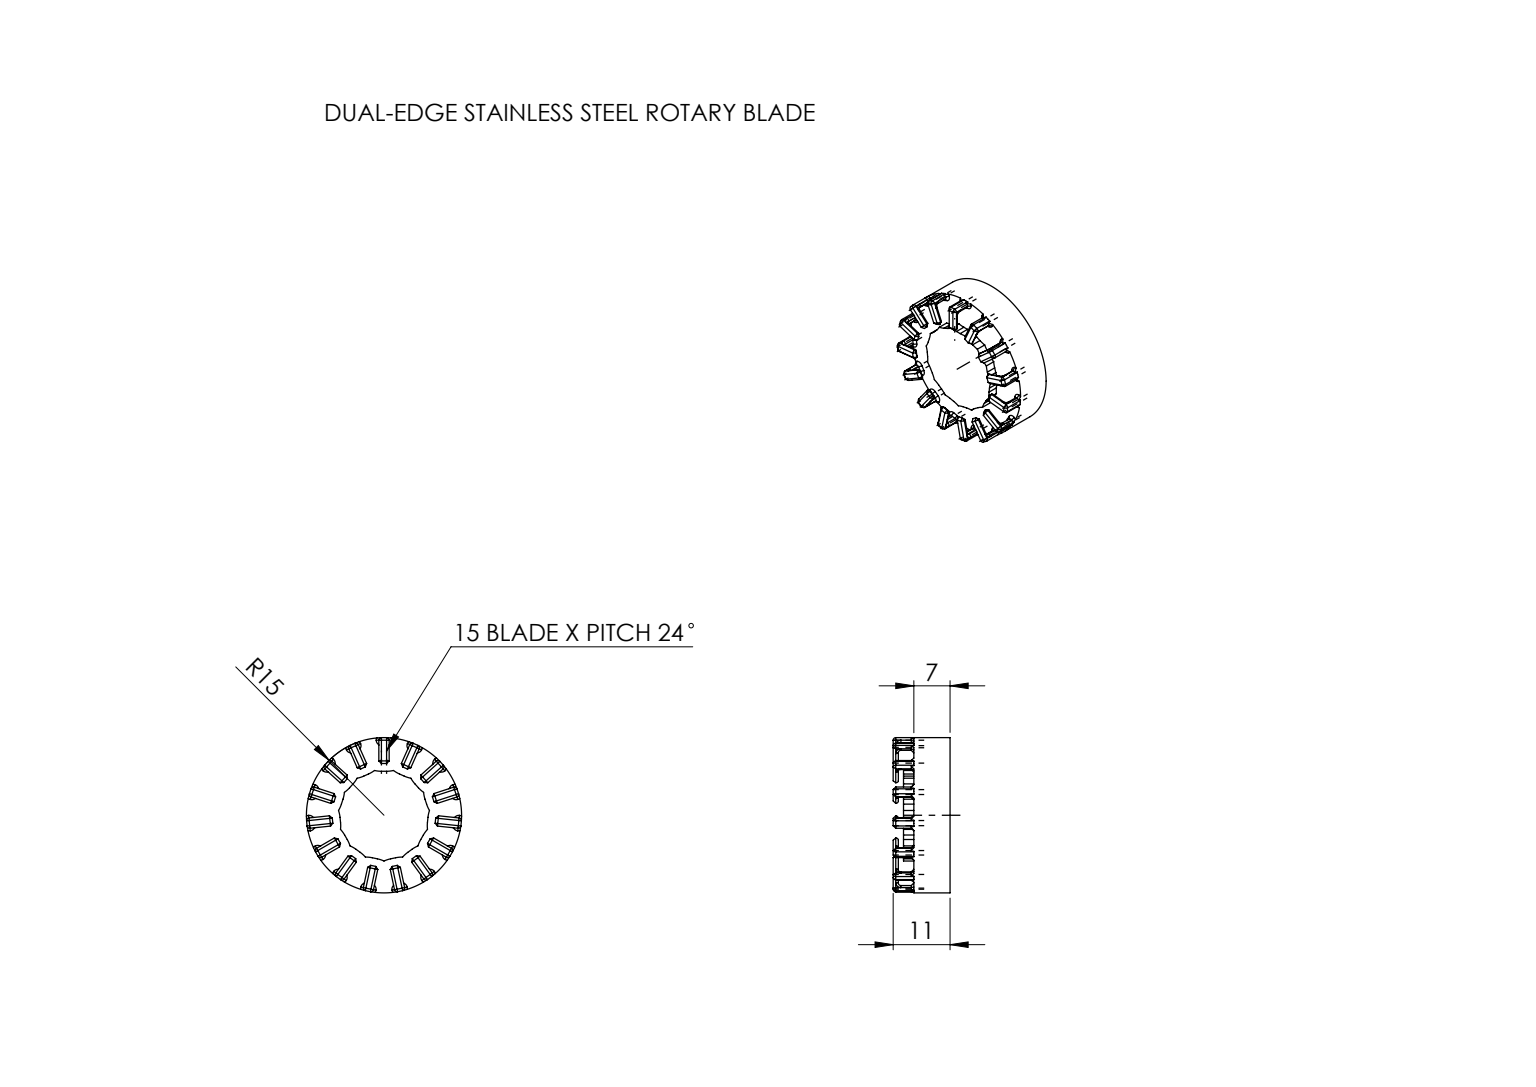
ISO-10303-21;
HEADER;
FILE_DESCRIPTION (('STEP AP214'),
    '1' );
FILE_NAME ('Dual-Edge Stainless Steel Rotary Blade.step',
    '2026-10-04T08:29:30',
    ( '' ),
    ( '' ),
    'SwSTEP 2.0',
    'SolidWorks 2026',
    '' );
FILE_SCHEMA (( 'AUTOMOTIVE_DESIGN' ));
ENDSEC;

DATA;
#1=DIRECTION ( 'NONE',  ( 1.000000000000000000, 0.000000000000000000, 0.000000000000000000 ) ) ;
#2=ORIENTED_EDGE ( 'NONE', *, *, #18761, .T. ) ;
#6=DIRECTION ( 'NONE',  ( 1.000000000000000000, 0.000000000000000000, 0.000000000000000000 ) ) ;
#11=ORIENTED_EDGE ( 'NONE', *, *, #12384, .T. ) ;
#13=DIRECTION ( 'NONE',  ( -0.2185080122244334455, 0.6724985119639524944, -0.7071067811865451302 ) ) ;
#14=ORIENTED_EDGE ( 'NONE', *, *, #11344, .T. ) ;
#16=ORIENTED_EDGE ( 'NONE', *, *, #14456, .T. ) ;
#21=CARTESIAN_POINT ( 'NONE',  ( -7.470035553104361625, 44.81454624109330354, 7.499999999999994671 ) ) ;
#23=DIRECTION ( 'NONE',  ( 0.8660254037844363761, -0.5000000000000038858, 0.000000000000000000 ) ) ;
#24=CARTESIAN_POINT ( 'NONE',  ( 0.000000000000000000, 22.50000000000000355, 7.000000000000000000 ) ) ;
#25=DIRECTION ( 'NONE',  ( 0.9510565162951544194, 0.3090169943749449533, -0.000000000000000000 ) ) ;
#26=AXIS2_PLACEMENT_3D ( 'NONE', #30413, #27350, #24305 ) ;
#29=CARTESIAN_POINT ( 'NONE',  ( 11.44473057578109199, 31.45924896672603310, 11.00000000000000000 ) ) ;
#32=PLANE ( 'NONE',  #24163 ) ;
#36=AXIS2_PLACEMENT_3D ( 'NONE', #271, #15908, #35000 ) ;
#42=VERTEX_POINT ( 'NONE', #38948 ) ;
#46=EDGE_LOOP ( 'NONE', ( #16862, #39215, #35738, #30448, #9840 ) ) ;
#50=DIRECTION ( 'NONE',  ( 0.000000000000000000, 0.000000000000000000, 1.000000000000000000 ) ) ;
#51=ORIENTED_EDGE ( 'NONE', *, *, #33215, .T. ) ;
#53=DIRECTION ( 'NONE',  ( 0.000000000000000000, 0.000000000000000000, 1.000000000000000000 ) ) ;
#55=VECTOR ( 'NONE', #14215, 1000.000000000000114 ) ;
#56=ORIENTED_EDGE ( 'NONE', *, *, #7043, .F. ) ;
#58=EDGE_LOOP ( 'NONE', ( #5255, #36161, #10685, #33701, #20952, #26926 ) ) ;
#62=ADVANCED_FACE ( 'NONE', ( #11719 ), #11120, .F. ) ;
#65=B_SPLINE_CURVE_WITH_KNOTS ( 'NONE', 3,
 ( #33912, #15414, #12759, #24753 ),
 .UNSPECIFIED., .F., .F.,
 ( 4, 4 ),
 ( 0.000000000000000000, 1.000000000000000000 ),
 .UNSPECIFIED. ) ;
#66=DIRECTION ( 'NONE',  ( -0.7431448254773862505, 0.6691306063588670083, 0.000000000000000000 ) ) ;
#68=AXIS2_PLACEMENT_3D ( 'NONE', #9965, #18910, #3865 ) ;
#69=CARTESIAN_POINT ( 'NONE',  ( 13.16028273094469192, 27.30176617939681449, 7.500000000000000000 ) ) ;
#71=AXIS2_PLACEMENT_3D ( 'NONE', #37438, #19346, #24844 ) ;
#72=DIRECTION ( 'NONE',  ( 1.000000000000000000, 0.000000000000000000, 0.000000000000000000 ) ) ;
#77=LINE ( 'NONE', #28854, #39100 ) ;
#80=AXIS2_PLACEMENT_3D ( 'NONE', #8723, #5868, #21115 ) ;
#86=EDGE_CURVE ( 'NONE', #10650, #36352, #5018, .T. ) ;
#87=EDGE_CURVE ( 'NONE', #32024, #8691, #8265, .T. ) ;
#88=FACE_OUTER_BOUND ( 'NONE', #25891, .T. ) ;
#92=EDGE_LOOP ( 'NONE', ( #13644, #34417, #27683, #7485 ) ) ;
#96=CARTESIAN_POINT ( 'NONE',  ( -10.06946225350398194, 32.23940090176283491, 9.500000000000000000 ) ) ;
#97=VECTOR ( 'NONE', #32100, 1000.000000000000000 ) ;
#101=CARTESIAN_POINT ( 'NONE',  ( -14.97283176289963968, 21.60377111278828011, 10.49999999999999645 ) ) ;
#103=ORIENTED_EDGE ( 'NONE', *, *, #28678, .T. ) ;
#106=LINE ( 'NONE', #9845, #39374 ) ;
#108=ORIENTED_EDGE ( 'NONE', *, *, #38694, .T. ) ;
#111=DIRECTION ( 'NONE',  ( 0.000000000000000000, 0.000000000000000000, 1.000000000000000000 ) ) ;
#113=VERTEX_POINT ( 'NONE', #23905 ) ;
#114=VECTOR ( 'NONE', #22519, 1000.000000000000000 ) ;
#117=DIRECTION ( 'NONE',  ( 0.1045284632676436315, -0.9945218953682742891, 0.000000000000000000 ) ) ;
#118=ORIENTED_EDGE ( 'NONE', *, *, #842, .F. ) ;
#119=CARTESIAN_POINT ( 'NONE',  ( 14.09933648065468503, 26.02968990214154843, 7.500000000000000888 ) ) ;
#121=DIRECTION ( 'NONE',  ( 0.5446390350150238646, -0.8386705679454261597, 0.000000000000000000 ) ) ;
#124=DIRECTION ( 'NONE',  ( 1.000000000000000000, 3.469446951953568829E-15, 0.000000000000000000 ) ) ;
#125=FACE_OUTER_BOUND ( 'NONE', #14098, .T. ) ;
#126=LINE ( 'NONE', #12516, #37440 ) ;
#127=CARTESIAN_POINT ( 'NONE',  ( 11.77212950435618488, 31.79629403205455063, 7.338691926023207301 ) ) ;
#129=CYLINDRICAL_SURFACE ( 'NONE', #3554, 0.5000000000000004441 ) ;
#130=ORIENTED_EDGE ( 'NONE', *, *, #22039, .F. ) ;
#132=FACE_OUTER_BOUND ( 'NONE', #27069, .T. ) ;
#134=AXIS2_PLACEMENT_3D ( 'NONE', #36095, #30198, #27342 ) ;
#136=ADVANCED_FACE ( 'NONE', ( #30004 ), #2180, .T. ) ;
#139=B_SPLINE_CURVE_WITH_KNOTS ( 'NONE', 3,
 ( #14310, #17577, #20620, #36259, #23258, #23855, #38896, #35449 ),
 .UNSPECIFIED., .F., .F.,
 ( 4, 2, 2, 4 ),
 ( 0.000000000000000000, 0.0004726692273637091287, 0.0007090038410455639642, 0.0009453384547274186912 ),
 .UNSPECIFIED. ) ;
#141=ORIENTED_EDGE ( 'NONE', *, *, #26869, .T. ) ;
#142=FACE_OUTER_BOUND ( 'NONE', #24319, .T. ) ;
#150=CARTESIAN_POINT ( 'NONE',  ( -8.927394655428429360, 11.06314620770957013, 11.00000000000000000 ) ) ;
#151=ORIENTED_EDGE ( 'NONE', *, *, #23785, .T. ) ;
#155=ORIENTED_EDGE ( 'NONE', *, *, #21487, .F. ) ;
#156=CYLINDRICAL_SURFACE ( 'NONE', #5742, 0.5000000000000004441 ) ;
#157=DIRECTION ( 'NONE',  ( -0.1045284632676566766, -0.9945218953682730678, 0.000000000000000000 ) ) ;
#159=EDGE_CURVE ( 'NONE', #19442, #37263, #30806, .T. ) ;
#162=EDGE_CURVE ( 'NONE', #21531, #36577, #11917, .T. ) ;
#163=VERTEX_POINT ( 'NONE', #30609 ) ;
#165=CARTESIAN_POINT ( 'NONE',  ( 6.654030453887980201, 35.94335816374507431, 7.500000000000000888 ) ) ;
#166=ORIENTED_EDGE ( 'NONE', *, *, #36174, .F. ) ;
#167=DIRECTION ( 'NONE',  ( -1.000000000000000000, 0.000000000000000000, 0.000000000000000000 ) ) ;
#170=VECTOR ( 'NONE', #21979, 1000.000000000000000 ) ;
#171=CARTESIAN_POINT ( 'NONE',  ( 0.000000000000000000, 22.50000000000000355, 7.000000000000000000 ) ) ;
#172=VERTEX_POINT ( 'NONE', #15755 ) ;
#174=DIRECTION ( 'NONE',  ( 0.000000000000000000, 0.000000000000000000, -1.000000000000000000 ) ) ;
#177=DIRECTION ( 'NONE',  ( 0.000000000000000000, 0.000000000000000000, -1.000000000000000000 ) ) ;
#178=CARTESIAN_POINT ( 'NONE',  ( 14.47283171447379146, 21.48159823030311344, 7.500000000000010658 ) ) ;
#180=ORIENTED_EDGE ( 'NONE', *, *, #19438, .T. ) ;
#184=LINE ( 'NONE', #27415, #10010 ) ;
#188=LINE ( 'NONE', #25168, #20681 ) ;
#189=EDGE_CURVE ( 'NONE', #7975, #16887, #8966, .T. ) ;
#190=AXIS2_PLACEMENT_3D ( 'NONE', #26813, #7919, #22957 ) ;
#197=CARTESIAN_POINT ( 'NONE',  ( -9.677076426724102731, 26.69573495723219736, 10.50000000000000000 ) ) ;
#198=ORIENTED_EDGE ( 'NONE', *, *, #35032, .T. ) ;
#201=CARTESIAN_POINT ( 'NONE',  ( -8.306370210276497801, 9.993911548625852959, 10.49999999999999822 ) ) ;
#202=LINE ( 'NONE', #23984, #35140 ) ;
#203=ORIENTED_EDGE ( 'NONE', *, *, #26918, .F. ) ;
#207=ORIENTED_EDGE ( 'NONE', *, *, #30268, .T. ) ;
#209=DIRECTION ( 'NONE',  ( 0.6123724356958052395, 0.3535533905932595200, -0.7071067811865454633 ) ) ;
#210=EDGE_CURVE ( 'NONE', #22927, #29202, #39935, .T. ) ;
#211=VECTOR ( 'NONE', #28552, 1000.000000000000000 ) ;
#215=EDGE_CURVE ( 'NONE', #19575, #30083, #1517, .T. ) ;
#216=EDGE_LOOP ( 'NONE', ( #4536, #16133, #31309, #14302 ) ) ;
#218=PLANE ( 'NONE',  #11258 ) ;
#219=AXIS2_PLACEMENT_3D ( 'NONE', #21595, #14504, #26896 ) ;
#220=CARTESIAN_POINT ( 'NONE',  ( 2.629601561899395534, 7.723830143584016206, 10.49999999999999822 ) ) ;
#222=STYLED_ITEM ( 'NONE', ( #29995 ), #8155 ) ;
#224=CARTESIAN_POINT ( 'NONE',  ( 5.288651019504051476, 36.01756689786824239, 10.83333333333333393 ) ) ;
#225=ORIENTED_EDGE ( 'NONE', *, *, #29984, .F. ) ;
#226=FACE_OUTER_BOUND ( 'NONE', #33759, .T. ) ;
#229=FACE_OUTER_BOUND ( 'NONE', #25110, .T. ) ;
#232=AXIS2_PLACEMENT_3D ( 'NONE', #21106, #26799, #8514 ) ;
#234=DIRECTION ( 'NONE',  ( -0.000000000000000000, -0.000000000000000000, -1.000000000000000000 ) ) ;
#236=EDGE_CURVE ( 'NONE', #29069, #1872, #12116, .T. ) ;
#239=CIRCLE ( 'NONE', #18429, 0.5000000000000004441 ) ;
#248=CIRCLE ( 'NONE', #15817, 0.5000000000000004441 ) ;
#249=ORIENTED_EDGE ( 'NONE', *, *, #12112, .F. ) ;
#252=DIRECTION ( 'NONE',  ( 0.9781476007338072431, 0.2079116908177519041, 0.000000000000000000 ) ) ;
#253=VERTEX_POINT ( 'NONE', #30414 ) ;
#257=VERTEX_POINT ( 'NONE', #18219 ) ;
#259=ORIENTED_EDGE ( 'NONE', *, *, #8002, .F. ) ;
#265=ORIENTED_EDGE ( 'NONE', *, *, #11360, .F. ) ;
#267=DIRECTION ( 'NONE',  ( 0.7431448254773953543, 0.6691306063588571273, 0.000000000000000000 ) ) ;
#271=CARTESIAN_POINT ( 'NONE',  ( -8.118377661053489902, 10.47536095541709322, 9.000000000000001776 ) ) ;
#272=PRODUCT_DEFINITION_SHAPE ( 'NONE', 'NONE',  #1580 ) ;
#277=CARTESIAN_POINT ( 'NONE',  ( 8.137585970692082782, 29.15429895402929361, 11.00000000000000000 ) ) ;
#280=CARTESIAN_POINT ( 'NONE',  ( -9.356056665764020508, 26.06569820189716324, 10.50000000000000533 ) ) ;
#283=AXIS2_PLACEMENT_3D ( 'NONE', #15158, #26953, #5218 ) ;
#287=LINE ( 'NONE', #25064, #8816 ) ;
#289=EDGE_LOOP ( 'NONE', ( #19488, #26739, #33941, #35393 ) ) ;
#290=EDGE_CURVE ( 'NONE', #7488, #10226, #26444, .T. ) ;
#291=DIRECTION ( 'NONE',  ( 0.9781476007338042455, -0.2079116908177663647, 0.000000000000000000 ) ) ;
#294=LINE ( 'NONE', #21426, #16002 ) ;
#297=ORIENTED_EDGE ( 'NONE', *, *, #12319, .F. ) ;
#300=PLANE ( 'NONE',  #32607 ) ;
#302=ORIENTED_EDGE ( 'NONE', *, *, #4167, .F. ) ;
#306=EDGE_CURVE ( 'NONE', #11401, #17187, #24700, .T. ) ;
#307=DIRECTION ( 'NONE',  ( 0.000000000000000000, 0.000000000000000000, -1.000000000000000000 ) ) ;
#310=VECTOR ( 'NONE', #30674, 1000.000000000000114 ) ;
#316=LINE ( 'NONE', #21645, #40068 ) ;
#320=CARTESIAN_POINT ( 'NONE',  ( -13.48130249190472796, 27.93180293473203690, 10.50000000000000533 ) ) ;
#324=DIRECTION ( 'NONE',  ( -0.000000000000000000, -0.000000000000000000, -1.000000000000000000 ) ) ;
#326=DIRECTION ( 'NONE',  ( -0.2079116908177664480, -0.9781476007338042455, 0.000000000000000000 ) ) ;
#328=CARTESIAN_POINT ( 'NONE',  ( 12.80736835487433289, 15.68301270189216545, 9.000000000000001776 ) ) ;
#332=DIRECTION ( 'NONE',  ( -0.2079116908177667256, -0.9781476007338041345, 1.734723475976808475E-15 ) ) ;
#335=CARTESIAN_POINT ( 'NONE',  ( 8.593266739736579396, 16.38397459621552699, 11.00000000000000000 ) ) ;
#336=DIRECTION ( 'NONE',  ( -0.000000000000000000, -0.000000000000000000, 1.000000000000000000 ) ) ;
#343=VECTOR ( 'NONE', #22858, 1000.000000000000000 ) ;
#347=VECTOR ( 'NONE', #26561, 1000.000000000000000 ) ;
#352=EDGE_CURVE ( 'NONE', #2306, #34064, #29151, .T. ) ;
#354=CARTESIAN_POINT ( 'NONE',  ( -10.44103466624267185, 32.57396620494226624, 7.000000000000000000 ) ) ;
#359=ORIENTED_EDGE ( 'NONE', *, *, #3116, .F. ) ;
#360=LINE ( 'NONE', #21297, #8908 ) ;
#361=DIRECTION ( 'NONE',  ( -0.9781476007338043566, 0.2079116908177657264, 0.000000000000000000 ) ) ;
#365=B_SPLINE_CURVE_WITH_KNOTS ( 'NONE', 3,
 ( #13662, #35008, #16115, #477 ),
 .UNSPECIFIED., .F., .F.,
 ( 4, 4 ),
 ( 0.0008976806579034594512, 0.0009453384547274206427 ),
 .UNSPECIFIED. ) ;
#366=EDGE_LOOP ( 'NONE', ( #29228, #30799, #2804, #38071 ) ) ;
#367=EDGE_CURVE ( 'NONE', #32326, #14728, #6690, .T. ) ;
#368=DIRECTION ( 'NONE',  ( -0.000000000000000000, -0.000000000000000000, 1.000000000000000000 ) ) ;
#371=DIRECTION ( 'NONE',  ( 0.4156269377774552409, 0.5720614028176769228, 0.7071067811865524577 ) ) ;
#374=AXIS2_PLACEMENT_3D ( 'NONE', #5565, #29757, #14717 ) ;
#375=AXIS2_PLACEMENT_3D ( 'NONE', #24776, #21926, #21529 ) ;
#377=EDGE_LOOP ( 'NONE', ( #16222, #29568, #22970, #4101 ) ) ;
#379=CARTESIAN_POINT ( 'NONE',  ( -9.337241587065845394, 10.76617146908760247, 10.49999999999999822 ) ) ;
#380=CARTESIAN_POINT ( 'NONE',  ( -9.625795778762141097, 10.95253033666833709, 10.50000000000000533 ) ) ;
#381=DIRECTION ( 'NONE',  ( -0.000000000000000000, -0.000000000000000000, -1.000000000000000000 ) ) ;
#383=DIRECTION ( 'NONE',  ( 0.000000000000000000, 0.000000000000000000, 1.000000000000000000 ) ) ;
#385=EDGE_LOOP ( 'NONE', ( #29056, #12887, #37064, #5355 ) ) ;
#392=ADVANCED_FACE ( 'NONE', ( #10459 ), #7403, .F. ) ;
#393=FACE_OUTER_BOUND ( 'NONE', #10195, .T. ) ;
#398=CARTESIAN_POINT ( 'NONE',  ( 14.08246327825360389, 27.69965426814068366, 10.49999999999999822 ) ) ;
#400=VERTEX_POINT ( 'NONE', #31792 ) ;
#402=AXIS2_PLACEMENT_3D ( 'NONE', #36373, #21524, #8537 ) ;
#408=ORIENTED_EDGE ( 'NONE', *, *, #8409, .F. ) ;
#410=CARTESIAN_POINT ( 'NONE',  ( -13.13581098909220302, 27.45627467658446008, 11.00000000000000000 ) ) ;
#413=ORIENTED_EDGE ( 'NONE', *, *, #8934, .F. ) ;
#416=ORIENTED_EDGE ( 'NONE', *, *, #27931, .F. ) ;
#425=ORIENTED_EDGE ( 'NONE', *, *, #25457, .F. ) ;
#429=DIRECTION ( 'NONE',  ( -0.8090169943749504489, -0.5877852522924690293, 0.000000000000000000 ) ) ;
#437=EDGE_CURVE ( 'NONE', #21611, #37532, #717, .T. ) ;
#438=ORIENTED_EDGE ( 'NONE', *, *, #8735, .T. ) ;
#442=EDGE_CURVE ( 'NONE', #4338, #959, #22639, .T. ) ;
#444=EDGE_LOOP ( 'NONE', ( #34440, #26778, #20838, #31828 ) ) ;
#445=VERTEX_POINT ( 'NONE', #22048 ) ;
#449=ORIENTED_EDGE ( 'NONE', *, *, #1153, .F. ) ;
#450=EDGE_CURVE ( 'NONE', #13434, #36251, #32021, .T. ) ;
#454=ORIENTED_EDGE ( 'NONE', *, *, #7492, .F. ) ;
#456=LINE ( 'NONE', #12243, #18704 ) ;
#457=DIRECTION ( 'NONE',  ( 0.000000000000000000, 0.000000000000000000, 1.000000000000000000 ) ) ;
#458=EDGE_LOOP ( 'NONE', ( #11462, #15497, #1605 ) ) ;
#462=AXIS2_PLACEMENT_3D ( 'NONE', #19631, #7640, #26540 ) ;
#465=ORIENTED_EDGE ( 'NONE', *, *, #21335, .F. ) ;
#467=CARTESIAN_POINT ( 'NONE',  ( -14.63635198741550347, 25.78286467897752487, 7.000000000000000000 ) ) ;
#470=VECTOR ( 'NONE', #7205, 1000.000000000000000 ) ;
#471=LINE ( 'NONE', #3906, #36294 ) ;
#474=DIRECTION ( 'NONE',  ( 1.000000000000000000, 0.000000000000000000, 0.000000000000000000 ) ) ;
#477=CARTESIAN_POINT ( 'NONE',  ( -14.44277748876676881, 26.55045409923033972, 7.499999999999993783 ) ) ;
#480=VECTOR ( 'NONE', #651, 1000.000000000000114 ) ;
#481=VERTEX_POINT ( 'NONE', #34449 ) ;
#483=AXIS2_PLACEMENT_3D ( 'NONE', #20290, #35930, #32279 ) ;
#486=CARTESIAN_POINT ( 'NONE',  ( 10.51560177358059534, 33.07492339674065818, 10.49999999999999822 ) ) ;
#490=VERTEX_POINT ( 'NONE', #28941 ) ;
#491=VECTOR ( 'NONE', #25478, 1000.000000000000000 ) ;
#493=DIRECTION ( 'NONE',  ( 0.7431448254773954654, 0.6691306063588569053, -0.000000000000000000 ) ) ;
#504=CARTESIAN_POINT ( 'NONE',  ( -3.597409820281606940, 14.42008525284352594, 9.000000000000001776 ) ) ;
#505=DIRECTION ( 'NONE',  ( -0.5877852522924796874, -0.8090169943749425663, 0.000000000000000000 ) ) ;
#506=CARTESIAN_POINT ( 'NONE',  ( -9.221287281574667816, 10.65863771052209863, 7.000000000000000000 ) ) ;
#511=ORIENTED_EDGE ( 'NONE', *, *, #1102, .F. ) ;
#512=VECTOR ( 'NONE', #22352, 1000.000000000000000 ) ;
#514=CARTESIAN_POINT ( 'NONE',  ( 14.36830325120613594, 20.48707633493483371, 9.000000000000001776 ) ) ;
#515=AXIS2_PLACEMENT_3D ( 'NONE', #19842, #29379, #10491 ) ;
#517=ADVANCED_FACE ( 'NONE', ( #1121 ), #13502, .T. ) ;
#518=CARTESIAN_POINT ( 'NONE',  ( 14.52509594610761923, 21.97885917798724975, 7.500000000000010658 ) ) ;
#519=VECTOR ( 'NONE', #30356, 999.9999999999998863 ) ;
#520=CARTESIAN_POINT ( 'NONE',  ( -11.61146752755215417, 31.78078372435996002, 10.49999999999999822 ) ) ;
#521=DIRECTION ( 'NONE',  ( -0.000000000000000000, -0.000000000000000000, -1.000000000000000000 ) ) ;
#523=LINE ( 'NONE', #12905, #3587 ) ;
#524=CARTESIAN_POINT ( 'NONE',  ( 14.55889214498799689, 20.02072497456981282, 10.49999999999999822 ) ) ;
#526=CARTESIAN_POINT ( 'NONE',  ( -14.81329996725647469, 19.93755115561707569, 11.00000000000000000 ) ) ;
#527=CARTESIAN_POINT ( 'NONE',  ( -14.25384497784211923, 25.55416164399415280, 7.000000000000000000 ) ) ;
#530=DIRECTION ( 'NONE',  ( 0.000000000000000000, 0.000000000000000000, -1.000000000000000000 ) ) ;
#531=ORIENTED_EDGE ( 'NONE', *, *, #18718, .T. ) ;
#533=CARTESIAN_POINT ( 'NONE',  ( 2.046188276595768407, 8.063706679521116527, 10.49999999999999822 ) ) ;
#540=DIRECTION ( 'NONE',  ( -0.000000000000000000, -0.000000000000000000, -1.000000000000000000 ) ) ;
#543=AXIS2_PLACEMENT_3D ( 'NONE', #36741, #6444, #8906 ) ;
#544=TOROIDAL_SURFACE ( 'NONE', #21940, 1.000000000000000000, 0.5000000000000000000 ) ;
#550=CARTESIAN_POINT ( 'NONE',  ( 5.767236651883445475, 13.71142893291679243, 10.50000000000000000 ) ) ;
#552=AXIS2_PLACEMENT_3D ( 'NONE', #26299, #39088, #32608 ) ;
#559=CARTESIAN_POINT ( 'NONE',  ( 14.81329996725643738, 19.93755115561686964, 11.00000000000000000 ) ) ;
#563=ADVANCED_FACE ( 'NONE', ( #26303 ), #20819, .T. ) ;
#568=AXIS2_PLACEMENT_3D ( 'NONE', #19540, #31929, #16503 ) ;
#570=ORIENTED_EDGE ( 'NONE', *, *, #16751, .F. ) ;
#571=EDGE_CURVE ( 'NONE', #36570, #10398, #25541, .T. ) ;
#574=CARTESIAN_POINT ( 'NONE',  ( -15.00000000000000000, 22.50000000000000355, 0.000000000000000000 ) ) ;
#576=AXIS2_PLACEMENT_3D ( 'NONE', #4517, #7758, #23405 ) ;
#578=CARTESIAN_POINT ( 'NONE',  ( 7.282669157963869822, 29.73016112791698262, 10.75000000000000000 ) ) ;
#585=PLANE ( 'NONE',  #20443 ) ;
#588=PLANE ( 'NONE',  #3155 ) ;
#593=EDGE_CURVE ( 'NONE', #38427, #25178, #1550, .T. ) ;
#594=CARTESIAN_POINT ( 'NONE',  ( 13.72389693702425184, 27.48489553602867019, 10.99387789255783687 ) ) ;
#595=DIRECTION ( 'NONE',  ( -0.000000000000000000, -0.000000000000000000, 1.000000000000000000 ) ) ;
#596=ADVANCED_FACE ( 'NONE', ( #10870 ), #32410, .F. ) ;
#597=ORIENTED_EDGE ( 'NONE', *, *, #23075, .F. ) ;
#599=CARTESIAN_POINT ( 'NONE',  ( 2.256323172317815207, 14.28970123917151192, 9.000000000000001776 ) ) ;
#602=FACE_OUTER_BOUND ( 'NONE', #27008, .T. ) ;
#603=EDGE_LOOP ( 'NONE', ( #23347, #6480, #32826, #34211 ) ) ;
#606=FACE_OUTER_BOUND ( 'NONE', #33987, .T. ) ;
#608=B_SPLINE_SURFACE_WITH_KNOTS ( 'NONE', 1, 3, ( 
 ( #8281, #20688, #33083, #17647, #29414, #30019, #1791, #10525, #2195, #7469 ),
 ( #32265, #16834, #29215, #30431, #11932, #11734, #27366, #2393, #27566, #11535 ) ),
 .UNSPECIFIED., .F., .F., .F.,
 ( 2, 2 ),
 ( 4, 2, 2, 2, 4 ),
 ( 0.000000000000000000, 1.000000000000000000 ),
 ( -1.344962617103292679, -0.9522635354045664302, -0.5595644537058401813, -0.1668653720071138769, 0.2258337096916124276 ),
 .UNSPECIFIED. ) ;
#611=DIRECTION ( 'NONE',  ( 0.000000000000000000, -0.000000000000000000, -1.000000000000000000 ) ) ;
#612=ORIENTED_EDGE ( 'NONE', *, *, #30344, .T. ) ;
#614=VERTEX_POINT ( 'NONE', #20214 ) ;
#616=CARTESIAN_POINT ( 'NONE',  ( -13.94482798346716201, 26.50521816028930999, 7.000000000000000000 ) ) ;
#617=CARTESIAN_POINT ( 'NONE',  ( 5.947717410344609767, 34.62949535663720013, 7.000000000000000000 ) ) ;
#621=EDGE_LOOP ( 'NONE', ( #17162, #4935, #36145, #2379, #27346, #12203, #28190 ) ) ;
#628=AXIS2_PLACEMENT_3D ( 'NONE', #36059, #24064, #26910 ) ;
#629=ORIENTED_EDGE ( 'NONE', *, *, #20742, .F. ) ;
#631=DIRECTION ( 'NONE',  ( 0.000000000000000000, 0.000000000000000000, -1.000000000000000000 ) ) ;
#643=DIRECTION ( 'NONE',  ( 0.3090169943749573322, 0.9510565162951504226, -0.000000000000000000 ) ) ;
#647=FACE_OUTER_BOUND ( 'NONE', #36295, .T. ) ;
#651=DIRECTION ( 'NONE',  ( -0.3535533905932792820, -0.6123724356957955806, -0.7071067811865437980 ) ) ;
#652=ORIENTED_EDGE ( 'NONE', *, *, #37876, .T. ) ;
#654=ORIENTED_EDGE ( 'NONE', *, *, #20863, .T. ) ;
#656=AXIS2_PLACEMENT_3D ( 'NONE', #39004, #20734, #38601 ) ;
#659=VERTEX_POINT ( 'NONE', #11273 ) ;
#660=AXIS2_PLACEMENT_3D ( 'NONE', #1120, #13501, #15263 ) ;
#661=DIRECTION ( 'NONE',  ( -0.000000000000000000, -0.000000000000000000, -1.000000000000000000 ) ) ;
#662=EDGE_CURVE ( 'NONE', #39411, #25405, #239, .T. ) ;
#666=FACE_OUTER_BOUND ( 'NONE', #37210, .T. ) ;
#667=VECTOR ( 'NONE', #4209, 1000.000000000000000 ) ;
#669=LINE ( 'NONE', #26655, #35272 ) ;
#675=ORIENTED_EDGE ( 'NONE', *, *, #10855, .T. ) ;
#678=CARTESIAN_POINT ( 'NONE',  ( 10.50986403156584714, 32.63594044384544901, 10.99387789255782977 ) ) ;
#687=CARTESIAN_POINT ( 'NONE',  ( -14.73239529508891188, 21.45431699865994446, 10.94611345180490680 ) ) ;
#688=EDGE_CURVE ( 'NONE', #13732, #13187, #35450, .T. ) ;
#690=CARTESIAN_POINT ( 'NONE',  ( 12.69365875748871808, 14.48606190191208043, 10.49999999999999822 ) ) ;
#691=EDGE_CURVE ( 'NONE', #38413, #8131, #33021, .T. ) ;
#700=CARTESIAN_POINT ( 'NONE',  ( -13.30736791469135483, 15.68301270237671474, 10.49999999999999822 ) ) ;
#701=CARTESIAN_POINT ( 'NONE',  ( -10.26940745284057321, 33.04623494220486890, 10.49999999999999822 ) ) ;
#702=ORIENTED_EDGE ( 'NONE', *, *, #1930, .F. ) ;
#705=AXIS2_PLACEMENT_3D ( 'NONE', #15865, #25, #24803 ) ;
#707=AXIS2_PLACEMENT_3D ( 'NONE', #29205, #32465, #35505 ) ;
#710=EDGE_CURVE ( 'NONE', #32625, #13649, #10400, .T. ) ;
#712=EDGE_CURVE ( 'NONE', #7720, #4426, #23259, .T. ) ;
#713=ORIENTED_EDGE ( 'NONE', *, *, #38236, .T. ) ;
#714=AXIS2_PLACEMENT_3D ( 'NONE', #38345, #10515, #35300 ) ;
#715=DIRECTION ( 'NONE',  ( -0.6691306063588706721, -0.7431448254773830309, -6.938893903907237844E-15 ) ) ;
#716=CARTESIAN_POINT ( 'NONE',  ( -11.48173768534022976, 32.16538668264431777, 10.49999999999999645 ) ) ;
#717=LINE ( 'NONE', #3561, #16478 ) ;
#721=CARTESIAN_POINT ( 'NONE',  ( -6.431109915229962226, 35.71521269883987770, 10.96580508970282253 ) ) ;
#722=DIRECTION ( 'NONE',  ( -0.1045284632676566766, -0.9945218953682730678, 0.000000000000000000 ) ) ;
#724=LINE ( 'NONE', #28551, #470 ) ;
#725=DIRECTION ( 'NONE',  ( 1.000000000000000000, 1.224646799147351235E-16, -0.000000000000000000 ) ) ;
#728=DIRECTION ( 'NONE',  ( 1.000000000000000000, 0.000000000000000000, 0.000000000000000000 ) ) ;
#733=CARTESIAN_POINT ( 'NONE',  ( 13.28731253932047807, 15.83618351361437959, 10.49999999999999822 ) ) ;
#734=CIRCLE ( 'NONE', #27335, 0.5000000000000007772 ) ;
#736=DIRECTION ( 'NONE',  ( 1.000000000000000000, 0.000000000000000000, 0.000000000000000000 ) ) ;
#738=ORIENTED_EDGE ( 'NONE', *, *, #6248, .T. ) ;
#740=ORIENTED_EDGE ( 'NONE', *, *, #36204, .T. ) ;
#741=CARTESIAN_POINT ( 'NONE',  ( 0.5000000000000005551, 32.50000000000000000, 10.49999999999999645 ) ) ;
#747=VERTEX_POINT ( 'NONE', #23050 ) ;
#749=CARTESIAN_POINT ( 'NONE',  ( -8.843266739736657556, 16.81698729810786830, 10.50000000000000000 ) ) ;
#751=VERTEX_POINT ( 'NONE', #4970 ) ;
#754=ORIENTED_EDGE ( 'NONE', *, *, #2123, .T. ) ;
#760=CIRCLE ( 'NONE', #6572, 1.000000000000007772 ) ;
#762=ORIENTED_EDGE ( 'NONE', *, *, #20179, .T. ) ;
#763=DIRECTION ( 'NONE',  ( -1.224646799147353947E-16, 1.000000000000000000, 0.000000000000000000 ) ) ;
#764=LINE ( 'NONE', #29397, #38958 ) ;
#765=CARTESIAN_POINT ( 'NONE',  ( 5.440908595777819379, 35.94977745735560859, 11.00000000000000000 ) ) ;
#766=ORIENTED_EDGE ( 'NONE', *, *, #9500, .T. ) ;
#768=CARTESIAN_POINT ( 'NONE',  ( -14.06524961900331760, 27.71236540882611621, 7.499999999999993783 ) ) ;
#769=CARTESIAN_POINT ( 'NONE',  ( -10.54700836463453584, 22.39697303105802462, 11.00000000000000000 ) ) ;
#770=AXIS2_PLACEMENT_3D ( 'NONE', #10146, #34727, #6484 ) ;
#771=FACE_OUTER_BOUND ( 'NONE', #385, .T. ) ;
#772=DIRECTION ( 'NONE',  ( 1.000000000000000000, 0.000000000000000000, 0.000000000000000000 ) ) ;
#773=DIRECTION ( 'NONE',  ( -0.07391278520356947546, -0.7032331762534066444, -0.7071067811865447972 ) ) ;
#778=DIRECTION ( 'NONE',  ( -0.8660254037844432595, -0.4999999999999920064, 0.000000000000000000 ) ) ;
#779=CARTESIAN_POINT ( 'NONE',  ( 7.766013557953382218, 28.81973365084987293, 10.00000000000000000 ) ) ;
#781=CARTESIAN_POINT ( 'NONE',  ( -11.44473057578096764, 31.45924896672619298, 7.500000000000004441 ) ) ;
#789=EDGE_CURVE ( 'NONE', #38536, #6543, #27496, .T. ) ;
#790=CARTESIAN_POINT ( 'NONE',  ( 14.11133924723983490, 27.61078317377175395, 10.49999999999999112 ) ) ;
#791=CARTESIAN_POINT ( 'NONE',  ( -0.9999999999999997780, 36.00000000000000711, 10.50000000000000000 ) ) ;
#792=ORIENTED_EDGE ( 'NONE', *, *, #25775, .F. ) ;
#794=CARTESIAN_POINT ( 'NONE',  ( 14.47283171447379146, 21.48159823030311344, 11.00000000000000000 ) ) ;
#795=ORIENTED_EDGE ( 'NONE', *, *, #33606, .T. ) ;
#797=EDGE_CURVE ( 'NONE', #24743, #614, #12560, .T. ) ;
#798=CYLINDRICAL_SURFACE ( 'NONE', #21949, 0.4999999999999981681 ) ;
#799=AXIS2_PLACEMENT_3D ( 'NONE', #36695, #5807, #18404 ) ;
#800=CARTESIAN_POINT ( 'NONE',  ( -10.33795143809923545, 20.40792924032147226, 10.49999999999999467 ) ) ;
#802=VERTEX_POINT ( 'NONE', #27695 ) ;
#805=ORIENTED_EDGE ( 'NONE', *, *, #87, .F. ) ;
#807=AXIS2_PLACEMENT_3D ( 'NONE', #26934, #39521, #39719 ) ;
#809=ORIENTED_EDGE ( 'NONE', *, *, #16122, .T. ) ;
#813=LINE ( 'NONE', #34149, #15004 ) ;
#815=DIRECTION ( 'NONE',  ( 0.000000000000000000, 0.000000000000000000, -1.000000000000000000 ) ) ;
#816=ORIENTED_EDGE ( 'NONE', *, *, #29193, .T. ) ;
#817=AXIS2_PLACEMENT_3D ( 'NONE', #2928, #34208, #30371 ) ;
#821=EDGE_CURVE ( 'NONE', #30083, #13640, #37873, .T. ) ;
#822=CARTESIAN_POINT ( 'NONE',  ( 12.05736835487432579, 14.38397459621550567, 10.49999999999999822 ) ) ;
#824=VECTOR ( 'NONE', #14516, 1000.000000000000114 ) ;
#830=CARTESIAN_POINT ( 'NONE',  ( 3.784364466546041417, 47.62563423532509432, 7.000000000000000000 ) ) ;
#836=CARTESIAN_POINT ( 'NONE',  ( 0.000000000000000000, 22.50000000000000355, 7.000000000000000000 ) ) ;
#842=EDGE_CURVE ( 'NONE', #17938, #4137, #39467, .T. ) ;
#846=DIRECTION ( 'NONE',  ( -0.4156269377774569063, -0.5720614028176815857, -0.7071067811865476838 ) ) ;
#847=EDGE_LOOP ( 'NONE', ( #36208, #23534, #21814, #12695 ) ) ;
#850=DIRECTION ( 'NONE',  ( 0.1045284632676569680, 0.9945218953682729568, -0.000000000000000000 ) ) ;
#852=EDGE_LOOP ( 'NONE', ( #11085, #1876, #20436, #35870 ) ) ;
#855=VERTEX_POINT ( 'NONE', #24451 ) ;
#863=FACE_OUTER_BOUND ( 'NONE', #16552, .T. ) ;
#865=AXIS2_PLACEMENT_3D ( 'NONE', #33227, #35660, #17588 ) ;
#866=DIRECTION ( 'NONE',  ( 0.9135454576426004225, -0.4067366430758009854, 0.000000000000000000 ) ) ;
#868=FACE_OUTER_BOUND ( 'NONE', #1524, .T. ) ;
#870=VECTOR ( 'NONE', #18177, 1000.000000000000114 ) ;
#876=DIRECTION ( 'NONE',  ( 0.000000000000000000, 0.000000000000000000, -1.000000000000000000 ) ) ;
#877=ORIENTED_EDGE ( 'NONE', *, *, #27021, .F. ) ;
#879=VECTOR ( 'NONE', #28401, 1000.000000000000000 ) ;
#892=EDGE_CURVE ( 'NONE', #1059, #25293, #22193, .T. ) ;
#895=ORIENTED_EDGE ( 'NONE', *, *, #15860, .F. ) ;
#898=CARTESIAN_POINT ( 'NONE',  ( 0.5000000000000000000, 37.00000000000000711, 7.000000000000000000 ) ) ;
#902=CARTESIAN_POINT ( 'NONE',  ( 13.30736791475921699, 15.68301270237638967, 10.49999999999999822 ) ) ;
#905=EDGE_CURVE ( 'NONE', #13411, #2697, #37018, .T. ) ;
#910=ORIENTED_EDGE ( 'NONE', *, *, #29653, .F. ) ;
#913=CARTESIAN_POINT ( 'NONE',  ( 5.400683141673458643, 15.91724817395916070, 9.000000000000001776 ) ) ;
#914=ORIENTED_EDGE ( 'NONE', *, *, #26901, .F. ) ;
#915=DIRECTION ( 'NONE',  ( -0.6691306063588671194, -0.7431448254773861395, -0.000000000000000000 ) ) ;
#916=EDGE_CURVE ( 'NONE', #33995, #4123, #669, .T. ) ;
#917=VECTOR ( 'NONE', #27944, 1000.000000000000114 ) ;
#920=CARTESIAN_POINT ( 'NONE',  ( -2.036571916123810055, 8.108948098542073879, 7.499999999999997335 ) ) ;
#923=DIRECTION ( 'NONE',  ( 1.000000000000000000, 0.000000000000000000, 0.000000000000000000 ) ) ;
#926=CARTESIAN_POINT ( 'NONE',  ( 14.44277748876681855, 26.55045409923015853, 7.000000000000000000 ) ) ;
#928=CARTESIAN_POINT ( 'NONE',  ( 13.19674782540804792, 16.00858767546125350, 10.49999999999999822 ) ) ;
#931=CARTESIAN_POINT ( 'NONE',  ( 8.927394655428274817, 11.06314620770945112, 9.500000000000000000 ) ) ;
#932=AXIS2_PLACEMENT_3D ( 'NONE', #35100, #7255, #38346 ) ;
#933=CARTESIAN_POINT ( 'NONE',  ( -13.36146265112639675, 15.68301270189280672, 7.445905703748357141 ) ) ;
#937=ORIENTED_EDGE ( 'NONE', *, *, #26202, .T. ) ;
#940=ORIENTED_EDGE ( 'NONE', *, *, #29925, .F. ) ;
#942=DIRECTION ( 'NONE',  ( 0.9510565162951504226, -0.3090169943749573322, 0.000000000000000000 ) ) ;
#944=EDGE_CURVE ( 'NONE', #35769, #14313, #38446, .T. ) ;
#949=ORIENTED_EDGE ( 'NONE', *, *, #13774, .F. ) ;
#950=EDGE_CURVE ( 'NONE', #4321, #28310, #29705, .T. ) ;
#954=ORIENTED_EDGE ( 'NONE', *, *, #24516, .T. ) ;
#957=EDGE_CURVE ( 'NONE', #26836, #32713, #21640, .T. ) ;
#959=VERTEX_POINT ( 'NONE', #13657 ) ;
#964=EDGE_LOOP ( 'NONE', ( #31219, #25857, #1045, #21630 ) ) ;
#965=ORIENTED_EDGE ( 'NONE', *, *, #34679, .F. ) ;
#966=DIRECTION ( 'NONE',  ( -0.5000000000000038858, -0.8660254037844364872, 0.000000000000000000 ) ) ;
#969=EDGE_CURVE ( 'NONE', #18974, #18778, #38852, .T. ) ;
#970=VECTOR ( 'NONE', #2003, 1000.000000000000114 ) ;
#971=CARTESIAN_POINT ( 'NONE',  ( -10.44103466624267185, 32.57396620494226624, 7.000000000000000000 ) ) ;
#975=FACE_OUTER_BOUND ( 'NONE', #36778, .T. ) ;
#979=FACE_OUTER_BOUND ( 'NONE', #25316, .T. ) ;
#981=DIRECTION ( 'NONE',  ( 0.8090169943749504489, 0.5877852522924689183, 0.000000000000000000 ) ) ;
#982=VECTOR ( 'NONE', #8472, 1000.000000000000000 ) ;
#985=LINE ( 'NONE', #10523, #15475 ) ;
#988=LINE ( 'NONE', #13370, #29539 ) ;
#992=EDGE_CURVE ( 'NONE', #16279, #36570, #31383, .T. ) ;
#996=EDGE_CURVE ( 'NONE', #36577, #34828, #35607, .T. ) ;
#1002=CIRCLE ( 'NONE', #26954, 0.5000000000000004441 ) ;
#1003=DIRECTION ( 'NONE',  ( -0.07391278520356937831, -0.7032331762534056452, 0.7071067811865457964 ) ) ;
#1006=DIRECTION ( 'NONE',  ( 1.000000000000000000, 0.000000000000000000, 0.000000000000000000 ) ) ;
#1011=CARTESIAN_POINT ( 'NONE',  ( 8.410254037844358876, 17.06698729810774395, 10.49999999999999822 ) ) ;
#1012=ORIENTED_EDGE ( 'NONE', *, *, #30842, .F. ) ;
#1015=AXIS2_PLACEMENT_3D ( 'NONE', #7326, #10794, #26626 ) ;
#1016=ORIENTED_EDGE ( 'NONE', *, *, #29221, .F. ) ;
#1018=DIRECTION ( 'NONE',  ( 0.000000000000000000, 0.000000000000000000, 1.000000000000000000 ) ) ;
#1019=LINE ( 'NONE', #9364, #17089 ) ;
#1020=CARTESIAN_POINT ( 'NONE',  ( -8.401171878996500197, 21.11424711454089476, 9.000000000000001776 ) ) ;
#1022=LINE ( 'NONE', #19908, #16824 ) ;
#1025=PLANE ( 'NONE',  #27349 ) ;
#1026=EDGE_CURVE ( 'NONE', #1570, #35419, #19056, .T. ) ;
#1027=FACE_OUTER_BOUND ( 'NONE', #29182, .T. ) ;
#1030=ORIENTED_EDGE ( 'NONE', *, *, #916, .T. ) ;
#1032=CARTESIAN_POINT ( 'NONE',  ( 0.000000000000000000, 22.50000000000000355, 7.000000000000000000 ) ) ;
#1035=DIRECTION ( 'NONE',  ( -1.000000000000000000, 0.000000000000000000, 0.000000000000000000 ) ) ;
#1036=ORIENTED_EDGE ( 'NONE', *, *, #9740, .F. ) ;
#1037=AXIS2_PLACEMENT_3D ( 'NONE', #25052, #28298, #18959 ) ;
#1043=DIRECTION ( 'NONE',  ( 0.9781476007338070211, 0.2079116908177532919, 0.000000000000000000 ) ) ;
#1044=ORIENTED_EDGE ( 'NONE', *, *, #7401, .F. ) ;
#1045=ORIENTED_EDGE ( 'NONE', *, *, #14187, .F. ) ;
#1048=CARTESIAN_POINT ( 'NONE',  ( -12.60100158617414934, 14.64745807297398983, 10.87262190629281378 ) ) ;
#1050=PLANE ( 'NONE',  #22867 ) ;
#1055=EDGE_CURVE ( 'NONE', #39013, #24143, #4522, .T. ) ;
#1056=ORIENTED_EDGE ( 'NONE', *, *, #19803, .T. ) ;
#1058=LINE ( 'NONE', #30989, #24781 ) ;
#1059=VERTEX_POINT ( 'NONE', #26046 ) ;
#1065=VECTOR ( 'NONE', #39012, 1000.000000000000000 ) ;
#1068=AXIS2_PLACEMENT_3D ( 'NONE', #29176, #32221, #13524 ) ;
#1070=AXIS2_PLACEMENT_3D ( 'NONE', #25458, #22617, #31769 ) ;
#1071=EDGE_CURVE ( 'NONE', #7930, #30348, #29905, .T. ) ;
#1073=B_SPLINE_CURVE_WITH_KNOTS ( 'NONE', 3,
 ( #35093, #37939, #19246, #4618, #7247, #765 ),
 .UNSPECIFIED., .F., .F.,
 ( 4, 2, 4 ),
 ( 0.000000000000000000, 0.5000000000000000000, 1.000000000000000000 ),
 .UNSPECIFIED. ) ;
#1075=CARTESIAN_POINT ( 'NONE',  ( -11.48173768534022976, 32.16538668264431777, 10.63089969389957012 ) ) ;
#1082=VERTEX_POINT ( 'NONE', #1477 ) ;
#1084=VERTEX_POINT ( 'NONE', #23210 ) ;
#1087=DIRECTION ( 'NONE',  ( -0.000000000000000000, -0.000000000000000000, -1.000000000000000000 ) ) ;
#1092=ORIENTED_EDGE ( 'NONE', *, *, #36685, .T. ) ;
#1094=CARTESIAN_POINT ( 'NONE',  ( -8.160254037844437036, 16.63397459621563712, 10.49999999999999822 ) ) ;
#1097=ORIENTED_EDGE ( 'NONE', *, *, #1427, .T. ) ;
#1102=EDGE_CURVE ( 'NONE', #6805, #11440, #7390, .T. ) ;
#1106=EDGE_CURVE ( 'NONE', #5248, #38699, #11028, .T. ) ;
#1108=EDGE_CURVE ( 'NONE', #22676, #5593, #20373, .T. ) ;
#1113=ORIENTED_EDGE ( 'NONE', *, *, #23489, .F. ) ;
#1115=CARTESIAN_POINT ( 'NONE',  ( -13.99633081586299532, 26.34670874090678439, 10.83333333333333570 ) ) ;
#1118=EDGE_CURVE ( 'NONE', #7593, #21179, #16509, .T. ) ;
#1119=CONICAL_SURFACE ( 'NONE', #1797, 1.000000000000002665, 0.7853981633974509435 ) ;
#1120=CARTESIAN_POINT ( 'NONE',  ( 23.80624316739448787, 27.22568555153026537, 7.000000000000000000 ) ) ;
#1121=FACE_OUTER_BOUND ( 'NONE', #18738, .T. ) ;
#1122=CARTESIAN_POINT ( 'NONE',  ( 12.80736835487432934, 15.68301270189215835, 11.00000000000000000 ) ) ;
#1123=ORIENTED_EDGE ( 'NONE', *, *, #27299, .F. ) ;
#1124=DIRECTION ( 'NONE',  ( 1.000000000000000000, 0.000000000000000000, 0.000000000000000000 ) ) ;
#1128=PLANE ( 'NONE',  #15137 ) ;
#1129=DIRECTION ( 'NONE',  ( 1.224646799147351235E-16, -1.000000000000000000, 0.000000000000000000 ) ) ;
#1131=AXIS2_PLACEMENT_3D ( 'NONE', #23713, #26563, #39745 ) ;
#1133=ORIENTED_EDGE ( 'NONE', *, *, #27197, .F. ) ;
#1137=DIRECTION ( 'NONE',  ( -0.3090169943749450643, 0.9510565162951544194, -0.000000000000000000 ) ) ;
#1141=ORIENTED_EDGE ( 'NONE', *, *, #7030, .T. ) ;
#1143=LINE ( 'NONE', #31610, #30909 ) ;
#1151=CARTESIAN_POINT ( 'NONE',  ( -5.473344025737326923, 14.11593743010433499, 10.00000000000000000 ) ) ;
#1152=CARTESIAN_POINT ( 'NONE',  ( -12.63195416618315825, 14.41050271297376462, 7.485646746502369275 ) ) ;
#1153=EDGE_CURVE ( 'NONE', #21780, #5670, #17808, .T. ) ;
#1155=ORIENTED_EDGE ( 'NONE', *, *, #7543, .F. ) ;
#1157=VECTOR ( 'NONE', #7333, 1000.000000000000000 ) ;
#1158=VECTOR ( 'NONE', #19430, 1000.000000000000000 ) ;
#1160=EDGE_LOOP ( 'NONE', ( #5743, #16893, #6841, #25465 ) ) ;
#1161=DIRECTION ( 'NONE',  ( -0.000000000000000000, -0.000000000000000000, -1.000000000000000000 ) ) ;
#1162=CYLINDRICAL_SURFACE ( 'NONE', #25192, 0.4999999999999999445 ) ;
#1165=ORIENTED_EDGE ( 'NONE', *, *, #15702, .F. ) ;
#1166=ORIENTED_EDGE ( 'NONE', *, *, #37930, .F. ) ;
#1167=DIRECTION ( 'NONE',  ( 0.3706816908110067699, -0.7275037805840999239, 0.5773502691896271743 ) ) ;
#1169=ADVANCED_FACE ( 'NONE', ( #6654 ), #30108, .T. ) ;
#1170=CARTESIAN_POINT ( 'NONE',  ( 13.14827996435953139, 25.72067290776661608, 10.00000000000000000 ) ) ;
#1171=ORIENTED_EDGE ( 'NONE', *, *, #36222, .T. ) ;
#1172=EDGE_CURVE ( 'NONE', #37413, #7627, #15815, .T. ) ;
#1176=FACE_OUTER_BOUND ( 'NONE', #21976, .T. ) ;
#1177=PLANE ( 'NONE',  #27529 ) ;
#1178=DIRECTION ( 'NONE',  ( 0.000000000000000000, 0.000000000000000000, 1.000000000000000000 ) ) ;
#1181=AXIS2_PLACEMENT_3D ( 'NONE', #12643, #53, #25031 ) ;
#1182=ORIENTED_EDGE ( 'NONE', *, *, #28357, .T. ) ;
#1183=EDGE_CURVE ( 'NONE', #36822, #20981, #34308, .T. ) ;
#1185=CARTESIAN_POINT ( 'NONE',  ( 3.503793317224327186, 8.420815634768674229, 7.000000000000000000 ) ) ;
#1186=DIRECTION ( 'NONE',  ( -0.000000000000000000, -0.000000000000000000, -1.000000000000000000 ) ) ;
#1188=CARTESIAN_POINT ( 'NONE',  ( -2.525645716490711123, 8.212903943950955465, 11.00000000000000000 ) ) ;
#1192=DIRECTION ( 'NONE',  ( 0.000000000000000000, 0.000000000000000000, 1.000000000000000000 ) ) ;
#1193=AXIS2_PLACEMENT_3D ( 'NONE', #14848, #27235, #11798 ) ;
#1198=DIRECTION ( 'NONE',  ( 1.000000000000000000, 0.000000000000000000, 0.000000000000000000 ) ) ;
#1199=CARTESIAN_POINT ( 'NONE',  ( 11.94134295108989896, 16.18301270189217433, 10.00000000000000000 ) ) ;
#1200=EDGE_CURVE ( 'NONE', #11801, #6957, #37554, .T. ) ;
#1201=ORIENTED_EDGE ( 'NONE', *, *, #17627, .T. ) ;
#1203=EDGE_CURVE ( 'NONE', #36455, #445, #34657, .T. ) ;
#1205=EDGE_CURVE ( 'NONE', #3451, #1436, #12018, .T. ) ;
#1206=LINE ( 'NONE', #13990, #38384 ) ;
#1209=DIRECTION ( 'NONE',  ( 0.000000000000000000, 0.000000000000000000, 1.000000000000000000 ) ) ;
#1211=ORIENTED_EDGE ( 'NONE', *, *, #23289, .F. ) ;
#1215=CONICAL_SURFACE ( 'NONE', #13527, 1.000000000000002665, 0.7853981633974547183 ) ;
#1219=CARTESIAN_POINT ( 'NONE',  ( 2.672146553953313131, 12.33340603770390764, 10.50000000000000000 ) ) ;
#1221=DIRECTION ( 'NONE',  ( 0.000000000000000000, 0.000000000000000000, -1.000000000000000000 ) ) ;
#1222=CARTESIAN_POINT ( 'NONE',  ( 8.910254037844365982, 17.93301270189218855, 10.50000000000000000 ) ) ;
#1225=CARTESIAN_POINT ( 'NONE',  ( 0.5000000000000000000, 37.50000000000000711, 10.49999999999999822 ) ) ;
#1227=EDGE_CURVE ( 'NONE', #29281, #13694, #28202, .T. ) ;
#1230=CARTESIAN_POINT ( 'NONE',  ( 13.63581098909226874, 27.45627467658428955, 7.000000000000000000 ) ) ;
#1233=ORIENTED_EDGE ( 'NONE', *, *, #26995, .F. ) ;
#1235=LINE ( 'NONE', #22751, #18810 ) ;
#1237=DIRECTION ( 'NONE',  ( 0.000000000000000000, 0.000000000000000000, 1.000000000000000000 ) ) ;
#1238=DIRECTION ( 'NONE',  ( 0.9781476007338041345, -0.2079116908177664202, 0.000000000000000000 ) ) ;
#1239=VECTOR ( 'NONE', #27661, 1000.000000000000000 ) ;
#1242=VECTOR ( 'NONE', #27565, 1000.000000000000000 ) ;
#1245=FACE_OUTER_BOUND ( 'NONE', #6644, .T. ) ;
#1246=ORIENTED_EDGE ( 'NONE', *, *, #32743, .T. ) ;
#1247=ORIENTED_EDGE ( 'NONE', *, *, #950, .T. ) ;
#1250=DIRECTION ( 'NONE',  ( -0.7032331762534058672, -0.07391278520355742954, -0.7071067811865467956 ) ) ;
#1253=LINE ( 'NONE', #10392, #32639 ) ;
#1254=ORIENTED_EDGE ( 'NONE', *, *, #37582, .T. ) ;
#1256=CARTESIAN_POINT ( 'NONE',  ( 14.42035624161478857, 26.65972665747660031, 10.49999999999999822 ) ) ;
#1257=DIRECTION ( 'NONE',  ( -0.1045284632676570929, -0.9945218953682730678, 0.000000000000000000 ) ) ;
#1263=DIRECTION ( 'NONE',  ( 0.1045284632676437842, -0.9945218953682742891, 0.000000000000000000 ) ) ;
#1265=ORIENTED_EDGE ( 'NONE', *, *, #18694, .F. ) ;
#1268=DIRECTION ( 'NONE',  ( -1.000000000000000000, -1.224646799147351235E-16, 0.000000000000000000 ) ) ;
#1271=DIRECTION ( 'NONE',  ( -1.000000000000000000, 0.000000000000000000, 0.000000000000000000 ) ) ;
#1272=LINE ( 'NONE', #13655, #19517 ) ;
#1280=ORIENTED_EDGE ( 'NONE', *, *, #14981, .F. ) ;
#1285=CARTESIAN_POINT ( 'NONE',  ( 10.44103466624280507, 32.57396620494213124, 10.99999999999999645 ) ) ;
#1292=CARTESIAN_POINT ( 'NONE',  ( -11.11016527260153630, 31.83082137946488643, 7.000000000000000000 ) ) ;
#1294=DIRECTION ( 'NONE',  ( -1.000000000000000000, 0.000000000000000000, 0.000000000000000000 ) ) ;
#1296=ORIENTED_EDGE ( 'NONE', *, *, #28654, .F. ) ;
#1299=CARTESIAN_POINT ( 'NONE',  ( -22.37674264578614469, 24.85189042352228839, 7.000000000000000000 ) ) ;
#1301=ORIENTED_EDGE ( 'NONE', *, *, #22155, .F. ) ;
#1303=EDGE_CURVE ( 'NONE', #21971, #24685, #2677, .T. ) ;
#1304=CARTESIAN_POINT ( 'NONE',  ( 5.187504188494417079, 36.60991850771481637, 11.00000000000000000 ) ) ;
#1306=CONICAL_SURFACE ( 'NONE', #24006, 0.9999999999999970024, 0.7853981633974552734 ) ;
#1312=ORIENTED_EDGE ( 'NONE', *, *, #25393, .F. ) ;
#1316=CARTESIAN_POINT ( 'NONE',  ( 9.840690490415068936, 20.46019347195515792, 10.50000000000000533 ) ) ;
#1318=CARTESIAN_POINT ( 'NONE',  ( -11.54426395383663539, 32.09594422634664568, 10.49999999999999822 ) ) ;
#1320=CARTESIAN_POINT ( 'NONE',  ( -0.9999999999999993339, 33.00000000000000000, 10.50000000000000178 ) ) ;
#1321=ORIENTED_EDGE ( 'NONE', *, *, #36254, .F. ) ;
#1322=ADVANCED_FACE ( 'NONE', ( #5718 ), #8061, .T. ) ;
#1323=CARTESIAN_POINT ( 'NONE',  ( -6.546529844544896726, 35.97445010452243963, 10.68306085400114469 ) ) ;
#1325=LINE ( 'NONE', #26511, #14257 ) ;
#1327=PLANE ( 'NONE',  #6311 ) ;
#1328=LINE ( 'NONE', #7615, #10590 ) ;
#1330=DIRECTION ( 'NONE',  ( -1.000000000000000000, 0.000000000000000000, 0.000000000000000000 ) ) ;
#1331=ORIENTED_EDGE ( 'NONE', *, *, #20700, .T. ) ;
#1337=ORIENTED_EDGE ( 'NONE', *, *, #16216, .F. ) ;
#1341=CARTESIAN_POINT ( 'NONE',  ( 14.31632963181209917, 26.62592636301939919, 10.82238861112333694 ) ) ;
#1344=VECTOR ( 'NONE', #28491, 1000.000000000000000 ) ;
#1348=ORIENTED_EDGE ( 'NONE', *, *, #957, .T. ) ;
#1360=FACE_OUTER_BOUND ( 'NONE', #19909, .T. ) ;
#1365=VERTEX_POINT ( 'NONE', #36801 ) ;
#1368=CIRCLE ( 'NONE', #31840, 0.5000000000000004441 ) ;
#1369=DIRECTION ( 'NONE',  ( 0.5446390350150349668, 0.8386705679454188322, -7.903458058585596061E-16 ) ) ;
#1370=ORIENTED_EDGE ( 'NONE', *, *, #15507, .T. ) ;
#1372=VECTOR ( 'NONE', #34789, 1000.000000000000114 ) ;
#1373=CARTESIAN_POINT ( 'NONE',  ( -14.97840499040354878, 21.69233280637162053, 7.455539900862802050 ) ) ;
#1374=ADVANCED_FACE ( 'NONE', ( #22106 ), #9347, .T. ) ;
#1378=CARTESIAN_POINT ( 'NONE',  ( -14.47283171447380390, 21.48159823030330529, 11.00000000000000000 ) ) ;
#1379=CYLINDRICAL_SURFACE ( 'NONE', #11271, 0.4999999999999999445 ) ;
#1381=CARTESIAN_POINT ( 'NONE',  ( 10.10646936306337729, 32.94553861768082470, 9.500000000000000000 ) ) ;
#1382=EDGE_LOOP ( 'NONE', ( #25850, #30866, #28267, #16850 ) ) ;
#1385=CARTESIAN_POINT ( 'NONE',  ( -0.5934445985556291436, 37.50000000000000711, 10.49999999999999822 ) ) ;
#1387=AXIS2_PLACEMENT_3D ( 'NONE', #12365, #28398, #31452 ) ;
#1390=CARTESIAN_POINT ( 'NONE',  ( -4.987329993433320396E-14, 13.65543219052647927, 7.000000000000000000 ) ) ;
#1395=CARTESIAN_POINT ( 'NONE',  ( 4.727507481117209309, 31.88885898370940453, 10.00000000000000000 ) ) ;
#1399=ORIENTED_EDGE ( 'NONE', *, *, #30628, .F. ) ;
#1400=ADVANCED_FACE ( 'NONE', ( #16413 ), #35301, .F. ) ;
#1402=AXIS2_PLACEMENT_3D ( 'NONE', #9572, #21954, #28251 ) ;
#1403=DIRECTION ( 'NONE',  ( -0.000000000000000000, -0.000000000000000000, -1.000000000000000000 ) ) ;
#1404=VERTEX_POINT ( 'NONE', #3817 ) ;
#1405=VECTOR ( 'NONE', #33314, 1000.000000000000000 ) ;
#1406=DIRECTION ( 'NONE',  ( 1.000000000000000000, 0.000000000000000000, 0.000000000000000000 ) ) ;
#1407=EDGE_CURVE ( 'NONE', #37972, #16754, #31408, .T. ) ;
#1411=ORIENTED_EDGE ( 'NONE', *, *, #18184, .T. ) ;
#1413=EDGE_CURVE ( 'NONE', #14680, #20195, #33151, .T. ) ;
#1416=AXIS2_PLACEMENT_3D ( 'NONE', #32542, #2255, #4697 ) ;
#1418=LINE ( 'NONE', #29444, #27453 ) ;
#1421=PLANE ( 'NONE',  #23980 ) ;
#1424=CARTESIAN_POINT ( 'NONE',  ( -2.629601561899595374, 7.723830143584053509, 10.49999999999999822 ) ) ;
#1426=LINE ( 'NONE', #13808, #32490 ) ;
#1427=EDGE_CURVE ( 'NONE', #25178, #38914, #38549, .T. ) ;
#1431=CARTESIAN_POINT ( 'NONE',  ( 6.354454053420414361, 35.54304081427980577, 7.000000000000000000 ) ) ;
#1432=CARTESIAN_POINT ( 'NONE',  ( -2.063787492809998625, 7.980908877017413694, 10.49999999999999645 ) ) ;
#1435=DIRECTION ( 'NONE',  ( 1.000000000000000000, 0.000000000000000000, 0.000000000000000000 ) ) ;
#1436=VERTEX_POINT ( 'NONE', #32050 ) ;
#1440=DIRECTION ( 'NONE',  ( -0.000000000000000000, -0.000000000000000000, -1.000000000000000000 ) ) ;
#1441=ORIENTED_EDGE ( 'NONE', *, *, #32902, .F. ) ;
#1444=DIRECTION ( 'NONE',  ( 0.000000000000000000, 0.000000000000000000, 1.000000000000000000 ) ) ;
#1445=EDGE_CURVE ( 'NONE', #11176, #10038, #11957, .T. ) ;
#1446=CARTESIAN_POINT ( 'NONE',  ( -12.74038105676665111, 14.56698729810790027, 10.49999999999999822 ) ) ;
#1447=CIRCLE ( 'NONE', #22192, 0.4999999999999997780 ) ;
#1449=LINE ( 'NONE', #8349, #28663 ) ;
#1455=LINE ( 'NONE', #16903, #16082 ) ;
#1456=ORIENTED_EDGE ( 'NONE', *, *, #37296, .T. ) ;
#1458=DIRECTION ( 'NONE',  ( 0.9781476007338072431, 0.2079116908177516265, 0.000000000000000000 ) ) ;
#1459=ORIENTED_EDGE ( 'NONE', *, *, #16258, .F. ) ;
#1461=EDGE_CURVE ( 'NONE', #11801, #13694, #16826, .T. ) ;
#1463=AXIS2_PLACEMENT_3D ( 'NONE', #33377, #21369, #3079 ) ;
#1465=EDGE_LOOP ( 'NONE', ( #32543, #28517, #29952, #26022 ) ) ;
#1470=PLANE ( 'NONE',  #5767 ) ;
#1471=AXIS2_PLACEMENT_3D ( 'NONE', #39229, #2264, #14653 ) ;
#1473=ADVANCED_FACE ( 'NONE', ( #4012 ), #1177, .T. ) ;
#1474=ADVANCED_FACE ( 'NONE', ( #4625 ), #17026, .F. ) ;
#1477=CARTESIAN_POINT ( 'NONE',  ( -10.36702044712415116, 31.16169077310601310, 7.000000000000000000 ) ) ;
#1481=LINE ( 'NONE', #13868, #13224 ) ;
#1484=EDGE_LOOP ( 'NONE', ( #15281, #34654, #5534 ) ) ;
#1487=LINE ( 'NONE', #23625, #21790 ) ;
#1489=VERTEX_POINT ( 'NONE', #28801 ) ;
#1491=ORIENTED_EDGE ( 'NONE', *, *, #37103, .T. ) ;
#1496=VECTOR ( 'NONE', #9423, 1000.000000000000114 ) ;
#1497=ORIENTED_EDGE ( 'NONE', *, *, #11640, .F. ) ;
#1502=ORIENTED_EDGE ( 'NONE', *, *, #26343, .T. ) ;
#1505=CARTESIAN_POINT ( 'NONE',  ( 11.44134295108988830, 15.31698729810772974, 7.000000000000000000 ) ) ;
#1506=LINE ( 'NONE', #19583, #6950 ) ;
#1507=EDGE_LOOP ( 'NONE', ( #5685, #4941, #29383, #39119 ) ) ;
#1510=CIRCLE ( 'NONE', #865, 0.9999999999999974465 ) ;
#1512=ORIENTED_EDGE ( 'NONE', *, *, #23760, .T. ) ;
#1515=AXIS2_PLACEMENT_3D ( 'NONE', #23057, #32207, #34854 ) ;
#1517=CIRCLE ( 'NONE', #10593, 0.4999999999999995559 ) ;
#1521=CARTESIAN_POINT ( 'NONE',  ( -15.15015520025801443, 37.49267296096588353, 9.500000000000000000 ) ) ;
#1522=CARTESIAN_POINT ( 'NONE',  ( 13.24038105676655164, 15.43301270189216368, 10.49999999999999822 ) ) ;
#1524=EDGE_LOOP ( 'NONE', ( #13086, #5976, #3796, #38278, #10393 ) ) ;
#1530=CARTESIAN_POINT ( 'NONE',  ( 14.49848586288626429, 20.47339359108930879, 11.00000000000000000 ) ) ;
#1534=ORIENTED_EDGE ( 'NONE', *, *, #21059, .F. ) ;
#1539=ADVANCED_FACE ( 'NONE', ( #34700 ), #6853, .F. ) ;
#1540=PLANE ( 'NONE',  #21107 ) ;
#1542=ORIENTED_EDGE ( 'NONE', *, *, #12015, .F. ) ;
#1544=ORIENTED_EDGE ( 'NONE', *, *, #26999, .T. ) ;
#1546=CARTESIAN_POINT ( 'NONE',  ( 14.17145697063259391, 26.57885438195654970, 10.94387467463490538 ) ) ;
#1550=CIRCLE ( 'NONE', #15810, 0.5000000000000000000 ) ;
#1556=CARTESIAN_POINT ( 'NONE',  ( -11.19134295108999311, 14.88397459621566554, 10.50000000000000000 ) ) ;
#1560=AXIS2_PLACEMENT_3D ( 'NONE', #4826, #17232, #29608 ) ;
#1562=EDGE_LOOP ( 'NONE', ( #30202, #37119, #17318, #13317 ) ) ;
#1565=EDGE_CURVE ( 'NONE', #37722, #22206, #24914, .T. ) ;
#1566=SURFACE_STYLE_FILL_AREA ( #8256 ) ;
#1569=AXIS2_PLACEMENT_3D ( 'NONE', #19000, #31392, #18413 ) ;
#1570=VERTEX_POINT ( 'NONE', #22899 ) ;
#1571=CARTESIAN_POINT ( 'NONE',  ( -21.94497077913238314, 33.50980436007203878, 9.500000000000000000 ) ) ;
#1574=EDGE_LOOP ( 'NONE', ( #25578, #22925, #37462, #6000 ) ) ;
#1578=DIRECTION ( 'NONE',  ( 0.6724985119639580455, -0.2185080122244185408, -0.7071067811865444641 ) ) ;
#1579=DIRECTION ( 'NONE',  ( -0.7071067811865474617, 0.000000000000000000, -0.7071067811865474617 ) ) ;
#1580=PRODUCT_DEFINITION ( 'UNKNOWN', '', #13877, #24826 ) ;
#1583=AXIS2_PLACEMENT_3D ( 'NONE', #2088, #14468, #37006 ) ;
#1585=CARTESIAN_POINT ( 'NONE',  ( -13.37378135583788286, 20.59160479820268108, 10.00000000000000000 ) ) ;
#1586=VERTEX_POINT ( 'NONE', #2586 ) ;
#1588=FACE_OUTER_BOUND ( 'NONE', #22780, .T. ) ;
#1593=CARTESIAN_POINT ( 'NONE',  ( -5.947717410344456113, 34.62949535663729250, 9.500000000000000000 ) ) ;
#1596=DIRECTION ( 'NONE',  ( -1.000000000000000000, 0.000000000000000000, 0.000000000000000000 ) ) ;
#1605=ORIENTED_EDGE ( 'NONE', *, *, #26621, .T. ) ;
#1606=DIRECTION ( 'NONE',  ( 0.1045284632676566766, 0.9945218953682730678, 0.000000000000000000 ) ) ;
#1608=FACE_OUTER_BOUND ( 'NONE', #23351, .T. ) ;
#1611=EDGE_CURVE ( 'NONE', #22260, #113, #18363, .T. ) ;
#1616=CIRCLE ( 'NONE', #27560, 0.5000000000000004441 ) ;
#1617=EDGE_LOOP ( 'NONE', ( #6826, #36816, #20076, #26907 ) ) ;
#1620=ORIENTED_EDGE ( 'NONE', *, *, #28007, .T. ) ;
#1623=CARTESIAN_POINT ( 'NONE',  ( -9.831584923911586671, 26.22020669908462764, 10.50000000000000000 ) ) ;
#1626=DIRECTION ( 'NONE',  ( 1.000000000000000000, 0.000000000000000000, 0.000000000000000000 ) ) ;
#1627=ORIENTED_EDGE ( 'NONE', *, *, #22674, .T. ) ;
#1628=DIRECTION ( 'NONE',  ( 0.000000000000000000, 0.000000000000000000, 1.000000000000000000 ) ) ;
#1629=PLANE ( 'NONE',  #29300 ) ;
#1630=CYLINDRICAL_SURFACE ( 'NONE', #11080, 6.000000000000003553 ) ;
#1631=EDGE_CURVE ( 'NONE', #25278, #4444, #33076, .T. ) ;
#1635=CARTESIAN_POINT ( 'NONE',  ( -4.987329993433320396E-14, 13.65543219052647927, 9.000000000000001776 ) ) ;
#1636=DIRECTION ( 'NONE',  ( -0.7071067811865503483, 0.000000000000000000, -0.7071067811865446862 ) ) ;
#1639=CARTESIAN_POINT ( 'NONE',  ( -6.572794801194226544, 16.58182897866500127, 9.000000000000001776 ) ) ;
#1645=DIRECTION ( 'NONE',  ( -0.000000000000000000, -0.000000000000000000, 1.000000000000000000 ) ) ;
#1652=AXIS2_PLACEMENT_3D ( 'NONE', #24702, #28341, #15562 ) ;
#1655=DIRECTION ( 'NONE',  ( 0.000000000000000000, 0.000000000000000000, 1.000000000000000000 ) ) ;
#1656=ORIENTED_EDGE ( 'NONE', *, *, #3598, .F. ) ;
#1658=FACE_OUTER_BOUND ( 'NONE', #39573, .T. ) ;
#1659=LINE ( 'NONE', #20755, #17439 ) ;
#1661=ORIENTED_EDGE ( 'NONE', *, *, #25292, .T. ) ;
#1663=CARTESIAN_POINT ( 'NONE',  ( -8.118377661053486349, 10.47536095541708967, 11.00000000000000000 ) ) ;
#1664=ORIENTED_EDGE ( 'NONE', *, *, #22285, .F. ) ;
#1671=DIRECTION ( 'NONE',  ( 0.5877852522924686962, -0.8090169943749506709, 0.000000000000000000 ) ) ;
#1674=VERTEX_POINT ( 'NONE', #20679 ) ;
#1676=AXIS2_PLACEMENT_3D ( 'NONE', #9385, #27868, #33971 ) ;
#1677=EDGE_CURVE ( 'NONE', #4321, #14858, #2166, .T. ) ;
#1680=VECTOR ( 'NONE', #22961, 1000.000000000000000 ) ;
#1681=DIRECTION ( 'NONE',  ( -0.000000000000000000, -0.000000000000000000, -1.000000000000000000 ) ) ;
#1682=EDGE_CURVE ( 'NONE', #30242, #19894, #9951, .T. ) ;
#1686=CARTESIAN_POINT ( 'NONE',  ( -13.30786737757920335, 15.60543024394081080, 10.49999999999999822 ) ) ;
#1687=CARTESIAN_POINT ( 'NONE',  ( 0.5000000000000001110, 37.00000000000000711, 9.500000000000000000 ) ) ;
#1688=ORIENTED_EDGE ( 'NONE', *, *, #32117, .T. ) ;
#1692=EDGE_CURVE ( 'NONE', #37009, #39268, #29406, .T. ) ;
#1696=EDGE_LOOP ( 'NONE', ( #16701, #34705, #38462, #6147 ) ) ;
#1698=ORIENTED_EDGE ( 'NONE', *, *, #13240, .F. ) ;
#1700=FACE_OUTER_BOUND ( 'NONE', #6725, .T. ) ;
#1702=CARTESIAN_POINT ( 'NONE',  ( -14.57486473880221745, 26.18419839932921533, 7.000000000000000000 ) ) ;
#1703=EDGE_LOOP ( 'NONE', ( #29129, #16048, #24200, #27157 ) ) ;
#1712=EDGE_CURVE ( 'NONE', #27384, #5452, #20876, .T. ) ;
#1713=CIRCLE ( 'NONE', #23097, 6.000000000000006217 ) ;
#1717=EDGE_CURVE ( 'NONE', #11442, #35565, #7437, .T. ) ;
#1719=VECTOR ( 'NONE', #17197, 1000.000000000000000 ) ;
#1721=CIRCLE ( 'NONE', #21165, 15.00000000000000000 ) ;
#1725=CARTESIAN_POINT ( 'NONE',  ( 14.75233815192021858, 19.78246761888935268, 7.202682876670055911 ) ) ;
#1726=DIRECTION ( 'NONE',  ( 0.000000000000000000, 0.000000000000000000, -1.000000000000000000 ) ) ;
#1728=CYLINDRICAL_SURFACE ( 'NONE', #5217, 0.5000000000000000000 ) ;
#1729=DIRECTION ( 'NONE',  ( 1.000000000000000000, 0.000000000000000000, 0.000000000000000000 ) ) ;
#1732=ORIENTED_EDGE ( 'NONE', *, *, #2639, .T. ) ;
#1737=CARTESIAN_POINT ( 'NONE',  ( -14.36830325120615548, 20.48707633493503621, 9.000000000000001776 ) ) ;
#1738=CARTESIAN_POINT ( 'NONE',  ( -14.85579657860262337, 20.34187940403377581, 10.49999999999999822 ) ) ;
#1743=VECTOR ( 'NONE', #5536, 1000.000000000000000 ) ;
#1746=LINE ( 'NONE', #11487, #24987 ) ;
#1748=ORIENTED_EDGE ( 'NONE', *, *, #24410, .F. ) ;
#1749=FACE_OUTER_BOUND ( 'NONE', #3413, .T. ) ;
#1752=DIRECTION ( 'NONE',  ( 0.3090169943749457304, -0.9510565162951540863, 0.000000000000000000 ) ) ;
#1761=CARTESIAN_POINT ( 'NONE',  ( -12.59277403104497850, 14.34973136966057616, 7.455686640544903376 ) ) ;
#1767=CARTESIAN_POINT ( 'NONE',  ( 2.525645716490518389, 8.212903943950921715, 9.000000000000001776 ) ) ;
#1769=LINE ( 'NONE', #38737, #38488 ) ;
#1771=DIRECTION ( 'NONE',  ( -0.4731467892558104960, 0.5254827454987662794, -0.7071067811865450192 ) ) ;
#1773=AXIS2_PLACEMENT_3D ( 'NONE', #27581, #5638, #21092 ) ;
#1774=ORIENTED_EDGE ( 'NONE', *, *, #27618, .T. ) ;
#1779=VERTEX_POINT ( 'NONE', #11329 ) ;
#1782=DIRECTION ( 'NONE',  ( -0.3090169943749573322, -0.9510565162951505336, 0.000000000000000000 ) ) ;
#1783=DIRECTION ( 'NONE',  ( -0.3090169943749573878, -0.9510565162951503115, -0.000000000000000000 ) ) ;
#1787=DIRECTION ( 'NONE',  ( -1.000000000000000000, 0.000000000000000000, 0.000000000000000000 ) ) ;
#1788=ORIENTED_EDGE ( 'NONE', *, *, #1813, .T. ) ;
#1790=CARTESIAN_POINT ( 'NONE',  ( 9.831584923911648843, 26.22020669908450330, 11.00000000000000000 ) ) ;
#1791=CARTESIAN_POINT ( 'NONE',  ( -13.67111072870484811, 27.95752071293692964, 10.49999999999999822 ) ) ;
#1795=FACE_OUTER_BOUND ( 'NONE', #40017, .T. ) ;
#1797=AXIS2_PLACEMENT_3D ( 'NONE', #34578, #6336, #21983 ) ;
#1803=DIRECTION ( 'NONE',  ( -1.224646799147351235E-16, 1.000000000000000000, 0.000000000000000000 ) ) ;
#1804=EDGE_LOOP ( 'NONE', ( #23516, #20092, #3804, #30968 ) ) ;
#1805=B_SPLINE_CURVE_WITH_KNOTS ( 'NONE', 3,
 ( #22643, #10263, #16973, #35049 ),
 .UNSPECIFIED., .F., .F.,
 ( 4, 4 ),
 ( 0.000000000000000000, 1.000000000000000000 ),
 .UNSPECIFIED. ) ;
#1809=CIRCLE ( 'NONE', #6343, 15.00000000000000000 ) ;
#1810=PLANE ( 'NONE',  #39047 ) ;
#1811=ORIENTED_EDGE ( 'NONE', *, *, #34625, .T. ) ;
#1812=CARTESIAN_POINT ( 'NONE',  ( 22.37674264578617667, 24.85189042352198641, 7.000000000000000000 ) ) ;
#1813=EDGE_CURVE ( 'NONE', #35819, #22041, #23556, .T. ) ;
#1814=DIRECTION ( 'NONE',  ( 0.3090169943749450643, -0.9510565162951544194, 0.000000000000000000 ) ) ;
#1817=ORIENTED_EDGE ( 'NONE', *, *, #21931, .T. ) ;
#1819=ADVANCED_FACE ( 'NONE', ( #2186 ), #8875, .T. ) ;
#1820=ADVANCED_FACE ( 'NONE', ( #21265 ), #15965, .F. ) ;
#1823=CARTESIAN_POINT ( 'NONE',  ( 10.72918489117958174, 32.98258515686296732, 7.499999999999997335 ) ) ;
#1824=VERTEX_POINT ( 'NONE', #37503 ) ;
#1831=CIRCLE ( 'NONE', #28436, 6.000000000000003553 ) ;
#1832=DIRECTION ( 'NONE',  ( -0.5720614028176804755, -0.4156269377774462481, 0.7071067811865549002 ) ) ;
#1834=CYLINDRICAL_SURFACE ( 'NONE', #29490, 0.5000000000000004441 ) ;
#1835=DIRECTION ( 'NONE',  ( 0.000000000000000000, 0.000000000000000000, 1.000000000000000000 ) ) ;
#1836=AXIS2_PLACEMENT_3D ( 'NONE', #37041, #11861, #2523 ) ;
#1837=CARTESIAN_POINT ( 'NONE',  ( 10.10646936306337729, 32.94553861768082470, 11.00000000000000000 ) ) ;
#1842=CARTESIAN_POINT ( 'NONE',  ( 12.80736835487432934, 15.68301270189215835, 11.00000000000000000 ) ) ;
#1843=FACE_OUTER_BOUND ( 'NONE', #7888, .T. ) ;
#1844=EDGE_CURVE ( 'NONE', #22956, #31091, #3177, .T. ) ;
#1845=ADVANCED_FACE ( 'NONE', ( #2978 ), #19027, .T. ) ;
#1848=DIRECTION ( 'NONE',  ( 0.7431448254773862505, -0.6691306063588670083, 0.000000000000000000 ) ) ;
#1852=LINE ( 'NONE', #11188, #36742 ) ;
#1853=EDGE_LOOP ( 'NONE', ( #36304, #15483, #37549, #20225, #29233, #37704, #6383 ) ) ;
#1854=ORIENTED_EDGE ( 'NONE', *, *, #31044, .T. ) ;
#1856=CARTESIAN_POINT ( 'NONE',  ( 10.44103466624280685, 32.57396620494213124, 7.000000000000000000 ) ) ;
#1858=AXIS2_PLACEMENT_3D ( 'NONE', #18848, #21298, #157 ) ;
#1859=VECTOR ( 'NONE', #13838, 999.9999999999998863 ) ;
#1861=DIRECTION ( 'NONE',  ( 0.000000000000000000, -1.000000000000000000, -0.000000000000000000 ) ) ;
#1862=ORIENTED_EDGE ( 'NONE', *, *, #14052, .F. ) ;
#1865=FACE_OUTER_BOUND ( 'NONE', #11055, .T. ) ;
#1866=CARTESIAN_POINT ( 'NONE',  ( -2.109203785269543996, 7.931710454523169140, 10.49999999999999822 ) ) ;
#1867=CIRCLE ( 'NONE', #33659, 1.000000000000000444 ) ;
#1868=ORIENTED_EDGE ( 'NONE', *, *, #12854, .F. ) ;
#1870=EDGE_CURVE ( 'NONE', #15928, #13281, #21656, .T. ) ;
#1872=VERTEX_POINT ( 'NONE', #24907 ) ;
#1874=AXIS2_PLACEMENT_3D ( 'NONE', #15398, #5853, #11953 ) ;
#1876=ORIENTED_EDGE ( 'NONE', *, *, #24459, .F. ) ;
#1879=CARTESIAN_POINT ( 'NONE',  ( 4.984135866956514782, 36.15314577889351000, 9.500000000000000000 ) ) ;
#1882=ORIENTED_EDGE ( 'NONE', *, *, #24342, .T. ) ;
#1883=CARTESIAN_POINT ( 'NONE',  ( -8.744117900323422177, 12.16605582823074982, 10.50000000000000000 ) ) ;
#1884=TOROIDAL_SURFACE ( 'NONE', #18100, 1.000000000000000000, 0.5000000000000000000 ) ;
#1886=AXIS2_PLACEMENT_3D ( 'NONE', #1185, #28606, #29412 ) ;
#1887=CARTESIAN_POINT ( 'NONE',  ( -4.577399223880544099, 35.23960032125097541, 9.500000000000000000 ) ) ;
#1895=ORIENTED_EDGE ( 'NONE', *, *, #32466, .F. ) ;
#1897=VERTEX_POINT ( 'NONE', #9678 ) ;
#1904=EDGE_LOOP ( 'NONE', ( #9050, #2463, #21703, #1664 ) ) ;
#1906=CARTESIAN_POINT ( 'NONE',  ( 13.49038105676655164, 15.86602540378438064, 7.000000000000000000 ) ) ;
#1908=CARTESIAN_POINT ( 'NONE',  ( -13.63581098909220479, 27.45627467658446008, 7.000000000000000000 ) ) ;
#1909=ORIENTED_EDGE ( 'NONE', *, *, #18794, .F. ) ;
#1914=VERTEX_POINT ( 'NONE', #5826 ) ;
#1918=ORIENTED_EDGE ( 'NONE', *, *, #2599, .F. ) ;
#1920=EDGE_CURVE ( 'NONE', #4426, #6906, #26801, .T. ) ;
#1922=CIRCLE ( 'NONE', #6417, 0.5000000000000004441 ) ;
#1923=ADVANCED_FACE ( 'NONE', ( #2776 ), #6602, .T. ) ;
#1925=ORIENTED_EDGE ( 'NONE', *, *, #35246, .F. ) ;
#1929=DIRECTION ( 'NONE',  ( 0.5877852522924689183, -0.8090169943749506709, 0.000000000000000000 ) ) ;
#1930=EDGE_CURVE ( 'NONE', #36749, #29091, #33866, .T. ) ;
#1932=CARTESIAN_POINT ( 'NONE',  ( -8.137585970691990411, 29.15429895402940730, 10.00000000000000000 ) ) ;
#1934=CARTESIAN_POINT ( 'NONE',  ( -5.022716998311358871, 36.63466579533663747, 7.202682876670054135 ) ) ;
#1935=VERTEX_POINT ( 'NONE', #15567 ) ;
#1941=EDGE_CURVE ( 'NONE', #6642, #7803, #7968, .T. ) ;
#1942=DIRECTION ( 'NONE',  ( 0.2079116908177522649, -0.9781476007338071321, 0.000000000000000000 ) ) ;
#1947=VECTOR ( 'NONE', #31201, 1000.000000000000000 ) ;
#1952=CARTESIAN_POINT ( 'NONE',  ( 0.000000000000000000, 22.50000000000000355, 7.000000000000000000 ) ) ;
#1954=EDGE_LOOP ( 'NONE', ( #13424, #12399, #14022, #25865 ) ) ;
#1955=DIRECTION ( 'NONE',  ( 0.3090169943749573878, 0.9510565162951503115, 0.000000000000000000 ) ) ;
#1956=VECTOR ( 'NONE', #12953, 999.9999999999998863 ) ;
#1957=ORIENTED_EDGE ( 'NONE', *, *, #21762, .T. ) ;
#1967=CARTESIAN_POINT ( 'NONE',  ( 12.80736835487433289, 15.68301270189216545, 11.00000000000000000 ) ) ;
#1969=CARTESIAN_POINT ( 'NONE',  ( 2.199596516245916789, 8.143600047011672061, 10.66666666666666075 ) ) ;
#1970=VERTEX_POINT ( 'NONE', #6017 ) ;
#1972=EDGE_CURVE ( 'NONE', #17859, #7248, #12445, .T. ) ;
#1974=ADVANCED_FACE ( 'NONE', ( #6218 ), #9290, .T. ) ;
#1976=ADVANCED_FACE ( 'NONE', ( #22850 ), #10674, .F. ) ;
#1978=CARTESIAN_POINT ( 'NONE',  ( -6.282361020112263716, 14.70372268239681190, 10.50000000000000533 ) ) ;
#1979=B_SPLINE_CURVE_WITH_KNOTS ( 'NONE', 3,
 ( #15645, #28031, #34336, #6487, #9751, #3449, #4247, #37974 ),
 .UNSPECIFIED., .F., .F.,
 ( 4, 2, 2, 4 ),
 ( 0.000000000000000000, 0.0002364868538934304361, 0.0004729737077868608722, 0.0009459474155737221781 ),
 .UNSPECIFIED. ) ;
#1980=SURFACE_SIDE_STYLE ('',( #1566 ) ) ;
#1982=ORIENTED_EDGE ( 'NONE', *, *, #11505, .F. ) ;
#1984=DIRECTION ( 'NONE',  ( -0.6123724356957936932, -0.3535533905932657373, -0.7071067811865523467 ) ) ;
#1985=CARTESIAN_POINT ( 'NONE',  ( -2.525645716490711568, 8.212903943950959018, 9.500000000000000000 ) ) ;
#1986=EDGE_LOOP ( 'NONE', ( #20235, #23112, #9530, #9981 ) ) ;
#1989=CARTESIAN_POINT ( 'NONE',  ( 14.81881748179396219, 20.25565617689056452, 10.49999999999999822 ) ) ;
#1990=DIRECTION ( 'NONE',  ( -0.3090169943749448977, 0.9510565162951543083, 0.000000000000000000 ) ) ;
#1992=DIRECTION ( 'NONE',  ( -0.9781476007338069101, -0.2079116908177535972, 0.000000000000000000 ) ) ;
#1993=ADVANCED_FACE ( 'NONE', ( #9866 ), #37892, .T. ) ;
#1995=CARTESIAN_POINT ( 'NONE',  ( 14.36830325120613594, 20.48707633493483371, 9.000000000000001776 ) ) ;
#1996=ORIENTED_EDGE ( 'NONE', *, *, #24508, .T. ) ;
#1997=AXIS2_PLACEMENT_3D ( 'NONE', #31151, #25638, #37442 ) ;
#1999=CARTESIAN_POINT ( 'NONE',  ( -21.55328011382844977, 16.02264588471131646, 11.00000000000000000 ) ) ;
#2003=DIRECTION ( 'NONE',  ( -0.9135454576426006446, 0.4067366430758008744, 0.000000000000000000 ) ) ;
#2005=CARTESIAN_POINT ( 'NONE',  ( -14.97009266215794021, 21.42933399866948463, 10.49999999999999822 ) ) ;
#2012=ORIENTED_EDGE ( 'NONE', *, *, #1026, .T. ) ;
#2015=VERTEX_POINT ( 'NONE', #16569 ) ;
#2017=ORIENTED_EDGE ( 'NONE', *, *, #19039, .T. ) ;
#2018=EDGE_CURVE ( 'NONE', #19442, #30652, #35888, .T. ) ;
#2019=DIRECTION ( 'NONE',  ( -1.000000000000000000, 0.000000000000000000, 0.000000000000000000 ) ) ;
#2020=DIRECTION ( 'NONE',  ( 0.1045284632676566766, 0.9945218953682730678, 0.000000000000000000 ) ) ;
#2021=VERTEX_POINT ( 'NONE', #10467 ) ;
#2023=ORIENTED_EDGE ( 'NONE', *, *, #236, .T. ) ;
#2025=VECTOR ( 'NONE', #33954, 1000.000000000000000 ) ;
#2028=CARTESIAN_POINT ( 'NONE',  ( 1.590043107810628964, 12.61456814725305442, 10.49999999999999467 ) ) ;
#2029=ORIENTED_EDGE ( 'NONE', *, *, #28253, .F. ) ;
#2031=DIRECTION ( 'NONE',  ( -0.6916548014802247346, -0.1470157664651938756, 0.7071067811865492381 ) ) ;
#2032=CARTESIAN_POINT ( 'NONE',  ( 8.007761790012084546, 9.776959832083274904, 10.49999999999999822 ) ) ;
#2040=ORIENTED_EDGE ( 'NONE', *, *, #10805, .F. ) ;
#2041=LINE ( 'NONE', #32316, #7339 ) ;
#2042=LINE ( 'NONE', #2241, #12971 ) ;
#2043=EDGE_CURVE ( 'NONE', #15223, #19849, #19655, .T. ) ;
#2045=FACE_OUTER_BOUND ( 'NONE', #24586, .T. ) ;
#2052=LINE ( 'NONE', #29469, #23768 ) ;
#2053=EDGE_CURVE ( 'NONE', #21971, #38824, #31800, .T. ) ;
#2054=VERTEX_POINT ( 'NONE', #926 ) ;
#2057=CARTESIAN_POINT ( 'NONE',  ( -5.440908595777636414, 35.94977745735568675, 7.000000000000000000 ) ) ;
#2058=DIRECTION ( 'NONE',  ( 0.9510565162951548634, 0.3090169943749434545, 0.000000000000000000 ) ) ;
#2059=CARTESIAN_POINT ( 'NONE',  ( -12.19134295108997890, 16.61602540378455117, 9.500000000000000000 ) ) ;
#2062=CARTESIAN_POINT ( 'NONE',  ( 11.11016527260166953, 31.83082137946472656, 11.00000000000000000 ) ) ;
#2065=CARTESIAN_POINT ( 'NONE',  ( -2.544902299099670362, 8.122308845603198435, 10.99387789255783332 ) ) ;
#2068=CARTESIAN_POINT ( 'NONE',  ( -13.74617375768319327, 27.96120515612786761, 10.49999999999999467 ) ) ;
#2069=EDGE_LOOP ( 'NONE', ( #28914, #13912, #28736, #3484, #2314 ) ) ;
#2074=ADVANCED_FACE ( 'NONE', ( #16165 ), #28949, .F. ) ;
#2078=CIRCLE ( 'NONE', #29962, 1.000000000000000888 ) ;
#2079=CARTESIAN_POINT ( 'NONE',  ( -3.607749162633401507, 7.931741834401821123, 10.49999999999999822 ) ) ;
#2080=ORIENTED_EDGE ( 'NONE', *, *, #19695, .T. ) ;
#2081=LINE ( 'NONE', #5120, #32752 ) ;
#2084=DIRECTION ( 'NONE',  ( 1.000000000000000000, 0.000000000000000000, 0.000000000000000000 ) ) ;
#2086=AXIS2_PLACEMENT_3D ( 'NONE', #33850, #5409, #36298 ) ;
#2088=CARTESIAN_POINT ( 'NONE',  ( 5.440908595777814050, 35.94977745735560859, 7.000000000000000000 ) ) ;
#2089=CARTESIAN_POINT ( 'NONE',  ( -13.28710325169430106, 15.51393791734817640, 10.49999999999999822 ) ) ;
#2090=CARTESIAN_POINT ( 'NONE',  ( -1.000000000000000000, 37.00000000000000711, 11.00000000000000000 ) ) ;
#2091=EDGE_CURVE ( 'NONE', #21646, #3260, #1328, .T. ) ;
#2092=ORIENTED_EDGE ( 'NONE', *, *, #33477, .F. ) ;
#2094=EDGE_LOOP ( 'NONE', ( #27297, #23033, #29887, #26081, #30239 ) ) ;
#2097=CARTESIAN_POINT ( 'NONE',  ( -14.30862178846737187, 26.15670448022670413, 10.49999999999999822 ) ) ;
#2099=EDGE_CURVE ( 'NONE', #16943, #29068, #7003, .T. ) ;
#2100=ORIENTED_EDGE ( 'NONE', *, *, #6542, .T. ) ;
#2102=EDGE_LOOP ( 'NONE', ( #14826, #14127, #27212, #32370, #31551, #19970, #30137 ) ) ;
#2104=CYLINDRICAL_SURFACE ( 'NONE', #15357, 0.5000000000000004441 ) ;
#2110=AXIS2_PLACEMENT_3D ( 'NONE', #27906, #24264, #34407 ) ;
#2112=VERTEX_POINT ( 'NONE', #13302 ) ;
#2114=CARTESIAN_POINT ( 'NONE',  ( -8.247851828378241379, 9.985713325475984448, 10.49999999999999822 ) ) ;
#2116=ORIENTED_EDGE ( 'NONE', *, *, #10994, .F. ) ;
#2120=EDGE_CURVE ( 'NONE', #14734, #7713, #10266, .T. ) ;
#2123=EDGE_CURVE ( 'NONE', #22721, #18984, #35459, .T. ) ;
#2124=CARTESIAN_POINT ( 'NONE',  ( -9.331903152615899089, 11.35703883385581037, 7.500000000000000888 ) ) ;
#2126=CARTESIAN_POINT ( 'NONE',  ( 0.5000000000000000000, 37.50000000000000711, 11.00000000000000000 ) ) ;
#2129=CARTESIAN_POINT ( 'NONE',  ( -5.537946624085890335, 36.44027069998196566, 7.500000000000000888 ) ) ;
#2130=VERTEX_POINT ( 'NONE', #25699 ) ;
#2132=DIRECTION ( 'NONE',  ( -0.9510565162951504226, 0.3090169943749573322, 0.000000000000000000 ) ) ;
#2133=CARTESIAN_POINT ( 'NONE',  ( -5.982165713378357452, 28.55918256678905465, 7.000000000000000000 ) ) ;
#2135=CARTESIAN_POINT ( 'NONE',  ( -12.80736835487442349, 15.68301270189233954, 11.00000000000000000 ) ) ;
#2136=DIRECTION ( 'NONE',  ( 0.8660254037844362651, -0.5000000000000041078, 0.000000000000000000 ) ) ;
#2139=CIRCLE ( 'NONE', #34006, 0.4999999999999997780 ) ;
#2141=VERTEX_POINT ( 'NONE', #38297 ) ;
#2147=ORIENTED_EDGE ( 'NONE', *, *, #34957, .F. ) ;
#2149=ORIENTED_EDGE ( 'NONE', *, *, #28641, .F. ) ;
#2154=CIRCLE ( 'NONE', #24846, 1.000000000000011324 ) ;
#2159=VERTEX_POINT ( 'NONE', #527 ) ;
#2162=FACE_OUTER_BOUND ( 'NONE', #37524, .T. ) ;
#2163=DIRECTION ( 'NONE',  ( 1.000000000000000000, 0.000000000000000000, 0.000000000000000000 ) ) ;
#2164=VERTEX_POINT ( 'NONE', #12909 ) ;
#2166=CIRCLE ( 'NONE', #27461, 0.5000000000000004441 ) ;
#2168=DIRECTION ( 'NONE',  ( 0.000000000000000000, 0.000000000000000000, 1.000000000000000000 ) ) ;
#2170=LINE ( 'NONE', #32449, #14167 ) ;
#2171=CARTESIAN_POINT ( 'NONE',  ( -5.237540274239744775, 35.49300472853438038, 10.00000000000000000 ) ) ;
#2172=EDGE_CURVE ( 'NONE', #17610, #9003, #24214, .T. ) ;
#2173=CIRCLE ( 'NONE', #36555, 0.5000000000000004441 ) ;
#2174=DIRECTION ( 'NONE',  ( -0.7431448254773962425, -0.6691306063588560171, 0.000000000000000000 ) ) ;
#2176=ORIENTED_EDGE ( 'NONE', *, *, #37827, .T. ) ;
#2177=DIRECTION ( 'NONE',  ( -0.8090169943749426773, 0.5877852522924797984, 0.000000000000000000 ) ) ;
#2179=CARTESIAN_POINT ( 'NONE',  ( -8.118377661053486349, 10.47536095541709145, 9.500000000000000000 ) ) ;
#2180=CYLINDRICAL_SURFACE ( 'NONE', #4086, 0.5000000000000004441 ) ;
#2182=DIRECTION ( 'NONE',  ( -0.1045284632676570929, -0.9945218953682730678, 0.000000000000000000 ) ) ;
#2183=DIRECTION ( 'NONE',  ( 0.2079116908177532363, -0.9781476007338070211, 6.938893903907217334E-15 ) ) ;
#2184=DIRECTION ( 'NONE',  ( -0.6691306063588569053, 0.7431448254773954654, 0.000000000000000000 ) ) ;
#2185=DIRECTION ( 'NONE',  ( -0.000000000000000000, -0.000000000000000000, -1.000000000000000000 ) ) ;
#2186=FACE_OUTER_BOUND ( 'NONE', #17740, .T. ) ;
#2187=ADVANCED_FACE ( 'NONE', ( #35052 ), #7206, .F. ) ;
#2195=CARTESIAN_POINT ( 'NONE',  ( -13.52529089031622078, 27.94609563178166667, 10.49999999999999822 ) ) ;
#2208=DIRECTION ( 'NONE',  ( 1.000000000000000000, 0.000000000000000000, 0.000000000000000000 ) ) ;
#2209=EDGE_LOOP ( 'NONE', ( #14768, #4118, #23816 ) ) ;
#2211=VERTEX_POINT ( 'NONE', #5571 ) ;
#2212=AXIS2_PLACEMENT_3D ( 'NONE', #2423, #39983, #33313 ) ;
#2215=CARTESIAN_POINT ( 'NONE',  ( -1.000000000000000000, 37.00000000000000711, 10.50000000000000178 ) ) ;
#2222=EDGE_CURVE ( 'NONE', #39268, #32514, #20343, .T. ) ;
#2223=AXIS2_PLACEMENT_3D ( 'NONE', #19253, #22698, #772 ) ;
#2226=ORIENTED_EDGE ( 'NONE', *, *, #21195, .F. ) ;
#2227=PLANE ( 'NONE',  #28118 ) ;
#2228=CARTESIAN_POINT ( 'NONE',  ( 14.47283171447379146, 21.48159823030311344, 7.000000000000000000 ) ) ;
#2229=DIRECTION ( 'NONE',  ( 1.000000000000000000, 0.000000000000000000, -0.000000000000000000 ) ) ;
#2230=ORIENTED_EDGE ( 'NONE', *, *, #8735, .F. ) ;
#2231=DIRECTION ( 'NONE',  ( -0.7071067811865489050, 0.000000000000000000, -0.7071067811865462405 ) ) ;
#2233=DIRECTION ( 'NONE',  ( -1.000000000000000000, 0.000000000000000000, 0.000000000000000000 ) ) ;
#2234=EDGE_CURVE ( 'NONE', #11472, #6733, #8004, .T. ) ;
#2237=AXIS2_PLACEMENT_3D ( 'NONE', #12110, #5609, #27348 ) ;
#2238=ORIENTED_EDGE ( 'NONE', *, *, #8676, .T. ) ;
#2240=DIRECTION ( 'NONE',  ( -0.000000000000000000, -0.000000000000000000, -1.000000000000000000 ) ) ;
#2241=CARTESIAN_POINT ( 'NONE',  ( 12.63581098909226341, 27.45627467658428955, 7.000000000000000000 ) ) ;
#2245=LINE ( 'NONE', #39607, #19188 ) ;
#2248=CARTESIAN_POINT ( 'NONE',  ( 11.36213480545086441, 32.05769576588207315, 10.87262190629440717 ) ) ;
#2249=ORIENTED_EDGE ( 'NONE', *, *, #12360, .F. ) ;
#2252=CYLINDRICAL_SURFACE ( 'NONE', #30846, 0.5000000000000008882 ) ;
#2253=CARTESIAN_POINT ( 'NONE',  ( -4.980911888400493481, 31.22871793335027490, 10.50000000000000533 ) ) ;
#2254=VECTOR ( 'NONE', #6076, 1000.000000000000000 ) ;
#2255=DIRECTION ( 'NONE',  ( -0.6123724356957908066, 0.3535533905932753962, 0.7071067811865500152 ) ) ;
#2256=ORIENTED_EDGE ( 'NONE', *, *, #9432, .F. ) ;
#2259=DIRECTION ( 'NONE',  ( 0.7886751345948049829, -0.2113248654051909647, 0.5773502691896350569 ) ) ;
#2260=CARTESIAN_POINT ( 'NONE',  ( -7.530592408761010326, 11.28437794979203268, 9.500000000000000000 ) ) ;
#2261=VERTEX_POINT ( 'NONE', #38704 ) ;
#2262=AXIS2_PLACEMENT_3D ( 'NONE', #25496, #22248, #3767 ) ;
#2264=DIRECTION ( 'NONE',  ( 0.000000000000000000, 0.000000000000000000, 1.000000000000000000 ) ) ;
#2267=AXIS2_PLACEMENT_3D ( 'NONE', #14457, #36006, #5316 ) ;
#2269=ORIENTED_EDGE ( 'NONE', *, *, #23711, .T. ) ;
#2272=LINE ( 'NONE', #11615, #35346 ) ;
#2275=DIRECTION ( 'NONE',  ( 0.2079116908177535972, -0.9781476007338069101, 0.000000000000000000 ) ) ;
#2276=EDGE_LOOP ( 'NONE', ( #38018, #7279, #33317, #4998 ) ) ;
#2277=CARTESIAN_POINT ( 'NONE',  ( 7.014595103779619478, 35.79644522156321074, 10.49999999999999822 ) ) ;
#2278=CARTESIAN_POINT ( 'NONE',  ( 3.161220354320216419, 12.43736188311278212, 10.49999999999999289 ) ) ;
#2279=CIRCLE ( 'NONE', #27592, 6.000000000000005329 ) ;
#2281=DIRECTION ( 'NONE',  ( 1.000000000000000000, 0.000000000000000000, 0.000000000000000000 ) ) ;
#2283=B_SPLINE_CURVE_WITH_KNOTS ( 'NONE', 3,
 ( #3022, #18468, #15412, #21314, #20913, #39390 ),
 .UNSPECIFIED., .F., .F.,
 ( 4, 2, 4 ),
 ( 0.000000000000000000, 0.5000000000000000000, 1.000000000000000000 ),
 .UNSPECIFIED. ) ;
#2286=AXIS2_PLACEMENT_3D ( 'NONE', #39508, #8231, #26524 ) ;
#2288=CARTESIAN_POINT ( 'NONE',  ( 4.780767545418608933, 35.69637305007220363, 9.500000000000000000 ) ) ;
#2292=VECTOR ( 'NONE', #37148, 1000.000000000000000 ) ;
#2294=AXIS2_PLACEMENT_3D ( 'NONE', #7981, #19987, #23433 ) ;
#2296=ADVANCED_FACE ( 'NONE', ( #39301 ), #8223, .T. ) ;
#2297=CARTESIAN_POINT ( 'NONE',  ( -2.525645716490711123, 8.212903943950955465, 11.00000000000000000 ) ) ;
#2299=ORIENTED_EDGE ( 'NONE', *, *, #4556, .T. ) ;
#2301=EDGE_LOOP ( 'NONE', ( #10276, #6341, #12281, #38075, #5978, #11958, #32596 ) ) ;
#2303=LINE ( 'NONE', #4945, #38709 ) ;
#2305=DIRECTION ( 'NONE',  ( 0.5877852522924689183, -0.8090169943749505599, -0.000000000000000000 ) ) ;
#2306=VERTEX_POINT ( 'NONE', #26711 ) ;
#2310=ORIENTED_EDGE ( 'NONE', *, *, #1930, .T. ) ;
#2312=CARTESIAN_POINT ( 'NONE',  ( -8.172817770806704019, 10.40043057260432668, 10.99387789255784043 ) ) ;
#2314=ORIENTED_EDGE ( 'NONE', *, *, #13952, .F. ) ;
#2316=ORIENTED_EDGE ( 'NONE', *, *, #21883, .F. ) ;
#2319=EDGE_CURVE ( 'NONE', #29659, #34986, #18402, .T. ) ;
#2320=ORIENTED_EDGE ( 'NONE', *, *, #20865, .T. ) ;
#2323=DIRECTION ( 'NONE',  ( -0.000000000000000000, -0.000000000000000000, -1.000000000000000000 ) ) ;
#2324=DIRECTION ( 'NONE',  ( -0.8090169943749504489, -0.5877852522924690293, 0.000000000000000000 ) ) ;
#2326=CIRCLE ( 'NONE', #34739, 0.4999999999999998335 ) ;
#2327=LINE ( 'NONE', #27101, #3162 ) ;
#2328=EDGE_CURVE ( 'NONE', #35366, #11163, #36460, .T. ) ;
#2332=CARTESIAN_POINT ( 'NONE',  ( -5.265294543811100070, 36.54569740949598611, 7.381627713044570882 ) ) ;
#2333=ORIENTED_EDGE ( 'NONE', *, *, #950, .F. ) ;
#2335=DIRECTION ( 'NONE',  ( -0.3090169943749560000, -0.9510565162951507556, 0.000000000000000000 ) ) ;
#2338=DIRECTION ( 'NONE',  ( 0.000000000000000000, 0.000000000000000000, -1.000000000000000000 ) ) ;
#2346=EDGE_CURVE ( 'NONE', #8691, #659, #11082, .T. ) ;
#2349=ORIENTED_EDGE ( 'NONE', *, *, #17055, .T. ) ;
#2350=CARTESIAN_POINT ( 'NONE',  ( 6.282361020112160688, 14.70372268239673197, 10.50000000000000000 ) ) ;
#2351=EDGE_LOOP ( 'NONE', ( #18823, #14815, #1312, #20592 ) ) ;
#2352=VECTOR ( 'NONE', #2496, 1000.000000000000000 ) ;
#2354=DIRECTION ( 'NONE',  ( -0.9510565162951540863, -0.3090169943749457304, 0.000000000000000000 ) ) ;
#2356=CARTESIAN_POINT ( 'NONE',  ( 7.983541495324169013, 10.37739674670157441, 10.83333333333332860 ) ) ;
#2357=VECTOR ( 'NONE', #20692, 1000.000000000000114 ) ;
#2360=CARTESIAN_POINT ( 'NONE',  ( 5.132330917503148626, 36.34800796123236211, 10.49999999999999822 ) ) ;
#2362=ORIENTED_EDGE ( 'NONE', *, *, #8529, .F. ) ;
#2368=EDGE_LOOP ( 'NONE', ( #6099, #35990, #11275 ) ) ;
#2371=CARTESIAN_POINT ( 'NONE',  ( 2.568190708544435541, 12.82247983807080871, 10.50000000000000000 ) ) ;
#2373=ADVANCED_FACE ( 'NONE', ( #35857 ), #9693, .T. ) ;
#2376=ORIENTED_EDGE ( 'NONE', *, *, #23048, .T. ) ;
#2379=ORIENTED_EDGE ( 'NONE', *, *, #27745, .F. ) ;
#2381=CARTESIAN_POINT ( 'NONE',  ( 8.304868622281791346, 28.96851274765995043, 10.75000000000000178 ) ) ;
#2382=AXIS2_PLACEMENT_3D ( 'NONE', #33788, #30538, #23830 ) ;
#2383=CYLINDRICAL_SURFACE ( 'NONE', #24691, 0.4999999999999997780 ) ;
#2385=CARTESIAN_POINT ( 'NONE',  ( -2.525645716490710679, 8.212903943950959018, 9.000000000000001776 ) ) ;
#2389=CARTESIAN_POINT ( 'NONE',  ( -7.249505266586148799, 35.63236627514445587, 7.102637441331451029 ) ) ;
#2393=CARTESIAN_POINT ( 'NONE',  ( -13.72389693702418789, 27.48489553602896152, 10.99387789255782977 ) ) ;
#2400=CARTESIAN_POINT ( 'NONE',  ( -12.49038105676665644, 14.13397459621567798, 10.50000000000000000 ) ) ;
#2405=DIRECTION ( 'NONE',  ( -0.000000000000000000, 1.000000000000000000, -0.000000000000000000 ) ) ;
#2409=VECTOR ( 'NONE', #14283, 999.9999999999998863 ) ;
#2412=CYLINDRICAL_SURFACE ( 'NONE', #8262, 0.5000000000000007772 ) ;
#2413=DIRECTION ( 'NONE',  ( 0.9945218953682729568, -0.1045284632676569680, 0.000000000000000000 ) ) ;
#2415=EDGE_CURVE ( 'NONE', #37418, #855, #9628, .T. ) ;
#2417=AXIS2_PLACEMENT_3D ( 'NONE', #526, #36711, #8874 ) ;
#2420=EDGE_CURVE ( 'NONE', #39537, #15928, #2763, .T. ) ;
#2423=CARTESIAN_POINT ( 'NONE',  ( -11.11016527260153630, 31.83082137946488643, 11.00000000000000000 ) ) ;
#2424=CARTESIAN_POINT ( 'NONE',  ( 14.36830325120613594, 20.48707633493483371, 7.000000000000000000 ) ) ;
#2426=DIRECTION ( 'NONE',  ( -0.8660254037844425934, -0.4999999999999933942, -3.469446951953613400E-15 ) ) ;
#2427=ORIENTED_EDGE ( 'NONE', *, *, #7350, .T. ) ;
#2428=DIRECTION ( 'NONE',  ( 0.000000000000000000, 0.000000000000000000, -1.000000000000000000 ) ) ;
#2433=VECTOR ( 'NONE', #10649, 1000.000000000000000 ) ;
#2435=CONICAL_SURFACE ( 'NONE', #40029, 1.000000000000002665, 0.7853981633974476129 ) ;
#2438=CYLINDRICAL_SURFACE ( 'NONE', #24230, 6.000000000000006217 ) ;
#2439=CARTESIAN_POINT ( 'NONE',  ( -14.70623423376111738, 19.54590544129804286, 7.000000000000000000 ) ) ;
#2441=CARTESIAN_POINT ( 'NONE',  ( -11.11016527260153808, 31.83082137946488643, 7.000000000000000000 ) ) ;
#2444=ADVANCED_FACE ( 'NONE', ( #18769 ), #33626, .F. ) ;
#2445=CARTESIAN_POINT ( 'NONE',  ( 13.30736835487433289, 15.68301270189216545, 7.499999999999997335 ) ) ;
#2446=ADVANCED_FACE ( 'NONE', ( #27312 ), #11874, .F. ) ;
#2451=DIRECTION ( 'NONE',  ( 0.000000000000000000, 0.000000000000000000, 1.000000000000000000 ) ) ;
#2452=VERTEX_POINT ( 'NONE', #31158 ) ;
#2455=DIRECTION ( 'NONE',  ( 1.000000000000000000, -6.938893903907203923E-15, 0.000000000000000000 ) ) ;
#2456=CARTESIAN_POINT ( 'NONE',  ( -11.14717238216079842, 32.53695909538301123, 7.000000000000000000 ) ) ;
#2457=DIRECTION ( 'NONE',  ( -0.3090169943749450643, 0.9510565162951544194, -0.000000000000000000 ) ) ;
#2460=CARTESIAN_POINT ( 'NONE',  ( 14.47283171447379146, 21.48159823030312054, 11.00000000000000000 ) ) ;
#2461=FACE_OUTER_BOUND ( 'NONE', #37369, .T. ) ;
#2463=ORIENTED_EDGE ( 'NONE', *, *, #32019, .T. ) ;
#2465=LINE ( 'NONE', #18700, #39083 ) ;
#2466=EDGE_CURVE ( 'NONE', #31286, #37934, #39893, .T. ) ;
#2467=ORIENTED_EDGE ( 'NONE', *, *, #25481, .F. ) ;
#2470=ADVANCED_FACE ( 'NONE', ( #6362 ), #6171, .T. ) ;
#2471=EDGE_LOOP ( 'NONE', ( #23597, #2040, #13074 ) ) ;
#2473=AXIS2_PLACEMENT_3D ( 'NONE', #36146, #39384, #10966 ) ;
#2475=CARTESIAN_POINT ( 'NONE',  ( 1.590043107810626966, 12.61456814725305975, 10.00000000000000000 ) ) ;
#2477=CIRCLE ( 'NONE', #16063, 15.00000000000000000 ) ;
#2479=ORIENTED_EDGE ( 'NONE', *, *, #31714, .F. ) ;
#2480=FACE_OUTER_BOUND ( 'NONE', #621, .T. ) ;
#2481=CARTESIAN_POINT ( 'NONE',  ( 5.644276917315719899, 36.40655018617690786, 7.000000000000000000 ) ) ;
#2486=LINE ( 'NONE', #38855, #36613 ) ;
#2487=CARTESIAN_POINT ( 'NONE',  ( -8.796116341590805021, 23.42450908139092647, 7.000000000000000000 ) ) ;
#2488=CARTESIAN_POINT ( 'NONE',  ( 14.63635198741554788, 25.78286467897733303, 7.000000000000000000 ) ) ;
#2489=ORIENTED_EDGE ( 'NONE', *, *, #37153, .T. ) ;
#2491=VECTOR ( 'NONE', #7848, 1000.000000000000000 ) ;
#2492=ORIENTED_EDGE ( 'NONE', *, *, #20432, .T. ) ;
#2496=DIRECTION ( 'NONE',  ( -0.000000000000000000, -0.000000000000000000, 1.000000000000000000 ) ) ;
#2503=CARTESIAN_POINT ( 'NONE',  ( 0.000000000000000000, 22.50000000000000355, 7.000000000000000000 ) ) ;
#2505=LINE ( 'NONE', #14485, #7498 ) ;
#2506=AXIS2_PLACEMENT_3D ( 'NONE', #26784, #20297, #27385 ) ;
#2507=VERTEX_POINT ( 'NONE', #24458 ) ;
#2510=CARTESIAN_POINT ( 'NONE',  ( 14.03781671904272521, 27.78639141342386765, 7.485646746502379933 ) ) ;
#2511=ORIENTED_EDGE ( 'NONE', *, *, #38179, .T. ) ;
#2513=CARTESIAN_POINT ( 'NONE',  ( -7.773262162581324297, 10.11013643092551284, 10.49999999999999822 ) ) ;
#2523=DIRECTION ( 'NONE',  ( 0.4999999999999933942, -0.8660254037844425934, 0.000000000000000000 ) ) ;
#2525=CIRCLE ( 'NONE', #4459, 15.00000000000000000 ) ;
#2526=CARTESIAN_POINT ( 'NONE',  ( 12.80736835487433289, 15.68301270189216545, 7.000000000000000000 ) ) ;
#2527=PLANE ( 'NONE',  #33778 ) ;
#2528=AXIS2_PLACEMENT_3D ( 'NONE', #9213, #25433, #15701 ) ;
#2530=CARTESIAN_POINT ( 'NONE',  ( -6.576253646258509278, 14.29921418520934218, 10.50000000000000000 ) ) ;
#2533=DIRECTION ( 'NONE',  ( 0.000000000000000000, 0.000000000000000000, 1.000000000000000000 ) ) ;
#2534=CARTESIAN_POINT ( 'NONE',  ( -3.399837471815634338, 8.909889435135630364, 7.499999999999997335 ) ) ;
#2536=DIRECTION ( 'NONE',  ( -0.2079116908177663092, -0.9781476007338041345, 0.000000000000000000 ) ) ;
#2539=VERTEX_POINT ( 'NONE', #18372 ) ;
#2542=EDGE_CURVE ( 'NONE', #20981, #36487, #18572, .T. ) ;
#2543=CARTESIAN_POINT ( 'NONE',  ( -5.184280209938394002, 31.68549066217158483, 10.50000000000000000 ) ) ;
#2545=ORIENTED_EDGE ( 'NONE', *, *, #16236, .F. ) ;
#2547=ORIENTED_EDGE ( 'NONE', *, *, #14351, .T. ) ;
#2549=DIRECTION ( 'NONE',  ( 1.000000000000000000, 0.000000000000000000, 0.000000000000000000 ) ) ;
#2553=VECTOR ( 'NONE', #8873, 1000.000000000000000 ) ;
#2558=ADVANCED_FACE ( 'NONE', ( #3324 ), #24800, .T. ) ;
#2561=CARTESIAN_POINT ( 'NONE',  ( -8.118377661053489902, 10.47536095541709322, 7.000000000000000000 ) ) ;
#2562=CARTESIAN_POINT ( 'NONE',  ( -10.39021566973305788, 20.90519018800560858, 10.50000000000000000 ) ) ;
#2563=EDGE_CURVE ( 'NONE', #21143, #2130, #3126, .T. ) ;
#2564=CARTESIAN_POINT ( 'NONE',  ( -14.96930490892015797, 21.54088032874991399, 7.500000000000004441 ) ) ;
#2565=VECTOR ( 'NONE', #34351, 1000.000000000000114 ) ;
#2572=CARTESIAN_POINT ( 'NONE',  ( 8.927394655428276593, 11.06314620770945290, 7.000000000000000000 ) ) ;
#2574=ORIENTED_EDGE ( 'NONE', *, *, #26846, .F. ) ;
#2575=EDGE_CURVE ( 'NONE', #13129, #10650, #30374, .T. ) ;
#2578=CARTESIAN_POINT ( 'NONE',  ( -2.629601561899595374, 7.723830143584053509, 11.00000000000000000 ) ) ;
#2581=CARTESIAN_POINT ( 'NONE',  ( -5.139519228945863993, 36.36965741570538313, 10.49999999999999467 ) ) ;
#2585=DIRECTION ( 'NONE',  ( 1.000000000000000000, 0.000000000000000000, 0.000000000000000000 ) ) ;
#2586=CARTESIAN_POINT ( 'NONE',  ( 6.101049646137017390, 36.20318186463901355, 7.000000000000000000 ) ) ;
#2593=LINE ( 'NONE', #21272, #32192 ) ;
#2597=ORIENTED_EDGE ( 'NONE', *, *, #13699, .F. ) ;
#2598=CARTESIAN_POINT ( 'NONE',  ( -4.096822963000303019, 8.035697679810709815, 11.00000000000000000 ) ) ;
#2599=EDGE_CURVE ( 'NONE', #11176, #9944, #13133, .T. ) ;
#2607=ORIENTED_EDGE ( 'NONE', *, *, #11866, .F. ) ;
#2610=VERTEX_POINT ( 'NONE', #3520 ) ;
#2612=DIRECTION ( 'NONE',  ( 0.4156269377774681195, 0.5720614028176796984, -0.7071067811865426878 ) ) ;
#2615=ORIENTED_EDGE ( 'NONE', *, *, #12904, .T. ) ;
#2620=CARTESIAN_POINT ( 'NONE',  ( -11.94134295108998245, 16.18301270189233065, 10.50000000000000000 ) ) ;
#2621=PLANE ( 'NONE',  #29940 ) ;
#2624=ORIENTED_EDGE ( 'NONE', *, *, #4066, .F. ) ;
#2626=CYLINDRICAL_SURFACE ( 'NONE', #7890, 0.5000000000000004441 ) ;
#2627=DIRECTION ( 'NONE',  ( -0.6691306063588569053, 0.7431448254773954654, -0.000000000000000000 ) ) ;
#2631=ORIENTED_EDGE ( 'NONE', *, *, #37932, .F. ) ;
#2633=FACE_OUTER_BOUND ( 'NONE', #5660, .T. ) ;
#2638=DIRECTION ( 'NONE',  ( 1.000000000000000000, 0.000000000000000000, 0.000000000000000000 ) ) ;
#2639=EDGE_CURVE ( 'NONE', #8101, #11482, #365, .T. ) ;
#2643=EDGE_CURVE ( 'NONE', #22086, #35666, #13052, .T. ) ;
#2644=CARTESIAN_POINT ( 'NONE',  ( -8.118377661053488126, 10.47536095541708967, 11.00000000000000000 ) ) ;
#2645=ORIENTED_EDGE ( 'NONE', *, *, #20055, .F. ) ;
#2652=VERTEX_POINT ( 'NONE', #23005 ) ;
#2654=AXIS2_PLACEMENT_3D ( 'NONE', #22846, #3960, #13913 ) ;
#2659=CARTESIAN_POINT ( 'NONE',  ( 7.468455364333220103, 29.89744377950669474, 10.50000000000000000 ) ) ;
#2660=ORIENTED_EDGE ( 'NONE', *, *, #35085, .F. ) ;
#2663=ORIENTED_EDGE ( 'NONE', *, *, #28494, .F. ) ;
#2665=VECTOR ( 'NONE', #1579, 1000.000000000000114 ) ;
#2668=CYLINDRICAL_SURFACE ( 'NONE', #35774, 0.4999999999999995559 ) ;
#2672=EDGE_LOOP ( 'NONE', ( #35264, #9022, #13060, #29979 ) ) ;
#2674=PLANE ( 'NONE',  #26654 ) ;
#2677=LINE ( 'NONE', #19062, #36605 ) ;
#2680=CARTESIAN_POINT ( 'NONE',  ( 7.910872327081121647, 10.00199400870852529, 10.49999999999999467 ) ) ;
#2685=ORIENTED_EDGE ( 'NONE', *, *, #19102, .F. ) ;
#2689=EDGE_CURVE ( 'NONE', #4212, #21531, #12862, .T. ) ;
#2692=VERTEX_POINT ( 'NONE', #25255 ) ;
#2696=CARTESIAN_POINT ( 'NONE',  ( 14.86556419889027048, 20.43481210330100240, 10.49999999999999822 ) ) ;
#2697=VERTEX_POINT ( 'NONE', #38450 ) ;
#2698=EDGE_CURVE ( 'NONE', #35769, #32713, #19557, .T. ) ;
#2701=CARTESIAN_POINT ( 'NONE',  ( 14.01212783660239580, 27.85398076522207944, 7.455686640544908705 ) ) ;
#2704=CARTESIAN_POINT ( 'NONE',  ( 9.062230821157433169, 11.16111041642485802, 10.83333333333333037 ) ) ;
#2705=CARTESIAN_POINT ( 'NONE',  ( 7.014595103779618590, 35.79644522156321784, 10.49999999999999822 ) ) ;
#2708=ORIENTED_EDGE ( 'NONE', *, *, #34640, .F. ) ;
#2715=EDGE_CURVE ( 'NONE', #33392, #16160, #29997, .T. ) ;
#2718=CARTESIAN_POINT ( 'NONE',  ( 5.524694096546953759, 36.45979188825327100, 10.49999999999999822 ) ) ;
#2720=AXIS2_PLACEMENT_3D ( 'NONE', #9943, #37578, #31280 ) ;
#2721=CARTESIAN_POINT ( 'NONE',  ( 10.44103466624280507, 32.57396620494213124, 9.500000000000000000 ) ) ;
#2723=DIRECTION ( 'NONE',  ( -0.7622652262560031255, -0.2926062055178105248, 0.5773502691896430505 ) ) ;
#2727=DIRECTION ( 'NONE',  ( -0.000000000000000000, -0.000000000000000000, -1.000000000000000000 ) ) ;
#2732=ORIENTED_EDGE ( 'NONE', *, *, #37444, .F. ) ;
#2735=ADVANCED_FACE ( 'NONE', ( #31753 ), #22843, .T. ) ;
#2736=DIRECTION ( 'NONE',  ( -1.000000000000000000, 0.000000000000000000, 0.000000000000000000 ) ) ;
#2738=EDGE_LOOP ( 'NONE', ( #36414, #4286, #37880, #26014 ) ) ;
#2744=DIRECTION ( 'NONE',  ( 1.000000000000000000, -0.000000000000000000, 0.000000000000000000 ) ) ;
#2747=FACE_OUTER_BOUND ( 'NONE', #17861, .T. ) ;
#2751=DIRECTION ( 'NONE',  ( -0.000000000000000000, -0.000000000000000000, -1.000000000000000000 ) ) ;
#2754=CARTESIAN_POINT ( 'NONE',  ( -8.843266739736662885, 16.81698729810787540, 11.00000000000000000 ) ) ;
#2755=VERTEX_POINT ( 'NONE', #28698 ) ;
#2759=CARTESIAN_POINT ( 'NONE',  ( 13.95683075005237050, 28.08631143191933432, 11.00000000000000000 ) ) ;
#2763=CIRCLE ( 'NONE', #2110, 0.4999999999999997780 ) ;
#2765=ADVANCED_FACE ( 'NONE', ( #22801 ), #28903, .F. ) ;
#2767=CONICAL_SURFACE ( 'NONE', #20957, 0.5000000000000023315, 0.7853981633974499443 ) ;
#2768=DIRECTION ( 'NONE',  ( -0.6916548014802258448, -0.1470157664651941254, -0.7071067811865482389 ) ) ;
#2771=DIRECTION ( 'NONE',  ( -0.4156269377774565732, -0.5720614028176828070, -0.7071067811865469066 ) ) ;
#2772=CARTESIAN_POINT ( 'NONE',  ( 2.317734025672769427, 9.191051544684729180, 9.500000000000000000 ) ) ;
#2773=AXIS2_PLACEMENT_3D ( 'NONE', #11010, #4706, #29487 ) ;
#2774=CARTESIAN_POINT ( 'NONE',  ( -0.5000000000000000000, 37.00000000000000711, 9.500000000000000000 ) ) ;
#2775=CARTESIAN_POINT ( 'NONE',  ( -14.31603901957233482, 19.98981538725089990, 9.500000000000000000 ) ) ;
#2776=FACE_OUTER_BOUND ( 'NONE', #32903, .T. ) ;
#2777=DIRECTION ( 'NONE',  ( -0.9135454576426059736, -0.4067366430757888285, 0.000000000000000000 ) ) ;
#2779=DIRECTION ( 'NONE',  ( 0.1045284632676422437, -0.9945218953682746221, 0.000000000000000000 ) ) ;
#2780=ORIENTED_EDGE ( 'NONE', *, *, #34355, .F. ) ;
#2781=AXIS2_PLACEMENT_3D ( 'NONE', #8402, #36035, #17357 ) ;
#2783=CARTESIAN_POINT ( 'NONE',  ( 7.766013557953383106, 28.81973365084986938, 10.50000000000000178 ) ) ;
#2784=DIRECTION ( 'NONE',  ( 0.6724985119639518283, 0.2185080122244121292, -0.7071067811865521247 ) ) ;
#2788=B_SPLINE_CURVE_WITH_KNOTS ( 'NONE', 3,
 ( #36402, #24802, #21360, #17923, #21157, #33565 ),
 .UNSPECIFIED., .F., .F.,
 ( 4, 2, 4 ),
 ( 0.000000000000000000, 0.5000000000000000000, 1.000000000000000000 ),
 .UNSPECIFIED. ) ;
#2790=ORIENTED_EDGE ( 'NONE', *, *, #22755, .T. ) ;
#2800=ORIENTED_EDGE ( 'NONE', *, *, #14509, .F. ) ;
#2802=AXIS2_PLACEMENT_3D ( 'NONE', #24162, #27016, #11381 ) ;
#2804=ORIENTED_EDGE ( 'NONE', *, *, #31693, .F. ) ;
#2805=CARTESIAN_POINT ( 'NONE',  ( 2.368912364081567024, 7.688072489931943032, 7.455539900862791391 ) ) ;
#2807=CARTESIAN_POINT ( 'NONE',  ( 7.611215932167711529, 18.68301270189218855, 7.000000000000000000 ) ) ;
#2810=CONICAL_SURFACE ( 'NONE', #28755, 1.000000000000016431, 0.7853981633974533860 ) ;
#2812=ORIENTED_EDGE ( 'NONE', *, *, #3348, .T. ) ;
#2813=CARTESIAN_POINT ( 'NONE',  ( 8.100578861132808228, 28.44816123811117592, 10.50000000000000178 ) ) ;
#2816=FACE_OUTER_BOUND ( 'NONE', #1853, .T. ) ;
#2817=ADVANCED_FACE ( 'NONE', ( #19968 ), #20378, .T. ) ;
#2819=CARTESIAN_POINT ( 'NONE',  ( -13.94482798346716557, 26.50521816028930289, 11.00000000000000000 ) ) ;
#2824=DIRECTION ( 'NONE',  ( -1.000000000000000000, 0.000000000000000000, 0.000000000000000000 ) ) ;
#2825=EDGE_CURVE ( 'NONE', #751, #30937, #10533, .T. ) ;
#2826=DIRECTION ( 'NONE',  ( 0.000000000000000000, 0.000000000000000000, -1.000000000000000000 ) ) ;
#2831=ORIENTED_EDGE ( 'NONE', *, *, #14626, .F. ) ;
#2842=EDGE_CURVE ( 'NONE', #10050, #34846, #18968, .T. ) ;
#2843=CYLINDRICAL_SURFACE ( 'NONE', #34158, 0.5000000000000000000 ) ;
#2844=EDGE_CURVE ( 'NONE', #29799, #20155, #23814, .T. ) ;
#2845=ORIENTED_EDGE ( 'NONE', *, *, #210, .T. ) ;
#2848=CARTESIAN_POINT ( 'NONE',  ( 0.5000000000000002220, 37.50000000000000711, 10.49999999999999822 ) ) ;
#2850=VECTOR ( 'NONE', #7811, 999.9999999999998863 ) ;
#2851=LINE ( 'NONE', #15239, #17000 ) ;
#2852=EDGE_LOOP ( 'NONE', ( #28372, #25079, #12755, #29327 ) ) ;
#2854=CARTESIAN_POINT ( 'NONE',  ( -14.09933648065464062, 26.02968990214173317, 10.50000000000000533 ) ) ;
#2855=LINE ( 'NONE', #12791, #34246 ) ;
#2856=B_SPLINE_SURFACE_WITH_KNOTS ( 'NONE', 1, 3, ( 
 ( #24221, #18331, #12031, #33387, #39459, #8582, #20979, #18531, #30922, #37014 ),
 ( #2887, #33580, #21766, #17941, #3085, #30726, #15479, #12230, #30324, #15279 ) ),
 .UNSPECIFIED., .F., .F., .F.,
 ( 2, 2 ),
 ( 4, 2, 2, 2, 4 ),
 ( 0.000000000000000000, 1.000000000000000000 ),
 ( -1.421612811542164678, -1.028913729843439651, -0.6362146481447145119, -0.2435155664459894009, 0.1491835152527357100 ),
 .UNSPECIFIED. ) ;
#2857=VERTEX_POINT ( 'NONE', #14676 ) ;
#2859=CARTESIAN_POINT ( 'NONE',  ( -8.626760388790547296, 16.94198729810787185, 10.74999999999999822 ) ) ;
#2860=ORIENTED_EDGE ( 'NONE', *, *, #21555, .T. ) ;
#2862=CONICAL_SURFACE ( 'NONE', #16488, 0.4999999999999997780, 0.7853981633974524978 ) ;
#2866=DIRECTION ( 'NONE',  ( -0.000000000000000000, -0.000000000000000000, -1.000000000000000000 ) ) ;
#2867=EDGE_CURVE ( 'NONE', #21617, #5911, #11632, .T. ) ;
#2869=CIRCLE ( 'NONE', #22986, 1.000000000000004441 ) ;
#2871=ORIENTED_EDGE ( 'NONE', *, *, #2319, .F. ) ;
#2872=CARTESIAN_POINT ( 'NONE',  ( 3.987511920225066397, 8.280017797930394607, 10.49999999999999822 ) ) ;
#2874=CARTESIAN_POINT ( 'NONE',  ( 2.629601561899395534, 7.723830143584016206, 11.00000000000000000 ) ) ;
#2875=DIRECTION ( 'NONE',  ( -0.000000000000000000, 0.000000000000000000, -1.000000000000000000 ) ) ;
#2877=CARTESIAN_POINT ( 'NONE',  ( 5.400683141673458643, 15.91724817395916070, 9.000000000000001776 ) ) ;
#2879=CARTESIAN_POINT ( 'NONE',  ( 7.790810073469618402, 10.07556825234751408, 10.49999999999999822 ) ) ;
#2880=DIRECTION ( 'NONE',  ( -1.000000000000000000, 0.000000000000000000, 0.000000000000000000 ) ) ;
#2881=CARTESIAN_POINT ( 'NONE',  ( 13.87104230352200140, 20.53934056656866147, 10.00000000000000000 ) ) ;
#2882=CIRCLE ( 'NONE', #21701, 0.5000000000000004441 ) ;
#2887=CARTESIAN_POINT ( 'NONE',  ( -3.607749162633399731, 7.931741834401828228, 10.49999999999999645 ) ) ;
#2888=ORIENTED_EDGE ( 'NONE', *, *, #29011, .F. ) ;
#2889=ORIENTED_EDGE ( 'NONE', *, *, #34484, .F. ) ;
#2894=AXIS2_PLACEMENT_3D ( 'NONE', #28848, #38196, #3864 ) ;
#2895=ORIENTED_EDGE ( 'NONE', *, *, #10144, .F. ) ;
#2898=CARTESIAN_POINT ( 'NONE',  ( 2.317734025672765430, 9.191051544684729180, 10.50000000000000000 ) ) ;
#2899=ORIENTED_EDGE ( 'NONE', *, *, #16069, .F. ) ;
#2901=PLANE ( 'NONE',  #23894 ) ;
#2902=CARTESIAN_POINT ( 'NONE',  ( -10.52087624881762196, 22.14834255721595824, 10.74999999999998934 ) ) ;
#2905=EDGE_LOOP ( 'NONE', ( #38137, #14487, #10573, #9669 ) ) ;
#2909=VERTEX_POINT ( 'NONE', #26259 ) ;
#2911=DIRECTION ( 'NONE',  ( 0.6123724356957948034, 0.3535533905932776721, -0.7071067811865452413 ) ) ;
#2913=VECTOR ( 'NONE', #34711, 1000.000000000000114 ) ;
#2916=EDGE_CURVE ( 'NONE', #1914, #22045, #26091, .T. ) ;
#2917=DIRECTION ( 'NONE',  ( 0.5000000000000039968, 0.8660254037844363761, -0.000000000000000000 ) ) ;
#2920=ADVANCED_FACE ( 'NONE', ( #32569 ), #20172, .F. ) ;
#2923=ORIENTED_EDGE ( 'NONE', *, *, #30613, .F. ) ;
#2926=DIRECTION ( 'NONE',  ( 0.000000000000000000, 0.000000000000000000, 1.000000000000000000 ) ) ;
#2928=CARTESIAN_POINT ( 'NONE',  ( 5.440908595777814050, 35.94977745735560859, 9.000000000000001776 ) ) ;
#2935=VERTEX_POINT ( 'NONE', #30115 ) ;
#2936=DIRECTION ( 'NONE',  ( 0.8090169943749421222, -0.5877852522924804646, 0.000000000000000000 ) ) ;
#2937=ADVANCED_FACE ( 'NONE', ( #23618 ), #34340, .T. ) ;
#2938=EDGE_LOOP ( 'NONE', ( #31533, #39184, #15875, #24617 ) ) ;
#2940=DIRECTION ( 'NONE',  ( 0.3090169943749448977, -0.9510565162951543083, 0.000000000000000000 ) ) ;
#2941=ADVANCED_FACE ( 'NONE', ( #37208 ), #13777, .T. ) ;
#2944=EDGE_CURVE ( 'NONE', #39810, #17859, #36497, .T. ) ;
#2948=DIRECTION ( 'NONE',  ( 1.000000000000000000, 1.224646799147353947E-16, 0.000000000000000000 ) ) ;
#2952=CARTESIAN_POINT ( 'NONE',  ( 9.356056665764066693, 26.06569820189703179, 10.50000000000000000 ) ) ;
#2953=CARTESIAN_POINT ( 'NONE',  ( 6.914817619329722831, 35.81128241919675759, 7.381627713044574435 ) ) ;
#2954=DIRECTION ( 'NONE',  ( -0.2079116908177663092, -0.9781476007338041345, 0.000000000000000000 ) ) ;
#2955=CIRCLE ( 'NONE', #4250, 0.5000000000000002220 ) ;
#2956=ORIENTED_EDGE ( 'NONE', *, *, #14335, .T. ) ;
#2961=CARTESIAN_POINT ( 'NONE',  ( -7.096882951594430722, 29.56287847632736288, 10.49999999999999822 ) ) ;
#2966=DIRECTION ( 'NONE',  ( -0.9135454576426005335, 0.4067366430758009299, -0.000000000000000000 ) ) ;
#2967=ADVANCED_FACE ( 'NONE', ( #39846 ), #32, .T. ) ;
#2970=CARTESIAN_POINT ( 'NONE',  ( 3.399837471815457590, 8.909889435135580626, 7.000000000000000000 ) ) ;
#2971=CARTESIAN_POINT ( 'NONE',  ( 13.05736835487433289, 16.11602540378438420, 10.50000000000000178 ) ) ;
#2973=DIRECTION ( 'NONE',  ( 0.6691306063588671194, 0.7431448254773861395, 0.000000000000000000 ) ) ;
#2974=CARTESIAN_POINT ( 'NONE',  ( 14.66655470856244037, 20.08105443166835258, 10.49999999999999822 ) ) ;
#2978=FACE_OUTER_BOUND ( 'NONE', #5641, .T. ) ;
#2981=DIRECTION ( 'NONE',  ( 0.000000000000000000, 0.000000000000000000, -1.000000000000000000 ) ) ;
#2982=CONICAL_SURFACE ( 'NONE', #23746, 1.000000000000007772, 0.7853981633974560506 ) ;
#2985=LINE ( 'NONE', #25112, #36943 ) ;
#2986=VECTOR ( 'NONE', #18239, 1000.000000000000000 ) ;
#2993=VERTEX_POINT ( 'NONE', #2487 ) ;
#2994=DIRECTION ( 'NONE',  ( -0.000000000000000000, -0.000000000000000000, -1.000000000000000000 ) ) ;
#3009=AXIS2_PLACEMENT_3D ( 'NONE', #40006, #27824, #11788 ) ;
#3012=AXIS2_PLACEMENT_3D ( 'NONE', #23878, #35677, #39314 ) ;
#3014=ORIENTED_EDGE ( 'NONE', *, *, #2091, .F. ) ;
#3015=DIRECTION ( 'NONE',  ( -0.000000000000000000, -0.000000000000000000, -1.000000000000000000 ) ) ;
#3016=ORIENTED_EDGE ( 'NONE', *, *, #22058, .T. ) ;
#3017=LINE ( 'NONE', #14810, #33336 ) ;
#3018=DIRECTION ( 'NONE',  ( 1.000000000000000000, 0.000000000000000000, 0.000000000000000000 ) ) ;
#3019=DIRECTION ( 'NONE',  ( -0.7431448254773862505, 0.6691306063588672304, -0.000000000000000000 ) ) ;
#3020=ORIENTED_EDGE ( 'NONE', *, *, #11811, .T. ) ;
#3022=CARTESIAN_POINT ( 'NONE',  ( -5.440908595777639079, 35.94977745735568675, 11.00000000000000000 ) ) ;
#3023=CARTESIAN_POINT ( 'NONE',  ( -9.331903152615899089, 11.35703883385581037, 9.500000000000000000 ) ) ;
#3024=FACE_OUTER_BOUND ( 'NONE', #8809, .T. ) ;
#3028=EDGE_LOOP ( 'NONE', ( #38755, #36747, #4844, #7937 ) ) ;
#3032=DIRECTION ( 'NONE',  ( 0.1045284632676422437, -0.9945218953682746221, 0.000000000000000000 ) ) ;
#3035=AXIS2_PLACEMENT_3D ( 'NONE', #2562, #14545, #36686 ) ;
#3041=CARTESIAN_POINT ( 'NONE',  ( 11.47910261372047636, 31.49019768869741753, 10.49999999999999822 ) ) ;
#3045=DIRECTION ( 'NONE',  ( -0.6691306063588570163, 0.7431448254773952433, 0.000000000000000000 ) ) ;
#3046=CARTESIAN_POINT ( 'NONE',  ( -9.296885549838707519, 10.71356306745948217, 10.49999999999999822 ) ) ;
#3047=ORIENTED_EDGE ( 'NONE', *, *, #16636, .T. ) ;
#3049=ADVANCED_FACE ( 'NONE', ( #18322 ), #18365, .T. ) ;
#3053=ORIENTED_EDGE ( 'NONE', *, *, #36357, .F. ) ;
#3055=CARTESIAN_POINT ( 'NONE',  ( 8.927394655428274817, 11.06314620770945290, 7.500000000000000888 ) ) ;
#3058=ORIENTED_EDGE ( 'NONE', *, *, #20232, .F. ) ;
#3061=DIRECTION ( 'NONE',  ( -0.4999999999999920064, 0.8660254037844432595, 0.000000000000000000 ) ) ;
#3063=AXIS2_PLACEMENT_3D ( 'NONE', #17957, #34184, #40067 ) ;
#3064=VECTOR ( 'NONE', #29426, 1000.000000000000000 ) ;
#3066=ORIENTED_EDGE ( 'NONE', *, *, #593, .T. ) ;
#3069=EDGE_CURVE ( 'NONE', #3204, #802, #39650, .T. ) ;
#3070=DIRECTION ( 'NONE',  ( 1.000000000000000000, 0.000000000000000000, 0.000000000000000000 ) ) ;
#3071=EDGE_CURVE ( 'NONE', #25412, #38194, #24810, .T. ) ;
#3072=VECTOR ( 'NONE', #12547, 1000.000000000000114 ) ;
#3073=CARTESIAN_POINT ( 'NONE',  ( 13.63581098909226519, 27.45627467658428600, 7.000000000000000000 ) ) ;
#3074=VECTOR ( 'NONE', #35458, 1000.000000000000114 ) ;
#3076=DIRECTION ( 'NONE',  ( -0.000000000000000000, -0.000000000000000000, 1.000000000000000000 ) ) ;
#3078=FACE_OUTER_BOUND ( 'NONE', #33550, .T. ) ;
#3079=DIRECTION ( 'NONE',  ( 1.000000000000000000, 0.000000000000000000, 0.000000000000000000 ) ) ;
#3080=CARTESIAN_POINT ( 'NONE',  ( 0.6108529249775871417, 37.48755679569043053, 7.500000000000000888 ) ) ;
#3081=ORIENTED_EDGE ( 'NONE', *, *, #21958, .F. ) ;
#3085=CARTESIAN_POINT ( 'NONE',  ( -3.574287532905768394, 8.089166425130688509, 10.87262190629277470 ) ) ;
#3086=EDGE_LOOP ( 'NONE', ( #11914, #38778, #23491 ) ) ;
#3087=ORIENTED_EDGE ( 'NONE', *, *, #18215, .T. ) ;
#3090=EDGE_CURVE ( 'NONE', #6733, #17177, #24615, .T. ) ;
#3092=VECTOR ( 'NONE', #32291, 1000.000000000000000 ) ;
#3094=ORIENTED_EDGE ( 'NONE', *, *, #38872, .T. ) ;
#3100=DIRECTION ( 'NONE',  ( -0.000000000000000000, -0.000000000000000000, -1.000000000000000000 ) ) ;
#3101=DIRECTION ( 'NONE',  ( -0.9945218953682740670, -0.1045284632676460046, 6.938893903907226800E-15 ) ) ;
#3105=ORIENTED_EDGE ( 'NONE', *, *, #4020, .F. ) ;
#3112=CARTESIAN_POINT ( 'NONE',  ( -14.49226701858006727, 26.37020042452770596, 7.438752290525425082 ) ) ;
#3114=DIRECTION ( 'NONE',  ( -0.8660254037844431485, -0.4999999999999921729, 0.000000000000000000 ) ) ;
#3115=DIRECTION ( 'NONE',  ( -0.9781476007338042455, 0.2079116908177664480, 0.000000000000000000 ) ) ;
#3116=EDGE_CURVE ( 'NONE', #36749, #20981, #14877, .T. ) ;
#3117=AXIS2_PLACEMENT_3D ( 'NONE', #23943, #17260, #7895 ) ;
#3118=CIRCLE ( 'NONE', #1181, 0.5000000000000004441 ) ;
#3120=CARTESIAN_POINT ( 'NONE',  ( -4.908204406342476567, 36.67476118479555680, 7.102474990965863100 ) ) ;
#3122=CARTESIAN_POINT ( 'NONE',  ( 10.10646936306337729, 32.94553861768082470, 10.49999999999999822 ) ) ;
#3125=CIRCLE ( 'NONE', #8325, 0.5000000000000004441 ) ;
#3126=LINE ( 'NONE', #36660, #34547 ) ;
#3128=VERTEX_POINT ( 'NONE', #36807 ) ;
#3133=ORIENTED_EDGE ( 'NONE', *, *, #4115, .F. ) ;
#3135=ORIENTED_EDGE ( 'NONE', *, *, #33825, .F. ) ;
#3137=LINE ( 'NONE', #30584, #28955 ) ;
#3140=DIRECTION ( 'NONE',  ( -0.8660254037844431485, -0.4999999999999921174, 0.000000000000000000 ) ) ;
#3144=LINE ( 'NONE', #27924, #11195 ) ;
#3146=EDGE_LOOP ( 'NONE', ( #766, #12726, #19900 ) ) ;
#3147=EDGE_CURVE ( 'NONE', #28465, #13430, #9177, .T. ) ;
#3149=CARTESIAN_POINT ( 'NONE',  ( -2.317734025672944842, 9.191051544684764707, 9.500000000000000000 ) ) ;
#3150=ADVANCED_FACE ( 'NONE', ( #6119 ), #24828, .T. ) ;
#3151=CARTESIAN_POINT ( 'NONE',  ( 10.81260707898150386, 32.90853150812155548, 10.49999999999999822 ) ) ;
#3153=ORIENTED_EDGE ( 'NONE', *, *, #22580, .F. ) ;
#3155=AXIS2_PLACEMENT_3D ( 'NONE', #35519, #19669, #14180 ) ;
#3157=CIRCLE ( 'NONE', #1886, 0.9999999999999974465 ) ;
#3159=CARTESIAN_POINT ( 'NONE',  ( -5.092030333742499693, 36.31140934042896617, 10.49999999999999822 ) ) ;
#3161=ORIENTED_EDGE ( 'NONE', *, *, #35362, .F. ) ;
#3162=VECTOR ( 'NONE', #14714, 1000.000000000000000 ) ;
#3164=DIRECTION ( 'NONE',  ( 1.000000000000000000, 0.000000000000000000, 0.000000000000000000 ) ) ;
#3168=EDGE_CURVE ( 'NONE', #2652, #10797, #32654, .T. ) ;
#3169=EDGE_CURVE ( 'NONE', #18534, #39411, #33263, .T. ) ;
#3171=CARTESIAN_POINT ( 'NONE',  ( 12.80736835487432934, 15.68301270189215835, 11.00000000000000000 ) ) ;
#3174=DIRECTION ( 'NONE',  ( -0.000000000000000000, -0.000000000000000000, 1.000000000000000000 ) ) ;
#3175=CARTESIAN_POINT ( 'NONE',  ( -10.44103466624267362, 32.57396620494226624, 9.500000000000000000 ) ) ;
#3176=DIRECTION ( 'NONE',  ( -0.4999999999999920064, 0.8660254037844432595, -0.000000000000000000 ) ) ;
#3177=LINE ( 'NONE', #30617, #16414 ) ;
#3178=CARTESIAN_POINT ( 'NONE',  ( -2.256323172317921788, 14.28970123917155277, 9.000000000000001776 ) ) ;
#3181=AXIS2_PLACEMENT_3D ( 'NONE', #2783, #24712, #37112 ) ;
#3184=CARTESIAN_POINT ( 'NONE',  ( 12.30736835487432934, 14.81698729810772797, 11.00000000000000000 ) ) ;
#3190=PRODUCT ( 'Dual-Edge Stainless Steel Rotary Blade', 'Dual-Edge Stainless Steel Rotary Blade', '', ( #10158 ) ) ;
#3192=CARTESIAN_POINT ( 'NONE',  ( -3.503793317224517700, 8.420815634768727520, 7.000000000000000000 ) ) ;
#3194=ADVANCED_FACE ( 'NONE', ( #18408 ), #33464, .T. ) ;
#3200=EDGE_CURVE ( 'NONE', #40105, #37972, #26479, .T. ) ;
#3202=CARTESIAN_POINT ( 'NONE',  ( 9.892954722048896699, 20.95745441963929423, 10.50000000000000533 ) ) ;
#3204=VERTEX_POINT ( 'NONE', #33998 ) ;
#3208=ORIENTED_EDGE ( 'NONE', *, *, #11173, .T. ) ;
#3209=DIRECTION ( 'NONE',  ( 0.5000000000000038858, 0.8660254037844363761, -0.000000000000000000 ) ) ;
#3210=CYLINDRICAL_SURFACE ( 'NONE', #21939, 0.5000000000000002220 ) ;
#3213=ORIENTED_EDGE ( 'NONE', *, *, #35941, .F. ) ;
#3214=LINE ( 'NONE', #15006, #29724 ) ;
#3215=ORIENTED_EDGE ( 'NONE', *, *, #25268, .F. ) ;
#3217=FACE_OUTER_BOUND ( 'NONE', #14654, .T. ) ;
#3219=EDGE_CURVE ( 'NONE', #24567, #35217, #30355, .T. ) ;
#3221=ORIENTED_EDGE ( 'NONE', *, *, #14900, .F. ) ;
#3224=LINE ( 'NONE', #37747, #33206 ) ;
#3226=LINE ( 'NONE', #15615, #15655 ) ;
#3229=EDGE_LOOP ( 'NONE', ( #22499, #24075, #23450 ) ) ;
#3233=CARTESIAN_POINT ( 'NONE',  ( 12.62284334487383397, 42.89764170712515323, 9.500000000000000000 ) ) ;
#3236=CARTESIAN_POINT ( 'NONE',  ( -10.10646936306323518, 32.94553861768095970, 10.49999999999999822 ) ) ;
#3238=AXIS2_PLACEMENT_3D ( 'NONE', #10375, #27700, #19716 ) ;
#3242=EDGE_CURVE ( 'NONE', #7627, #12011, #36253, .T. ) ;
#3244=CARTESIAN_POINT ( 'NONE',  ( 5.632984386902417206, 36.38118674759823534, 10.68306085400105587 ) ) ;
#3248=CARTESIAN_POINT ( 'NONE',  ( -14.85188145504476687, 20.30462949162108544, 10.49999999999999822 ) ) ;
#3249=CARTESIAN_POINT ( 'NONE',  ( 8.633502029282041690, 11.46765470489692795, 7.500000000000000888 ) ) ;
#3250=CARTESIAN_POINT ( 'NONE',  ( 11.62435565298210882, 14.63397459621550922, 10.50000000000000000 ) ) ;
#3251=EDGE_LOOP ( 'NONE', ( #15723, #19590, #5631, #7044 ) ) ;
#3253=CARTESIAN_POINT ( 'NONE',  ( 11.77929587896052155, 31.08767655398733254, 7.000000000000000000 ) ) ;
#3254=LINE ( 'NONE', #28033, #7645 ) ;
#3258=ORIENTED_EDGE ( 'NONE', *, *, #944, .T. ) ;
#3260=VERTEX_POINT ( 'NONE', #14712 ) ;
#3262=LINE ( 'NONE', #34348, #39780 ) ;
#3263=DIRECTION ( 'NONE',  ( 1.000000000000000000, 0.000000000000000000, 0.000000000000000000 ) ) ;
#3265=CARTESIAN_POINT ( 'NONE',  ( 5.440908595777819379, 35.94977745735560859, 11.00000000000000000 ) ) ;
#3266=ORIENTED_EDGE ( 'NONE', *, *, #34375, .F. ) ;
#3267=CARTESIAN_POINT ( 'NONE',  ( 0.000000000000000000, 22.50000000000000355, 7.000000000000000000 ) ) ;
#3270=CARTESIAN_POINT ( 'NONE',  ( 12.67417846324118358, 14.47720745114811436, 7.499999999999997335 ) ) ;
#3274=EDGE_CURVE ( 'NONE', #30348, #6928, #15106, .T. ) ;
#3277=CYLINDRICAL_SURFACE ( 'NONE', #19321, 6.000000000000003553 ) ;
#3280=AXIS2_PLACEMENT_3D ( 'NONE', #25842, #3512, #37644 ) ;
#3290=VERTEX_POINT ( 'NONE', #18358 ) ;
#3293=CARTESIAN_POINT ( 'NONE',  ( 13.81820544359399427, 28.33708565239886212, 7.102637441331454582 ) ) ;
#3294=VERTEX_POINT ( 'NONE', #2124 ) ;
#3298=ADVANCED_FACE ( 'NONE', ( #9211 ), #27690, .F. ) ;
#3300=ORIENTED_EDGE ( 'NONE', *, *, #38411, .F. ) ;
#3308=CARTESIAN_POINT ( 'NONE',  ( -14.47475276859717219, 26.43532618598166906, 7.470075214869918767 ) ) ;
#3309=CARTESIAN_POINT ( 'NONE',  ( -13.49038105676663868, 15.86602540378456361, 10.49999999999999822 ) ) ;
#3310=DIRECTION ( 'NONE',  ( 1.000000000000000000, 0.000000000000000000, 0.000000000000000000 ) ) ;
#3311=VECTOR ( 'NONE', #22188, 1000.000000000000000 ) ;
#3312=ADVANCED_FACE ( 'NONE', ( #39286 ), #27493, .F. ) ;
#3313=DIRECTION ( 'NONE',  ( 0.5877852522924796874, 0.8090169943749426773, 0.000000000000000000 ) ) ;
#3315=CARTESIAN_POINT ( 'NONE',  ( -11.54666566735211752, 32.07468077621347646, 7.500000000000004441 ) ) ;
#3316=EDGE_CURVE ( 'NONE', #7248, #23537, #33415, .T. ) ;
#3321=DIRECTION ( 'NONE',  ( -0.3090169943749457304, 0.9510565162951540863, 0.000000000000000000 ) ) ;
#3323=AXIS2_PLACEMENT_3D ( 'NONE', #13559, #4218, #19252 ) ;
#3324=FACE_OUTER_BOUND ( 'NONE', #17500, .T. ) ;
#3329=CARTESIAN_POINT ( 'NONE',  ( -0.5000000000000004441, 33.00000000000000000, 10.00000000000000000 ) ) ;
#3331=ORIENTED_EDGE ( 'NONE', *, *, #20332, .T. ) ;
#3333=ORIENTED_EDGE ( 'NONE', *, *, #32867, .F. ) ;
#3335=DIRECTION ( 'NONE',  ( -1.000000000000000000, 0.000000000000000000, 0.000000000000000000 ) ) ;
#3345=AXIS2_PLACEMENT_3D ( 'NONE', #22944, #32300, #38189 ) ;
#3346=DIRECTION ( 'NONE',  ( 0.000000000000000000, 0.000000000000000000, 1.000000000000000000 ) ) ;
#3347=EDGE_CURVE ( 'NONE', #42, #35381, #31292, .T. ) ;
#3348=EDGE_CURVE ( 'NONE', #3653, #11472, #24447, .T. ) ;
#3349=CARTESIAN_POINT ( 'NONE',  ( -9.363324537585851814, 32.27640801132209702, 10.50000000000000000 ) ) ;
#3350=EDGE_LOOP ( 'NONE', ( #14030, #15005, #33607, #23429 ) ) ;
#3354=ORIENTED_EDGE ( 'NONE', *, *, #31722, .F. ) ;
#3357=CYLINDRICAL_SURFACE ( 'NONE', #22545, 0.5000000000000004441 ) ;
#3358=ORIENTED_EDGE ( 'NONE', *, *, #16307, .T. ) ;
#3359=LINE ( 'NONE', #15557, #917 ) ;
#3362=FACE_OUTER_BOUND ( 'NONE', #18698, .T. ) ;
#3367=DIRECTION ( 'NONE',  ( 0.000000000000000000, -0.000000000000000000, 1.000000000000000000 ) ) ;
#3368=CARTESIAN_POINT ( 'NONE',  ( 7.014595103779618590, 35.79644522156321784, 11.00000000000000000 ) ) ;
#3371=DIRECTION ( 'NONE',  ( -0.9510565162951504226, 0.3090169943749573322, 0.000000000000000000 ) ) ;
#3373=CARTESIAN_POINT ( 'NONE',  ( 13.30736791475921699, 15.68301270237638967, 10.49999999999999822 ) ) ;
#3374=ORIENTED_EDGE ( 'NONE', *, *, #24516, .F. ) ;
#3377=CARTESIAN_POINT ( 'NONE',  ( 13.20348688925205316, 15.99217894729783929, 10.49999999999999822 ) ) ;
#3378=AXIS2_PLACEMENT_3D ( 'NONE', #30403, #18012, #40124 ) ;
#3387=CIRCLE ( 'NONE', #9278, 1.000000000000000444 ) ;
#3392=CARTESIAN_POINT ( 'NONE',  ( 11.54200800595913456, 31.54683795827724424, 10.49999999999999822 ) ) ;
#3395=EDGE_CURVE ( 'NONE', #31091, #11163, #21401, .T. ) ;
#3399=CARTESIAN_POINT ( 'NONE',  ( 2.441045247299091336, 7.699747138389255063, 7.485699520496970294 ) ) ;
#3404=ORIENTED_EDGE ( 'NONE', *, *, #16213, .F. ) ;
#3405=CONICAL_SURFACE ( 'NONE', #18355, 0.4999999999999961142, 0.7853981633974473908 ) ;
#3406=FACE_OUTER_BOUND ( 'NONE', #29927, .T. ) ;
#3407=EDGE_LOOP ( 'NONE', ( #26062, #32980, #28248, #27448 ) ) ;
#3408=CYLINDRICAL_SURFACE ( 'NONE', #27489, 6.000000000000010658 ) ;
#3409=DIRECTION ( 'NONE',  ( -1.000000000000000000, 0.000000000000000000, 0.000000000000000000 ) ) ;
#3410=ADVANCED_FACE ( 'NONE', ( #863 ), #12452, .F. ) ;
#3411=AXIS2_PLACEMENT_3D ( 'NONE', #22976, #22368, #31323 ) ;
#3413=EDGE_LOOP ( 'NONE', ( #16065, #8742, #17773, #425 ) ) ;
#3414=EDGE_CURVE ( 'NONE', #9720, #37780, #26131, .T. ) ;
#3417=DIRECTION ( 'NONE',  ( -0.4156269377774573504, -0.5720614028176800314, -0.7071067811865487940 ) ) ;
#3418=DIRECTION ( 'NONE',  ( -0.000000000000000000, -0.000000000000000000, -1.000000000000000000 ) ) ;
#3423=EDGE_CURVE ( 'NONE', #8840, #36419, #20204, .T. ) ;
#3427=CARTESIAN_POINT ( 'NONE',  ( 15.00099999999999945, 32.50000000000000000, 10.00000000000000000 ) ) ;
#3430=DIRECTION ( 'NONE',  ( 0.7431448254773953543, 0.6691306063588570163, -0.000000000000000000 ) ) ;
#3436=VECTOR ( 'NONE', #12673, 1000.000000000000000 ) ;
#3437=CARTESIAN_POINT ( 'NONE',  ( 8.317671217785902016, 10.20105690706387591, 10.87262190629280489 ) ) ;
#3442=DIRECTION ( 'NONE',  ( 0.1470157664651934593, -0.6916548014802230693, -0.7071067811865510144 ) ) ;
#3447=EDGE_LOOP ( 'NONE', ( #937, #35537, #39151, #28477 ) ) ;
#3449=CARTESIAN_POINT ( 'NONE',  ( 14.58225150643707835, 26.01772713467079612, 7.202682876670051471 ) ) ;
#3450=CARTESIAN_POINT ( 'NONE',  ( -5.440908595777636414, 35.94977745735568675, 7.000000000000000000 ) ) ;
#3451=VERTEX_POINT ( 'NONE', #6941 ) ;
#3454=VECTOR ( 'NONE', #9475, 1000.000000000000114 ) ;
#3457=VECTOR ( 'NONE', #37884, 1000.000000000000000 ) ;
#3461=DIRECTION ( 'NONE',  ( 1.000000000000000000, 0.000000000000000000, -0.000000000000000000 ) ) ;
#3462=EDGE_CURVE ( 'NONE', #16093, #27294, #30947, .T. ) ;
#3464=CIRCLE ( 'NONE', #4098, 0.5000000000000000000 ) ;
#3465=DIRECTION ( 'NONE',  ( 1.000000000000000000, 0.000000000000000000, 0.000000000000000000 ) ) ;
#3467=EDGE_CURVE ( 'NONE', #18499, #8101, #28942, .T. ) ;
#3468=CARTESIAN_POINT ( 'NONE',  ( 3.523049899833284648, 8.330220536420911870, 10.99387789255784220 ) ) ;
#3471=LINE ( 'NONE', #6703, #38331 ) ;
#3477=LINE ( 'NONE', #3675, #20655 ) ;
#3478=ORIENTED_EDGE ( 'NONE', *, *, #25524, .T. ) ;
#3483=CARTESIAN_POINT ( 'NONE',  ( -6.151085731882352192, 35.08626808545859888, 9.500000000000000000 ) ) ;
#3484=ORIENTED_EDGE ( 'NONE', *, *, #36732, .T. ) ;
#3485=ORIENTED_EDGE ( 'NONE', *, *, #35941, .T. ) ;
#3494=ORIENTED_EDGE ( 'NONE', *, *, #25374, .F. ) ;
#3496=CARTESIAN_POINT ( 'NONE',  ( -14.31603901957233660, 19.98981538725089990, 7.000000000000000000 ) ) ;
#3501=VERTEX_POINT ( 'NONE', #25633 ) ;
#3508=CARTESIAN_POINT ( 'NONE',  ( -14.58494835919645993, 26.00628811930699413, 7.192820069705969210 ) ) ;
#3510=AXIS2_PLACEMENT_3D ( 'NONE', #20574, #32969, #2281 ) ;
#3512=DIRECTION ( 'NONE',  ( 0.000000000000000000, 0.000000000000000000, 1.000000000000000000 ) ) ;
#3514=AXIS2_PLACEMENT_3D ( 'NONE', #35158, #1237, #35364 ) ;
#3516=DIRECTION ( 'NONE',  ( -0.000000000000000000, -0.000000000000000000, -1.000000000000000000 ) ) ;
#3518=FACE_OUTER_BOUND ( 'NONE', #37865, .T. ) ;
#3520=CARTESIAN_POINT ( 'NONE',  ( 1.547498115756713588, 8.004992253133169200, 7.000000000000000000 ) ) ;
#3530=ORIENTED_EDGE ( 'NONE', *, *, #33606, .F. ) ;
#3532=LINE ( 'NONE', #6182, #24406 ) ;
#3538=CARTESIAN_POINT ( 'NONE',  ( -8.505700342264141511, 22.10876900990917804, 7.000000000000000000 ) ) ;
#3540=ORIENTED_EDGE ( 'NONE', *, *, #2825, .F. ) ;
#3542=EDGE_CURVE ( 'NONE', #34288, #2054, #34996, .T. ) ;
#3543=LINE ( 'NONE', #9246, #21905 ) ;
#3546=ORIENTED_EDGE ( 'NONE', *, *, #1183, .T. ) ;
#3548=CONICAL_SURFACE ( 'NONE', #31446, 0.4999999999999997780, 0.7853981633974511656 ) ;
#3550=EDGE_CURVE ( 'NONE', #31065, #4676, #34394, .T. ) ;
#3552=ORIENTED_EDGE ( 'NONE', *, *, #16350, .F. ) ;
#3554=AXIS2_PLACEMENT_3D ( 'NONE', #28350, #31207, #25109 ) ;
#3556=DIRECTION ( 'NONE',  ( 1.000000000000000000, 0.000000000000000000, 0.000000000000000000 ) ) ;
#3557=VECTOR ( 'NONE', #10312, 1000.000000000000114 ) ;
#3559=CARTESIAN_POINT ( 'NONE',  ( -7.611215932167763043, 18.68301270189229513, 9.000000000000001776 ) ) ;
#3560=CARTESIAN_POINT ( 'NONE',  ( -11.14453731054088514, 31.86177010143615007, 11.00000000000000000 ) ) ;
#3561=CARTESIAN_POINT ( 'NONE',  ( 14.96930490892014731, 21.54088032874976832, 7.000000000000000000 ) ) ;
#3564=EDGE_CURVE ( 'NONE', #25343, #26836, #31339, .T. ) ;
#3565=PLANE ( 'NONE',  #14979 ) ;
#3566=EDGE_CURVE ( 'NONE', #2935, #11482, #34195, .T. ) ;
#3570=FACE_OUTER_BOUND ( 'NONE', #7499, .T. ) ;
#3573=DIRECTION ( 'NONE',  ( 0.2079116908177533751, -0.9781476007338069101, 0.000000000000000000 ) ) ;
#3576=LINE ( 'NONE', #8882, #31744 ) ;
#3577=LINE ( 'NONE', #37510, #24409 ) ;
#3583=AXIS2_PLACEMENT_3D ( 'NONE', #28961, #3775, #736 ) ;
#3584=CARTESIAN_POINT ( 'NONE',  ( 13.05736835487433289, 16.11602540378438420, 7.499999999999997335 ) ) ;
#3587=VECTOR ( 'NONE', #19397, 999.9999999999998863 ) ;
#3598=EDGE_CURVE ( 'NONE', #36223, #5248, #34588, .T. ) ;
#3600=VERTEX_POINT ( 'NONE', #16103 ) ;
#3601=DIRECTION ( 'NONE',  ( 0.000000000000000000, 0.000000000000000000, 1.000000000000000000 ) ) ;
#3607=ORIENTED_EDGE ( 'NONE', *, *, #12440, .T. ) ;
#3609=AXIS2_PLACEMENT_3D ( 'NONE', #18185, #34412, #28506 ) ;
#3611=VECTOR ( 'NONE', #27554, 999.9999999999998863 ) ;
#3612=CIRCLE ( 'NONE', #39951, 0.5000000000000004441 ) ;
#3613=DIRECTION ( 'NONE',  ( 0.9510565162951543083, 0.3090169943749450088, -0.000000000000000000 ) ) ;
#3614=VERTEX_POINT ( 'NONE', #22382 ) ;
#3616=DIRECTION ( 'NONE',  ( 0.000000000000000000, 0.000000000000000000, 1.000000000000000000 ) ) ;
#3618=EDGE_CURVE ( 'NONE', #29941, #18778, #13042, .T. ) ;
#3620=CARTESIAN_POINT ( 'NONE',  ( 14.36830325120613594, 20.48707633493483371, 7.500000000000010658 ) ) ;
#3621=LINE ( 'NONE', #16016, #879 ) ;
#3623=ORIENTED_EDGE ( 'NONE', *, *, #31240, .F. ) ;
#3627=PLANE ( 'NONE',  #17221 ) ;
#3630=FACE_OUTER_BOUND ( 'NONE', #10587, .T. ) ;
#3635=LINE ( 'NONE', #9939, #36136 ) ;
#3640=EDGE_CURVE ( 'NONE', #29758, #32296, #10003, .T. ) ;
#3641=DIRECTION ( 'NONE',  ( -0.000000000000000000, -0.000000000000000000, -1.000000000000000000 ) ) ;
#3643=CARTESIAN_POINT ( 'NONE',  ( 0.000000000000000000, 22.50000000000000355, 7.000000000000000000 ) ) ;
#3646=ADVANCED_FACE ( 'NONE', ( #16711 ), #33172, .T. ) ;
#3648=VECTOR ( 'NONE', #29010, 1000.000000000000000 ) ;
#3649=CARTESIAN_POINT ( 'NONE',  ( 13.13581098909226696, 27.45627467658428955, 7.000000000000000000 ) ) ;
#3653=VERTEX_POINT ( 'NONE', #1879 ) ;
#3656=ORIENTED_EDGE ( 'NONE', *, *, #6896, .F. ) ;
#3658=CARTESIAN_POINT ( 'NONE',  ( 10.73859285986296541, 31.49625607628530588, 7.499999999999996447 ) ) ;
#3661=DIRECTION ( 'NONE',  ( -1.000000000000000000, 0.000000000000000000, 0.000000000000000000 ) ) ;
#3662=ORIENTED_EDGE ( 'NONE', *, *, #3423, .T. ) ;
#3663=FACE_OUTER_BOUND ( 'NONE', #34352, .T. ) ;
#3665=DIRECTION ( 'NONE',  ( 1.000000000000000000, 0.000000000000000000, 0.000000000000000000 ) ) ;
#3666=EDGE_CURVE ( 'NONE', #36832, #9748, #30594, .T. ) ;
#3667=EDGE_CURVE ( 'NONE', #34816, #23702, #26244, .T. ) ;
#3672=CIRCLE ( 'NONE', #12114, 1.000000000000008660 ) ;
#3675=CARTESIAN_POINT ( 'NONE',  ( 4.591666147298500533, 15.32946292166668556, 9.000000000000001776 ) ) ;
#3676=ORIENTED_EDGE ( 'NONE', *, *, #9427, .T. ) ;
#3681=ORIENTED_EDGE ( 'NONE', *, *, #6738, .T. ) ;
#3682=ORIENTED_EDGE ( 'NONE', *, *, #11565, .T. ) ;
#3685=ADVANCED_FACE ( 'NONE', ( #10611 ), #22992, .T. ) ;
#3689=CARTESIAN_POINT ( 'NONE',  ( 2.421689871081641687, 8.701977744317826335, 7.499999999999991118 ) ) ;
#3692=EDGE_CURVE ( 'NONE', #28502, #6243, #37076, .T. ) ;
#3693=CARTESIAN_POINT ( 'NONE',  ( 0.000000000000000000, 22.50000000000000355, 7.000000000000000000 ) ) ;
#3695=ORIENTED_EDGE ( 'NONE', *, *, #16640, .T. ) ;
#3697=EDGE_LOOP ( 'NONE', ( #33973, #7904, #9994, #33355 ) ) ;
#3700=VECTOR ( 'NONE', #36527, 1000.000000000000000 ) ;
#3701=CARTESIAN_POINT ( 'NONE',  ( -11.54666566735214772, 32.07468077621344094, 7.000000000000000000 ) ) ;
#3704=DIRECTION ( 'NONE',  ( -0.000000000000000000, -0.000000000000000000, -1.000000000000000000 ) ) ;
#3706=AXIS2_PLACEMENT_3D ( 'NONE', #24506, #30616, #6601 ) ;
#3707=DIRECTION ( 'NONE',  ( 0.9510565162951503115, -0.3090169943749574988, 0.000000000000000000 ) ) ;
#3708=DIRECTION ( 'NONE',  ( 0.8090169943749426773, -0.5877852522924797984, -0.000000000000000000 ) ) ;
#3716=ORIENTED_EDGE ( 'NONE', *, *, #31912, .F. ) ;
#3722=EDGE_LOOP ( 'NONE', ( #3530, #35691, #702, #21001, #24401 ) ) ;
#3725=AXIS2_PLACEMENT_3D ( 'NONE', #5165, #36255, #39287 ) ;
#3727=CYLINDRICAL_SURFACE ( 'NONE', #28337, 0.5000000000000004441 ) ;
#3746=AXIS2_PLACEMENT_3D ( 'NONE', #38003, #7725, #1035 ) ;
#3748=DIRECTION ( 'NONE',  ( 1.000000000000000000, 0.000000000000000000, 0.000000000000000000 ) ) ;
#3749=CIRCLE ( 'NONE', #11542, 0.5000000000000004441 ) ;
#3750=AXIS2_PLACEMENT_3D ( 'NONE', #2561, #27138, #20450 ) ;
#3751=VERTEX_POINT ( 'NONE', #7554 ) ;
#3752=DIRECTION ( 'NONE',  ( 0.000000000000000000, 0.000000000000000000, -1.000000000000000000 ) ) ;
#3754=DIRECTION ( 'NONE',  ( 0.6691306063588670083, 0.7431448254773862505, -0.000000000000000000 ) ) ;
#3757=CARTESIAN_POINT ( 'NONE',  ( 14.73239529508889767, 21.45431699865973840, 10.94611345180490503 ) ) ;
#3760=CARTESIAN_POINT ( 'NONE',  ( 14.40879062396295041, 19.98622263052302017, 10.49999999999999822 ) ) ;
#3763=DIRECTION ( 'NONE',  ( -0.000000000000000000, -0.000000000000000000, -1.000000000000000000 ) ) ;
#3767=DIRECTION ( 'NONE',  ( -0.8090169943749505599, -0.5877852522924689183, 0.000000000000000000 ) ) ;
#3770=LINE ( 'NONE', #22453, #25243 ) ;
#3771=EDGE_CURVE ( 'NONE', #10321, #2610, #32557, .T. ) ;
#3772=CARTESIAN_POINT ( 'NONE',  ( 12.80736835487433112, 15.68301270189216545, 11.00000000000000000 ) ) ;
#3774=ADVANCED_FACE ( 'NONE', ( #26445 ), #32353, .T. ) ;
#3775=DIRECTION ( 'NONE',  ( -0.000000000000000000, -0.000000000000000000, -1.000000000000000000 ) ) ;
#3777=ORIENTED_EDGE ( 'NONE', *, *, #13619, .F. ) ;
#3783=AXIS2_PLACEMENT_3D ( 'NONE', #559, #31831, #13137 ) ;
#3787=ORIENTED_EDGE ( 'NONE', *, *, #1941, .T. ) ;
#3791=AXIS2_PLACEMENT_3D ( 'NONE', #4563, #25886, #7397 ) ;
#3792=ORIENTED_EDGE ( 'NONE', *, *, #23020, .T. ) ;
#3794=CIRCLE ( 'NONE', #15488, 6.000000000000003553 ) ;
#3796=ORIENTED_EDGE ( 'NONE', *, *, #12269, .F. ) ;
#3797=DIRECTION ( 'NONE',  ( 0.8660254037844364872, -0.5000000000000038858, 0.000000000000000000 ) ) ;
#3798=ADVANCED_FACE ( 'NONE', ( #20160 ), #4716, .F. ) ;
#3804=ORIENTED_EDGE ( 'NONE', *, *, #21784, .F. ) ;
#3806=CARTESIAN_POINT ( 'NONE',  ( 7.929471891321336230, 25.60217271033461373, 9.000000000000001776 ) ) ;
#3808=CIRCLE ( 'NONE', #18724, 0.9999999999999974465 ) ;
#3809=VECTOR ( 'NONE', #7940, 1000.000000000000000 ) ;
#3810=CARTESIAN_POINT ( 'NONE',  ( -13.94482798346716201, 26.50521816028930999, 11.00000000000000000 ) ) ;
#3814=DIRECTION ( 'NONE',  ( -0.7431448254773953543, -0.6691306063588570163, -0.000000000000000000 ) ) ;
#3815=CIRCLE ( 'NONE', #29141, 0.5000000000000004441 ) ;
#3817=CARTESIAN_POINT ( 'NONE',  ( -8.927394655428429360, 11.06314620770957013, 11.00000000000000000 ) ) ;
#3819=CARTESIAN_POINT ( 'NONE',  ( -10.77256156952734223, 32.87247436945333590, 10.76099332938164288 ) ) ;
#3821=DIRECTION ( 'NONE',  ( 0.000000000000000000, 0.000000000000000000, 1.000000000000000000 ) ) ;
#3824=PLANE ( 'NONE',  #11599 ) ;
#3825=FACE_OUTER_BOUND ( 'NONE', #8701, .T. ) ;
#3828=CARTESIAN_POINT ( 'NONE',  ( 9.331903152615748098, 11.35703883385568780, 7.000000000000000000 ) ) ;
#3840=AXIS2_PLACEMENT_3D ( 'NONE', #1687, #19213, #38098 ) ;
#3843=VERTEX_POINT ( 'NONE', #31934 ) ;
#3845=CARTESIAN_POINT ( 'NONE',  ( -6.557822374958138134, 35.99981354310120452, 10.49999999999999822 ) ) ;
#3846=EDGE_CURVE ( 'NONE', #9898, #22045, #4103, .T. ) ;
#3848=ADVANCED_FACE ( 'NONE', ( #12207 ), #24601, .T. ) ;
#3849=AXIS2_PLACEMENT_3D ( 'NONE', #32304, #31893, #25591 ) ;
#3854=ORIENTED_EDGE ( 'NONE', *, *, #25042, .F. ) ;
#3860=DIRECTION ( 'NONE',  ( 1.000000000000000000, 1.224646799147353947E-16, 0.000000000000000000 ) ) ;
#3862=DIRECTION ( 'NONE',  ( 1.000000000000000000, 0.000000000000000000, 0.000000000000000000 ) ) ;
#3863=ORIENTED_EDGE ( 'NONE', *, *, #1692, .T. ) ;
#3864=DIRECTION ( 'NONE',  ( -1.000000000000000000, 0.000000000000000000, 0.000000000000000000 ) ) ;
#3865=DIRECTION ( 'NONE',  ( -0.5000000000000041078, -0.8660254037844362651, 0.000000000000000000 ) ) ;
#3866=CYLINDRICAL_SURFACE ( 'NONE', #31832, 0.5000000000000004441 ) ;
#3867=EDGE_CURVE ( 'NONE', #4036, #31246, #36203, .T. ) ;
#3870=AXIS2_PLACEMENT_3D ( 'NONE', #10063, #3367, #34258 ) ;
#3871=ORIENTED_EDGE ( 'NONE', *, *, #26288, .T. ) ;
#3873=DIRECTION ( 'NONE',  ( 1.000000000000000000, 0.000000000000000000, 0.000000000000000000 ) ) ;
#3880=CARTESIAN_POINT ( 'NONE',  ( 3.992867117591230919, 8.524771480177550487, 10.49999999999999822 ) ) ;
#3888=ORIENTED_EDGE ( 'NONE', *, *, #8164, .T. ) ;
#3890=LINE ( 'NONE', #38226, #27801 ) ;
#3891=DIRECTION ( 'NONE',  ( 0.9945218953682730678, -0.1045284632676564962, 0.000000000000000000 ) ) ;
#3892=ORIENTED_EDGE ( 'NONE', *, *, #18834, .F. ) ;
#3894=B_SPLINE_CURVE_WITH_KNOTS ( 'NONE', 3,
 ( #26383, #17863, #30244, #4850, #7698, #14804 ),
 .UNSPECIFIED., .F., .F.,
 ( 4, 2, 4 ),
 ( 0.000000000000000000, 0.5000000000000000000, 1.000000000000000000 ),
 .UNSPECIFIED. ) ;
#3896=EDGE_LOOP ( 'NONE', ( #11240, #32138, #1348, #19088, #151 ) ) ;
#3901=ORIENTED_EDGE ( 'NONE', *, *, #36880, .T. ) ;
#3903=VECTOR ( 'NONE', #16356, 1000.000000000000000 ) ;
#3906=CARTESIAN_POINT ( 'NONE',  ( 8.472151273871505239, 28.78272654129060371, 11.00000000000000000 ) ) ;
#3908=EDGE_CURVE ( 'NONE', #5670, #38309, #5312, .T. ) ;
#3911=EDGE_CURVE ( 'NONE', #31137, #20501, #8967, .T. ) ;
#3915=DIRECTION ( 'NONE',  ( -0.4067366430757888840, 0.9135454576426058626, 0.000000000000000000 ) ) ;
#3916=ORIENTED_EDGE ( 'NONE', *, *, #29266, .F. ) ;
#3918=VERTEX_POINT ( 'NONE', #17723 ) ;
#3920=ADVANCED_FACE ( 'NONE', ( #18119 ), #2668, .T. ) ;
#3922=DIRECTION ( 'NONE',  ( 0.000000000000000000, 0.000000000000000000, 1.000000000000000000 ) ) ;
#3924=ORIENTED_EDGE ( 'NONE', *, *, #14241, .F. ) ;
#3926=DIRECTION ( 'NONE',  ( 0.7032331762534107522, 0.07391278520356026061, -0.7071067811865416886 ) ) ;
#3927=VECTOR ( 'NONE', #8213, 1000.000000000000114 ) ;
#3928=EDGE_LOOP ( 'NONE', ( #39432, #12397, #6346 ) ) ;
#3930=LINE ( 'NONE', #4333, #23159 ) ;
#3933=EDGE_LOOP ( 'NONE', ( #26449, #21740, #1211, #26684, #33240 ) ) ;
#3936=DIRECTION ( 'NONE',  ( 0.4067366430758009299, 0.9135454576426005335, 0.000000000000000000 ) ) ;
#3938=EDGE_LOOP ( 'NONE', ( #7219, #21347, #12485, #33491, #39613 ) ) ;
#3940=PLANE ( 'NONE',  #31686 ) ;
#3941=CARTESIAN_POINT ( 'NONE',  ( 12.30736835487432934, 14.81698729810772797, 11.00000000000000000 ) ) ;
#3945=EDGE_CURVE ( 'NONE', #18383, #7720, #16959, .T. ) ;
#3948=CIRCLE ( 'NONE', #19520, 1.000000000000000444 ) ;
#3949=EDGE_LOOP ( 'NONE', ( #4698, #19522, #26894, #1254 ) ) ;
#3952=ORIENTED_EDGE ( 'NONE', *, *, #2916, .T. ) ;
#3953=CARTESIAN_POINT ( 'NONE',  ( -7.468455364333119739, 29.89744377950679421, 10.50000000000000000 ) ) ;
#3954=EDGE_CURVE ( 'NONE', #17593, #20190, #12008, .T. ) ;
#3955=DIRECTION ( 'NONE',  ( 1.000000000000000000, 0.000000000000000000, 0.000000000000000000 ) ) ;
#3956=DIRECTION ( 'NONE',  ( 0.000000000000000000, 0.000000000000000000, 1.000000000000000000 ) ) ;
#3959=ORIENTED_EDGE ( 'NONE', *, *, #15015, .F. ) ;
#3960=DIRECTION ( 'NONE',  ( -0.000000000000000000, -0.000000000000000000, -1.000000000000000000 ) ) ;
#3961=LINE ( 'NONE', #28745, #23974 ) ;
#3964=DIRECTION ( 'NONE',  ( 0.6691306063588570163, -0.7431448254773953543, 0.000000000000000000 ) ) ;
#3970=CARTESIAN_POINT ( 'NONE',  ( 3.712277862705659182, 32.06720926237454705, 10.74999999999998757 ) ) ;
#3971=CARTESIAN_POINT ( 'NONE',  ( 13.13451774850152809, 16.06441397984643871, 10.49999999999999822 ) ) ;
#3972=AXIS2_PLACEMENT_3D ( 'NONE', #5505, #20766, #39635 ) ;
#3978=VERTEX_POINT ( 'NONE', #30506 ) ;
#3980=DIRECTION ( 'NONE',  ( 0.000000000000000000, 0.000000000000000000, -1.000000000000000000 ) ) ;
#3986=VERTEX_POINT ( 'NONE', #20955 ) ;
#3994=ORIENTED_EDGE ( 'NONE', *, *, #10162, .T. ) ;
#3995=FACE_OUTER_BOUND ( 'NONE', #16900, .T. ) ;
#4000=AXIS2_PLACEMENT_3D ( 'NONE', #38140, #1578, #16411 ) ;
#4001=ORIENTED_EDGE ( 'NONE', *, *, #3395, .T. ) ;
#4010=CIRCLE ( 'NONE', #2086, 0.9999999999999994449 ) ;
#4012=FACE_OUTER_BOUND ( 'NONE', #3938, .T. ) ;
#4013=CARTESIAN_POINT ( 'NONE',  ( -1.932616070714923806, 8.598021898908978500, 9.500000000000000000 ) ) ;
#4015=DIRECTION ( 'NONE',  ( -0.000000000000000000, -0.000000000000000000, -1.000000000000000000 ) ) ;
#4016=ORIENTED_EDGE ( 'NONE', *, *, #36452, .F. ) ;
#4018=DIRECTION ( 'NONE',  ( -0.4999999999999912292, 0.8660254037844437036, 0.000000000000000000 ) ) ;
#4020=EDGE_CURVE ( 'NONE', #9166, #36223, #734, .T. ) ;
#4022=FACE_OUTER_BOUND ( 'NONE', #2368, .T. ) ;
#4025=CARTESIAN_POINT ( 'NONE',  ( 13.24038105676655164, 15.43301270189216368, 7.000000000000000000 ) ) ;
#4027=AXIS2_PLACEMENT_3D ( 'NONE', #27458, #15271, #8978 ) ;
#4032=CARTESIAN_POINT ( 'NONE',  ( 1.278175571583998860, 14.08178954835375940, 9.000000000000001776 ) ) ;
#4033=ORIENTED_EDGE ( 'NONE', *, *, #1071, .T. ) ;
#4035=FACE_OUTER_BOUND ( 'NONE', #13688, .T. ) ;
#4036=VERTEX_POINT ( 'NONE', #32960 ) ;
#4039=EDGE_CURVE ( 'NONE', #4629, #13902, #5115, .T. ) ;
#4040=VECTOR ( 'NONE', #7090, 1000.000000000000114 ) ;
#4041=CARTESIAN_POINT ( 'NONE',  ( -1.000000000000000000, 37.50000000000000711, 10.50000000000000000 ) ) ;
#4042=ORIENTED_EDGE ( 'NONE', *, *, #17226, .T. ) ;
#4044=EDGE_CURVE ( 'NONE', #13649, #15610, #10536, .T. ) ;
#4048=VECTOR ( 'NONE', #31176, 1000.000000000000114 ) ;
#4052=EDGE_CURVE ( 'NONE', #27294, #12629, #813, .T. ) ;
#4053=LINE ( 'NONE', #13193, #32661 ) ;
#4054=DIRECTION ( 'NONE',  ( 0.3090169943749560000, 0.9510565162951507556, 0.000000000000000000 ) ) ;
#4056=DIRECTION ( 'NONE',  ( -1.000000000000000000, 0.000000000000000000, 0.000000000000000000 ) ) ;
#4057=VERTEX_POINT ( 'NONE', #12801 ) ;
#4061=DIRECTION ( 'NONE',  ( -0.6916548014802208488, 0.1470157664652026186, 0.7071067811865512365 ) ) ;
#4066=EDGE_CURVE ( 'NONE', #17580, #12323, #28042, .T. ) ;
#4067=CARTESIAN_POINT ( 'NONE',  ( 8.796116341590819232, 23.42450908139080568, 9.000000000000001776 ) ) ;
#4069=EDGE_CURVE ( 'NONE', #35744, #38427, #31829, .T. ) ;
#4072=CARTESIAN_POINT ( 'NONE',  ( -1.100969307443859568, 12.51061230184420481, 10.50000000000000533 ) ) ;
#4073=ORIENTED_EDGE ( 'NONE', *, *, #32797, .T. ) ;
#4075=CIRCLE ( 'NONE', #26794, 6.000000000000005329 ) ;
#4079=ORIENTED_EDGE ( 'NONE', *, *, #34599, .T. ) ;
#4080=ORIENTED_EDGE ( 'NONE', *, *, #34551, .F. ) ;
#4084=CARTESIAN_POINT ( 'NONE',  ( -12.71633695260880970, 14.58086916811587130, 10.68306085400111805 ) ) ;
#4086=AXIS2_PLACEMENT_3D ( 'NONE', #11522, #31004, #36900 ) ;
#4087=CARTESIAN_POINT ( 'NONE',  ( -13.46205012405082435, 15.88307354764209300, 7.318814606722385818 ) ) ;
#4090=LINE ( 'NONE', #32337, #16147 ) ;
#4091=DIRECTION ( 'NONE',  ( -0.8660254037844348218, 0.5000000000000066613, 0.000000000000000000 ) ) ;
#4095=CARTESIAN_POINT ( 'NONE',  ( -0.5000000000000004441, 37.00000000000000711, 9.000000000000001776 ) ) ;
#4096=VERTEX_POINT ( 'NONE', #617 ) ;
#4098=AXIS2_PLACEMENT_3D ( 'NONE', #37555, #12566, #7256 ) ;
#4101=ORIENTED_EDGE ( 'NONE', *, *, #38640, .F. ) ;
#4103=LINE ( 'NONE', #2475, #16306 ) ;
#4105=CONICAL_SURFACE ( 'NONE', #7997, 0.5000000000000007772, 0.7853981633974519427 ) ;
#4106=CYLINDRICAL_SURFACE ( 'NONE', #33056, 0.5000000000000004441 ) ;
#4107=CYLINDRICAL_SURFACE ( 'NONE', #3280, 0.5000000000000004441 ) ;
#4108=VECTOR ( 'NONE', #32621, 1000.000000000000114 ) ;
#4112=EDGE_CURVE ( 'NONE', #2130, #28310, #12993, .T. ) ;
#4114=CARTESIAN_POINT ( 'NONE',  ( -10.44103466624267185, 32.57396620494226624, 7.500000000000004441 ) ) ;
#4115=EDGE_CURVE ( 'NONE', #28177, #21498, #9365, .T. ) ;
#4117=CIRCLE ( 'NONE', #9328, 6.000000000000010658 ) ;
#4118=ORIENTED_EDGE ( 'NONE', *, *, #15991, .F. ) ;
#4121=DIRECTION ( 'NONE',  ( -0.1470157664652030627, -0.6916548014802235134, -0.7071067811865485719 ) ) ;
#4123=VERTEX_POINT ( 'NONE', #220 ) ;
#4125=CYLINDRICAL_SURFACE ( 'NONE', #37167, 6.000000000000015987 ) ;
#4128=CARTESIAN_POINT ( 'NONE',  ( 7.645071344821493753, 9.594463043616155318, 7.000000000000000000 ) ) ;
#4130=CARTESIAN_POINT ( 'NONE',  ( 12.09742388243072675, 14.36084852659828215, 10.49999999999999822 ) ) ;
#4131=AXIS2_PLACEMENT_3D ( 'NONE', #31247, #27797, #6842 ) ;
#4135=CARTESIAN_POINT ( 'NONE',  ( -0.5000000000000008882, 36.00000000000000711, 10.00000000000000000 ) ) ;
#4137=VERTEX_POINT ( 'NONE', #9564 ) ;
#4139=DIRECTION ( 'NONE',  ( 0.000000000000000000, 0.000000000000000000, -1.000000000000000000 ) ) ;
#4141=ORIENTED_EDGE ( 'NONE', *, *, #19454, .F. ) ;
#4143=EDGE_CURVE ( 'NONE', #10321, #30937, #21947, .T. ) ;
#4145=ADVANCED_FACE ( 'NONE', ( #25197 ), #6498, .F. ) ;
#4147=EDGE_LOOP ( 'NONE', ( #30293, #895, #25239, #29580 ) ) ;
#4149=CIRCLE ( 'NONE', #8717, 6.000000000000003553 ) ;
#4150=FACE_OUTER_BOUND ( 'NONE', #30902, .T. ) ;
#4152=CARTESIAN_POINT ( 'NONE',  ( 19.48557158514997667, 33.74999999999982236, 7.000000000000000000 ) ) ;
#4154=LINE ( 'NONE', #16559, #30802 ) ;
#4156=CARTESIAN_POINT ( 'NONE',  ( -11.40045278936307405, 32.09219743356619858, 10.82238787011334935 ) ) ;
#4158=CARTESIAN_POINT ( 'NONE',  ( 13.03339520833710985, 15.55251603720134668, 10.94611345180490680 ) ) ;
#4160=CARTESIAN_POINT ( 'NONE',  ( -6.373266493267534472, 35.58529424598371094, 10.99999999999999289 ) ) ;
#4161=CARTESIAN_POINT ( 'NONE',  ( -8.137585970691985082, 29.15429895402941440, 10.50000000000000000 ) ) ;
#4164=EDGE_CURVE ( 'NONE', #20190, #33341, #38375, .T. ) ;
#4165=CARTESIAN_POINT ( 'NONE',  ( -10.14158519589098795, 20.93132230382252246, 10.74999999999998579 ) ) ;
#4167=EDGE_CURVE ( 'NONE', #35366, #36352, #22535, .T. ) ;
#4169=CARTESIAN_POINT ( 'NONE',  ( -8.927394655428429360, 11.06314620770957013, 7.000000000000000000 ) ) ;
#4170=VERTEX_POINT ( 'NONE', #4260 ) ;
#4175=FACE_OUTER_BOUND ( 'NONE', #15420, .T. ) ;
#4179=B_SPLINE_SURFACE_WITH_KNOTS ( 'NONE', 1, 3, ( 
 ( #12688, #4700, #16142, #37869, #28526, #26229, #701, #13079, #26430, #38625 ),
 ( #23184, #32744, #10044, #17105, #35584, #7742, #4901, #32545, #14242, #23987 ) ),
 .UNSPECIFIED., .F., .F., .F.,
 ( 2, 2 ),
 ( 4, 2, 2, 2, 4 ),
 ( 0.000000000000000000, 1.000000000000000000 ),
 ( -1.003840680322661605, -0.6111415986239409071, -0.2184425169252202648, 0.1742565647735004053, 0.5669556464722210753 ),
 .UNSPECIFIED. ) ;
#4180=VERTEX_POINT ( 'NONE', #38791 ) ;
#4189=ORIENTED_EDGE ( 'NONE', *, *, #8503, .F. ) ;
#4192=CYLINDRICAL_SURFACE ( 'NONE', #462, 0.5000000000000000000 ) ;
#4194=AXIS2_PLACEMENT_3D ( 'NONE', #8479, #21659, #36511 ) ;
#4195=EDGE_LOOP ( 'NONE', ( #38731, #18506, #39505, #34141, #7421 ) ) ;
#4198=VECTOR ( 'NONE', #39441, 1000.000000000000000 ) ;
#4201=ADVANCED_FACE ( 'NONE', ( #20112 ), #13716, .T. ) ;
#4206=ORIENTED_EDGE ( 'NONE', *, *, #24248, .T. ) ;
#4209=DIRECTION ( 'NONE',  ( -0.5254827454987561763, 0.4731467892558144928, -0.7071067811865497932 ) ) ;
#4211=FACE_OUTER_BOUND ( 'NONE', #19288, .T. ) ;
#4212=VERTEX_POINT ( 'NONE', #16661 ) ;
#4214=CARTESIAN_POINT ( 'NONE',  ( -11.81630298851966288, 31.79381426990562787, 7.000000000000000000 ) ) ;
#4215=CARTESIAN_POINT ( 'NONE',  ( 4.940908595777813161, 35.94977745735560859, 7.500000000000000888 ) ) ;
#4216=B_SPLINE_CURVE_WITH_KNOTS ( 'NONE', 3,
 ( #768, #13151, #25543, #34898, #26147, #23314, #19865, #13556 ),
 .UNSPECIFIED., .F., .F.,
 ( 4, 2, 2, 4 ),
 ( 0.000000000000000000, 0.0002364868538934252319, 0.0004729737077868504638, 0.0009459474155737089508 ),
 .UNSPECIFIED. ) ;
#4218=DIRECTION ( 'NONE',  ( 0.2876062384759395796, -0.6459741880212476195, 0.7071067811865551223 ) ) ;
#4222=LINE ( 'NONE', #10122, #6222 ) ;
#4223=VECTOR ( 'NONE', #2231, 1000.000000000000000 ) ;
#4224=ORIENTED_EDGE ( 'NONE', *, *, #15317, .T. ) ;
#4226=CIRCLE ( 'NONE', #1070, 0.5000000000000002220 ) ;
#4227=PLANE ( 'NONE',  #36256 ) ;
#4238=LINE ( 'NONE', #7883, #3064 ) ;
#4239=FACE_OUTER_BOUND ( 'NONE', #9065, .T. ) ;
#4240=ORIENTED_EDGE ( 'NONE', *, *, #8884, .T. ) ;
#4242=ORIENTED_EDGE ( 'NONE', *, *, #38933, .F. ) ;
#4243=AXIS2_PLACEMENT_3D ( 'NONE', #11596, #17503, #4693 ) ;
#4245=EDGE_LOOP ( 'NONE', ( #5551, #27933, #35489, #36307 ) ) ;
#4247=CARTESIAN_POINT ( 'NONE',  ( 14.61015742389396976, 25.89965074521812127, 7.102474990965866652 ) ) ;
#4248=PLANE ( 'NONE',  #28435 ) ;
#4249=ORIENTED_EDGE ( 'NONE', *, *, #14847, .F. ) ;
#4250=AXIS2_PLACEMENT_3D ( 'NONE', #22655, #1137, #22256 ) ;
#4252=EDGE_LOOP ( 'NONE', ( #4224, #2607, #33309, #12390 ) ) ;
#4255=CIRCLE ( 'NONE', #30856, 1.000000000000004441 ) ;
#4256=ORIENTED_EDGE ( 'NONE', *, *, #10056, .T. ) ;
#4260=CARTESIAN_POINT ( 'NONE',  ( 6.576253646258392038, 14.29921418520926046, 10.00000000000000000 ) ) ;
#4270=CARTESIAN_POINT ( 'NONE',  ( 2.317734025672766318, 9.191051544684723851, 7.000000000000000000 ) ) ;
#4275=DIRECTION ( 'NONE',  ( -0.000000000000000000, -0.000000000000000000, 1.000000000000000000 ) ) ;
#4276=ORIENTED_EDGE ( 'NONE', *, *, #33558, .F. ) ;
#4277=VECTOR ( 'NONE', #17643, 1000.000000000000000 ) ;
#4282=EDGE_CURVE ( 'NONE', #34166, #35530, #18744, .T. ) ;
#4285=ADVANCED_FACE ( 'NONE', ( #23148 ), #31890, .T. ) ;
#4286=ORIENTED_EDGE ( 'NONE', *, *, #30344, .F. ) ;
#4287=VERTEX_POINT ( 'NONE', #19496 ) ;
#4289=LINE ( 'NONE', #34975, #19147 ) ;
#4290=CARTESIAN_POINT ( 'NONE',  ( -12.34742388243084577, 14.79386122849067142, 11.00000000000000000 ) ) ;
#4297=VERTEX_POINT ( 'NONE', #1222 ) ;
#4300=VERTEX_POINT ( 'NONE', #10970 ) ;
#4304=EDGE_CURVE ( 'NONE', #14016, #20580, #14005, .T. ) ;
#4305=ORIENTED_EDGE ( 'NONE', *, *, #34579, .T. ) ;
#4307=EDGE_CURVE ( 'NONE', #36822, #7885, #24107, .T. ) ;
#4311=AXIS2_PLACEMENT_3D ( 'NONE', #33641, #493, #21229 ) ;
#4312=DIRECTION ( 'NONE',  ( 0.000000000000000000, -0.000000000000000000, 1.000000000000000000 ) ) ;
#4313=VECTOR ( 'NONE', #4743, 999.9999999999998863 ) ;
#4314=FACE_OUTER_BOUND ( 'NONE', #23220, .T. ) ;
#4321=VERTEX_POINT ( 'NONE', #4465 ) ;
#4323=ORIENTED_EDGE ( 'NONE', *, *, #11912, .T. ) ;
#4326=CARTESIAN_POINT ( 'NONE',  ( -6.654030453887870067, 35.94335816374513115, 7.000000000000000000 ) ) ;
#4331=ORIENTED_EDGE ( 'NONE', *, *, #5599, .T. ) ;
#4333=CARTESIAN_POINT ( 'NONE',  ( -6.811226782241547539, 35.33967249274200384, 7.000000000000000000 ) ) ;
#4336=VECTOR ( 'NONE', #25281, 1000.000000000000000 ) ;
#4338=VERTEX_POINT ( 'NONE', #25588 ) ;
#4343=ORIENTED_EDGE ( 'NONE', *, *, #13774, .T. ) ;
#4347=ORIENTED_EDGE ( 'NONE', *, *, #14214, .T. ) ;
#4356=DIRECTION ( 'NONE',  ( 0.000000000000000000, 0.000000000000000000, -1.000000000000000000 ) ) ;
#4357=VECTOR ( 'NONE', #1257, 999.9999999999998863 ) ;
#4358=AXIS2_PLACEMENT_3D ( 'NONE', #37526, #21482, #25126 ) ;
#4359=DIRECTION ( 'NONE',  ( 0.4067366430758009299, 0.9135454576426005335, 0.000000000000000000 ) ) ;
#4361=LINE ( 'NONE', #29552, #10756 ) ;
#4363=CARTESIAN_POINT ( 'NONE',  ( -6.557822374958135470, 35.99981354310119741, 10.49999999999999289 ) ) ;
#4364=DIRECTION ( 'NONE',  ( 0.3090169943749573878, 0.9510565162951503115, 0.000000000000000000 ) ) ;
#4367=CARTESIAN_POINT ( 'NONE',  ( -0.4999999999999998890, 37.00000000000000711, 7.000000000000000000 ) ) ;
#4368=CARTESIAN_POINT ( 'NONE',  ( 9.625795778761983001, 10.95253033666821274, 7.000000000000000000 ) ) ;
#4369=EDGE_CURVE ( 'NONE', #13430, #13564, #28842, .T. ) ;
#4371=PLANE ( 'NONE',  #20454 ) ;
#4372=ORIENTED_EDGE ( 'NONE', *, *, #14614, .F. ) ;
#4375=ADVANCED_FACE ( 'NONE', ( #7295 ), #10360, .F. ) ;
#4376=EDGE_CURVE ( 'NONE', #6805, #16537, #19701, .T. ) ;
#4380=EDGE_LOOP ( 'NONE', ( #22572, #36401, #21102, #26460, #16646, #25969, #9225 ) ) ;
#4384=CARTESIAN_POINT ( 'NONE',  ( -8.411683849014160330, 19.76687823897114882, 7.000000000000000000 ) ) ;
#4387=EDGE_CURVE ( 'NONE', #17829, #3843, #26194, .T. ) ;
#4391=ORIENTED_EDGE ( 'NONE', *, *, #1813, .F. ) ;
#4398=AXIS2_PLACEMENT_3D ( 'NONE', #21731, #30690, #6290 ) ;
#4399=AXIS2_PLACEMENT_3D ( 'NONE', #23486, #14141, #36684 ) ;
#4403=DIRECTION ( 'NONE',  ( -0.9781476007338042455, 0.2079116908177663370, 0.000000000000000000 ) ) ;
#4405=EDGE_CURVE ( 'NONE', #29211, #28177, #18267, .T. ) ;
#4408=EDGE_CURVE ( 'NONE', #26227, #38309, #30527, .T. ) ;
#4410=AXIS2_PLACEMENT_3D ( 'NONE', #12099, #39527, #18796 ) ;
#4412=CARTESIAN_POINT ( 'NONE',  ( 14.11133924723984379, 27.61078317377175750, 11.00000000000000000 ) ) ;
#4414=DIRECTION ( 'NONE',  ( -0.000000000000000000, -0.000000000000000000, -1.000000000000000000 ) ) ;
#4415=EDGE_LOOP ( 'NONE', ( #2780, #2800, #21972 ) ) ;
#4418=DIRECTION ( 'NONE',  ( 0.000000000000000000, 0.000000000000000000, 1.000000000000000000 ) ) ;
#4421=ADVANCED_FACE ( 'NONE', ( #14411 ), #36545, .T. ) ;
#4422=CARTESIAN_POINT ( 'NONE',  ( 6.811226782241711852, 35.33967249274190436, 7.500000000000000888 ) ) ;
#4425=AXIS2_PLACEMENT_3D ( 'NONE', #25467, #19788, #13895 ) ;
#4426=VERTEX_POINT ( 'NONE', #38991 ) ;
#4429=CARTESIAN_POINT ( 'NONE',  ( -0.4999999999999998890, 37.33905845026563952, 10.87262190629436098 ) ) ;
#4430=ADVANCED_FACE ( 'NONE', ( #39189 ), #2621, .T. ) ;
#4432=DIRECTION ( 'NONE',  ( 0.7431448254773953543, 0.6691306063588570163, 0.000000000000000000 ) ) ;
#4444=VERTEX_POINT ( 'NONE', #5463 ) ;
#4446=EDGE_LOOP ( 'NONE', ( #14663, #9636, #3066, #23674, #13844, #2492, #27196 ) ) ;
#4448=DIRECTION ( 'NONE',  ( 0.2079116908177519041, -0.9781476007338072431, 0.000000000000000000 ) ) ;
#4449=ORIENTED_EDGE ( 'NONE', *, *, #32946, .F. ) ;
#4451=FACE_OUTER_BOUND ( 'NONE', #10237, .T. ) ;
#4453=ORIENTED_EDGE ( 'NONE', *, *, #236, .F. ) ;
#4455=ORIENTED_EDGE ( 'NONE', *, *, #18486, .T. ) ;
#4458=CIRCLE ( 'NONE', #7048, 0.5000000000000004441 ) ;
#4459=AXIS2_PLACEMENT_3D ( 'NONE', #3693, #31529, #31922 ) ;
#4460=ORIENTED_EDGE ( 'NONE', *, *, #22084, .T. ) ;
#4463=VECTOR ( 'NONE', #866, 1000.000000000000114 ) ;
#4465=CARTESIAN_POINT ( 'NONE',  ( 12.05736835487432579, 14.38397459621550567, 7.499999999999997335 ) ) ;
#4467=LINE ( 'NONE', #16870, #9055 ) ;
#4469=CARTESIAN_POINT ( 'NONE',  ( 0.000000000000000000, 0.000000000000000000, 0.000000000000000000 ) ) ;
#4470=DIRECTION ( 'NONE',  ( 0.5720614028176880250, 0.4156269377774530760, -0.7071067811865446862 ) ) ;
#4475=ORIENTED_EDGE ( 'NONE', *, *, #31463, .F. ) ;
#4477=FACE_OUTER_BOUND ( 'NONE', #28424, .T. ) ;
#4478=EDGE_CURVE ( 'NONE', #11050, #29636, #14953, .T. ) ;
#4481=LINE ( 'NONE', #16886, #14670 ) ;
#4485=CIRCLE ( 'NONE', #27195, 0.5000000000000000000 ) ;
#4488=DIRECTION ( 'NONE',  ( 1.000000000000000000, 1.224646799147351235E-16, -0.000000000000000000 ) ) ;
#4490=ORIENTED_EDGE ( 'NONE', *, *, #16846, .T. ) ;
#4491=CIRCLE ( 'NONE', #28492, 0.9999999999999995559 ) ;
#4494=FACE_OUTER_BOUND ( 'NONE', #4415, .T. ) ;
#4496=DIRECTION ( 'NONE',  ( 0.2185080122244173473, 0.6724985119639624864, -0.7071067811865404673 ) ) ;
#4500=DIRECTION ( 'NONE',  ( 0.8090169943749423442, -0.5877852522924800205, 0.000000000000000000 ) ) ;
#4507=DIRECTION ( 'NONE',  ( 1.000000000000000000, 0.000000000000000000, 0.000000000000000000 ) ) ;
#4510=ORIENTED_EDGE ( 'NONE', *, *, #21090, .F. ) ;
#4512=EDGE_CURVE ( 'NONE', #15610, #32625, #33159, .T. ) ;
#4514=CARTESIAN_POINT ( 'NONE',  ( -6.354454053420248272, 35.54304081427989814, 7.500000000000000888 ) ) ;
#4517=CARTESIAN_POINT ( 'NONE',  ( 11.11016527260166420, 31.83082137946473367, 7.000000000000000000 ) ) ;
#4522=LINE ( 'NONE', #26452, #17130 ) ;
#4526=DIRECTION ( 'NONE',  ( 0.000000000000000000, 0.000000000000000000, 1.000000000000000000 ) ) ;
#4528=ORIENTED_EDGE ( 'NONE', *, *, #22968, .F. ) ;
#4536=ORIENTED_EDGE ( 'NONE', *, *, #17259, .F. ) ;
#4538=DIRECTION ( 'NONE',  ( -0.000000000000000000, -0.000000000000000000, -1.000000000000000000 ) ) ;
#4541=CIRCLE ( 'NONE', #6473, 15.00000000000000000 ) ;
#4542=ORIENTED_EDGE ( 'NONE', *, *, #15471, .T. ) ;
#4545=DIRECTION ( 'NONE',  ( -0.000000000000000000, -0.000000000000000000, -1.000000000000000000 ) ) ;
#4552=ORIENTED_EDGE ( 'NONE', *, *, #23555, .F. ) ;
#4556=EDGE_CURVE ( 'NONE', #5579, #253, #17873, .T. ) ;
#4557=ORIENTED_EDGE ( 'NONE', *, *, #18014, .F. ) ;
#4560=B_SPLINE_CURVE_WITH_KNOTS ( 'NONE', 3,
 ( #18167, #34197, #8818, #18950, #2718, #15107 ),
 .UNSPECIFIED., .F., .F.,
 ( 4, 2, 4 ),
 ( 0.000000000000000000, 0.5000000000000000000, 1.000000000000000000 ),
 .UNSPECIFIED. ) ;
#4561=DIRECTION ( 'NONE',  ( 0.6691306063588671194, 0.7431448254773861395, 0.000000000000000000 ) ) ;
#4562=CONICAL_SURFACE ( 'NONE', #37645, 1.000000000000014655, 0.7853981633974526089 ) ;
#4563=CARTESIAN_POINT ( 'NONE',  ( -9.831584923911586671, 26.22020669908462764, 10.50000000000000000 ) ) ;
#4564=EDGE_CURVE ( 'NONE', #24685, #38824, #35951, .T. ) ;
#4565=EDGE_CURVE ( 'NONE', #7663, #18302, #32911, .T. ) ;
#4566=LINE ( 'NONE', #20012, #3927 ) ;
#4567=DIRECTION ( 'NONE',  ( 0.000000000000000000, 0.000000000000000000, 1.000000000000000000 ) ) ;
#4568=DIRECTION ( 'NONE',  ( 0.1045284632676570929, 0.9945218953682730678, -0.000000000000000000 ) ) ;
#4570=CARTESIAN_POINT ( 'NONE',  ( 1.590043107810628298, 12.61456814725305442, 10.49999999999999467 ) ) ;
#4571=CARTESIAN_POINT ( 'NONE',  ( -1.828660225306042442, 9.087095699275883121, 10.50000000000000000 ) ) ;
#4574=LINE ( 'NONE', #4165, #29029 ) ;
#4577=DIRECTION ( 'NONE',  ( -0.8090169943749426773, 0.5877852522924797984, 0.000000000000000000 ) ) ;
#4578=ORIENTED_EDGE ( 'NONE', *, *, #688, .T. ) ;
#4581=ADVANCED_FACE ( 'NONE', ( #30051 ), #4562, .T. ) ;
#4584=FACE_OUTER_BOUND ( 'NONE', #23081, .T. ) ;
#4586=VERTEX_POINT ( 'NONE', #23956 ) ;
#4588=EDGE_LOOP ( 'NONE', ( #21407, #5230, #40183, #19119 ) ) ;
#4599=AXIS2_PLACEMENT_3D ( 'NONE', #28743, #23053, #23263 ) ;
#4600=DIRECTION ( 'NONE',  ( 0.4999999999999919509, -0.8660254037844432595, 0.000000000000000000 ) ) ;
#4601=CARTESIAN_POINT ( 'NONE',  ( -10.04974741695039242, 22.44923726269184527, 10.49999999999999467 ) ) ;
#4602=DIRECTION ( 'NONE',  ( -0.2079116908177663092, -0.9781476007338040235, 0.000000000000000000 ) ) ;
#4603=ORIENTED_EDGE ( 'NONE', *, *, #20515, .F. ) ;
#4609=CONICAL_SURFACE ( 'NONE', #11748, 1.000000000000002665, 0.7853981633974532750 ) ;
#4610=EDGE_CURVE ( 'NONE', #38482, #6428, #36350, .T. ) ;
#4614=EDGE_LOOP ( 'NONE', ( #6625, #10565, #8299, #19367, #37634 ) ) ;
#4615=CARTESIAN_POINT ( 'NONE',  ( 12.19971670159632637, 4.637739668175409058, 7.500000000000010658 ) ) ;
#4617=AXIS2_PLACEMENT_3D ( 'NONE', #7761, #29901, #38243 ) ;
#4618=CARTESIAN_POINT ( 'NONE',  ( 5.547064146435681131, 36.18820672788721993, 10.94611345180490680 ) ) ;
#4621=VECTOR ( 'NONE', #26848, 1000.000000000000000 ) ;
#4622=CARTESIAN_POINT ( 'NONE',  ( -13.42604558747169463, 21.08886574588681384, 7.000000000000000000 ) ) ;
#4623=CARTESIAN_POINT ( 'NONE',  ( 5.947717410344610656, 34.62949535663720013, 10.00000000000000000 ) ) ;
#4625=FACE_OUTER_BOUND ( 'NONE', #4729, .T. ) ;
#4629=VERTEX_POINT ( 'NONE', #36949 ) ;
#4631=DIRECTION ( 'NONE',  ( -0.8090169943749426773, 0.5877852522924797984, 0.000000000000000000 ) ) ;
#4632=DIRECTION ( 'NONE',  ( -1.000000000000000000, 0.000000000000000000, 0.000000000000000000 ) ) ;
#4638=ADVANCED_FACE ( 'NONE', ( #39984 ), #21700, .T. ) ;
#4643=CARTESIAN_POINT ( 'NONE',  ( -3.607749162633401507, 7.931741834401821123, 11.00000000000000000 ) ) ;
#4646=ORIENTED_EDGE ( 'NONE', *, *, #30393, .T. ) ;
#4648=CARTESIAN_POINT ( 'NONE',  ( 13.47830981910552062, 21.58612669357076896, 10.50000000000000000 ) ) ;
#4650=VECTOR ( 'NONE', #32510, 1000.000000000000227 ) ;
#4651=DIRECTION ( 'NONE',  ( 1.000000000000000000, 0.000000000000000000, 0.000000000000000000 ) ) ;
#4652=CARTESIAN_POINT ( 'NONE',  ( 8.981834765181430313, 10.98821582489669169, 10.99387789255785997 ) ) ;
#4653=B_SPLINE_CURVE_WITH_KNOTS ( 'NONE', 3,
 ( #1522, #7200, #19601, #4158, #10871, #1122 ),
 .UNSPECIFIED., .F., .F.,
 ( 4, 2, 4 ),
 ( 0.000000000000000000, 0.5000000000000000000, 1.000000000000000000 ),
 .UNSPECIFIED. ) ;
#4657=ADVANCED_FACE ( 'NONE', ( #33906 ), #12952, .T. ) ;
#4660=EDGE_CURVE ( 'NONE', #8524, #22764, #16983, .T. ) ;
#4661=EDGE_LOOP ( 'NONE', ( #20499, #36912, #28846, #12553 ) ) ;
#4663=ORIENTED_EDGE ( 'NONE', *, *, #25063, .F. ) ;
#4664=DIRECTION ( 'NONE',  ( -0.7071067811865521247, 0.000000000000000000, -0.7071067811865430208 ) ) ;
#4667=EDGE_CURVE ( 'NONE', #24512, #10050, #37738, .T. ) ;
#4669=ORIENTED_EDGE ( 'NONE', *, *, #12319, .T. ) ;
#4670=CARTESIAN_POINT ( 'NONE',  ( -6.151085731882353969, 35.08626808545859888, 7.500000000000000888 ) ) ;
#4671=DIRECTION ( 'NONE',  ( 0.000000000000000000, 0.000000000000000000, -1.000000000000000000 ) ) ;
#4676=VERTEX_POINT ( 'NONE', #24745 ) ;
#4678=CARTESIAN_POINT ( 'NONE',  ( 0.000000000000000000, 22.50000000000000355, 7.000000000000000000 ) ) ;
#4680=DIRECTION ( 'NONE',  ( 1.000000000000000000, 0.000000000000000000, 0.000000000000000000 ) ) ;
#4684=ORIENTED_EDGE ( 'NONE', *, *, #11757, .F. ) ;
#4689=CARTESIAN_POINT ( 'NONE',  ( 24.58993327517434224, 16.11278406388105111, 7.499999999999996447 ) ) ;
#4691=VERTEX_POINT ( 'NONE', #27994 ) ;
#4693=DIRECTION ( 'NONE',  ( 0.1045284632676569680, 0.9945218953682730678, 0.000000000000000000 ) ) ;
#4695=TOROIDAL_SURFACE ( 'NONE', #27398, 1.000000000000000000, 0.5000000000000000000 ) ;
#4697=DIRECTION ( 'NONE',  ( -0.5000000000000039968, -0.8660254037844363761, 0.000000000000000000 ) ) ;
#4698=ORIENTED_EDGE ( 'NONE', *, *, #21447, .F. ) ;
#4700=CARTESIAN_POINT ( 'NONE',  ( -10.75008043808887948, 32.97797437800713283, 10.49999999999999822 ) ) ;
#4701=PLANE ( 'NONE',  #22594 ) ;
#4702=CARTESIAN_POINT ( 'NONE',  ( -2.538198952020866539, 7.704401919100564378, 10.49999999999999822 ) ) ;
#4704=ORIENTED_EDGE ( 'NONE', *, *, #22788, .T. ) ;
#4706=DIRECTION ( 'NONE',  ( 0.4067366430758010409, 0.9135454576426005335, -0.000000000000000000 ) ) ;
#4712=EDGE_CURVE ( 'NONE', #4212, #23885, #37030, .T. ) ;
#4713=ORIENTED_EDGE ( 'NONE', *, *, #27851, .T. ) ;
#4716=CYLINDRICAL_SURFACE ( 'NONE', #24740, 0.4999999999999999445 ) ;
#4718=CARTESIAN_POINT ( 'NONE',  ( -8.118377661053489902, 10.47536095541709322, 7.000000000000000000 ) ) ;
#4719=ORIENTED_EDGE ( 'NONE', *, *, #39168, .F. ) ;
#4720=CARTESIAN_POINT ( 'NONE',  ( -2.525645716490710679, 8.212903943950959018, 7.000000000000000000 ) ) ;
#4723=CARTESIAN_POINT ( 'NONE',  ( 5.947717410344610656, 34.62949535663720013, 10.50000000000000000 ) ) ;
#4726=CARTESIAN_POINT ( 'NONE',  ( 14.06524961900339399, 27.71236540882591015, 7.500000000000000888 ) ) ;
#4727=DIRECTION ( 'NONE',  ( -0.4999999999999921729, 0.8660254037844432595, 0.000000000000000000 ) ) ;
#4728=DIRECTION ( 'NONE',  ( -0.6724985119639511622, 0.2185080122244150436, -0.7071067811865519026 ) ) ;
#4729=EDGE_LOOP ( 'NONE', ( #24943, #31736, #35055, #4206 ) ) ;
#4731=VERTEX_POINT ( 'NONE', #25145 ) ;
#4734=CARTESIAN_POINT ( 'NONE',  ( -2.036571916123810055, 8.108948098542073879, 10.50000000000000355 ) ) ;
#4738=EDGE_CURVE ( 'NONE', #16076, #15620, #21895, .T. ) ;
#4743=DIRECTION ( 'NONE',  ( -0.3090169943749450643, 0.9510565162951544194, -0.000000000000000000 ) ) ;
#4750=ORIENTED_EDGE ( 'NONE', *, *, #28240, .T. ) ;
#4758=VECTOR ( 'NONE', #31494, 1000.000000000000114 ) ;
#4760=ORIENTED_EDGE ( 'NONE', *, *, #34932, .T. ) ;
#4763=AXIS2_PLACEMENT_3D ( 'NONE', #21855, #12709, #18225 ) ;
#4765=FACE_OUTER_BOUND ( 'NONE', #32845, .T. ) ;
#4767=DIRECTION ( 'NONE',  ( -1.000000000000000000, 0.000000000000000000, 0.000000000000000000 ) ) ;
#4768=CARTESIAN_POINT ( 'NONE',  ( -14.11133924723978161, 27.61078317377194224, 11.00000000000000000 ) ) ;
#4769=DIRECTION ( 'NONE',  ( -0.2079116908177533474, 0.9781476007338067991, 0.000000000000000000 ) ) ;
#4772=CARTESIAN_POINT ( 'NONE',  ( -0.5000000000000004441, 32.50000000000000000, 10.00000000000000000 ) ) ;
#4773=CARTESIAN_POINT ( 'NONE',  ( -0.9999999999999993339, 33.00000000000000000, 10.50000000000000000 ) ) ;
#4776=CARTESIAN_POINT ( 'NONE',  ( 5.440908595777814050, 35.94977745735560859, 7.500000000000000888 ) ) ;
#4778=VERTEX_POINT ( 'NONE', #34298 ) ;
#4782=ADVANCED_FACE ( 'NONE', ( #2816 ), #15210, .T. ) ;
#4784=FACE_OUTER_BOUND ( 'NONE', #11902, .T. ) ;
#4786=EDGE_LOOP ( 'NONE', ( #3221, #29275, #15404, #36512 ) ) ;
#4790=CARTESIAN_POINT ( 'NONE',  ( -14.97009266215794021, 21.42933399866948463, 11.00000000000000000 ) ) ;
#4794=AXIS2_PLACEMENT_3D ( 'NONE', #25889, #38289, #14512 ) ;
#4800=LINE ( 'NONE', #1151, #1158 ) ;
#4801=CARTESIAN_POINT ( 'NONE',  ( -12.30264615366000491, 13.91750221598363346, 7.102637441331451029 ) ) ;
#4803=CARTESIAN_POINT ( 'NONE',  ( -8.007761790012255076, 9.776959832083379709, 11.00000000000000000 ) ) ;
#4804=EDGE_LOOP ( 'NONE', ( #13605, #24050, #2645, #25143 ) ) ;
#4806=VECTOR ( 'NONE', #39449, 999.9999999999998863 ) ;
#4814=EDGE_CURVE ( 'NONE', #35744, #14392, #35747, .T. ) ;
#4816=EDGE_CURVE ( 'NONE', #21531, #22937, #764, .T. ) ;
#4817=DIRECTION ( 'NONE',  ( -0.4999999999999920619, 0.8660254037844433705, 0.000000000000000000 ) ) ;
#4818=CARTESIAN_POINT ( 'NONE',  ( 6.354454053420414361, 35.54304081427980577, 11.00000000000000000 ) ) ;
#4825=CARTESIAN_POINT ( 'NONE',  ( 12.53339520833710985, 14.68649063341690564, 10.94611345180490680 ) ) ;
#4826=CARTESIAN_POINT ( 'NONE',  ( 0.000000000000000000, 22.50000000000000355, 7.000000000000000000 ) ) ;
#4828=CARTESIAN_POINT ( 'NONE',  ( 22.38266491662918156, 24.02827644978115984, 10.00000000000000000 ) ) ;
#4831=LINE ( 'NONE', #17442, #38887 ) ;
#4832=FACE_OUTER_BOUND ( 'NONE', #58, .T. ) ;
#4837=EDGE_CURVE ( 'NONE', #2755, #36470, #14306, .T. ) ;
#4838=DIRECTION ( 'NONE',  ( -0.9135454576426059736, -0.4067366430757888285, 0.000000000000000000 ) ) ;
#4843=DIRECTION ( 'NONE',  ( -0.8090169943749426773, 0.5877852522924796874, -0.000000000000000000 ) ) ;
#4844=ORIENTED_EDGE ( 'NONE', *, *, #15955, .F. ) ;
#4847=CARTESIAN_POINT ( 'NONE',  ( 5.397160494303298250, 36.49555269156554260, 7.455686640544908705 ) ) ;
#4849=DIRECTION ( 'NONE',  ( 0.8660254037844362651, -0.5000000000000041078, -3.469446951953615767E-15 ) ) ;
#4850=CARTESIAN_POINT ( 'NONE',  ( -8.271785691010729025, 10.26421291652884449, 10.94611345180490147 ) ) ;
#4851=VERTEX_POINT ( 'NONE', #16208 ) ;
#4853=ORIENTED_EDGE ( 'NONE', *, *, #9315, .F. ) ;
#4855=ORIENTED_EDGE ( 'NONE', *, *, #6989, .T. ) ;
#4857=EDGE_LOOP ( 'NONE', ( #3094, #10835, #17762 ) ) ;
#4859=CYLINDRICAL_SURFACE ( 'NONE', #13205, 0.5000000000000024425 ) ;
#4861=DIRECTION ( 'NONE',  ( 0.1045284632676436593, -0.9945218953682742891, 0.000000000000000000 ) ) ;
#4864=CARTESIAN_POINT ( 'NONE',  ( 8.593266739736568738, 16.38397459621552699, 10.50000000000000000 ) ) ;
#4866=CARTESIAN_POINT ( 'NONE',  ( -4.727507481117087629, 31.88885898370948269, 11.00000000000000000 ) ) ;
#4867=CYLINDRICAL_SURFACE ( 'NONE', #18285, 0.5000000000000004441 ) ;
#4868=LINE ( 'NONE', #17282, #37031 ) ;
#4873=DIRECTION ( 'NONE',  ( 0.000000000000000000, 0.000000000000000000, 1.000000000000000000 ) ) ;
#4878=CARTESIAN_POINT ( 'NONE',  ( 13.46929972531963848, 26.35070966310165375, 7.500000000000000000 ) ) ;
#4887=FACE_OUTER_BOUND ( 'NONE', #1160, .T. ) ;
#4888=EDGE_LOOP ( 'NONE', ( #3087, #15606, #21210 ) ) ;
#4891=VECTOR ( 'NONE', #15322, 1000.000000000000114 ) ;
#4892=CARTESIAN_POINT ( 'NONE',  ( 10.73859285986296541, 31.49625607628530588, 7.499999999999996447 ) ) ;
#4894=CIRCLE ( 'NONE', #37344, 0.5000000000000004441 ) ;
#4897=VECTOR ( 'NONE', #31475, 1000.000000000000114 ) ;
#4901=CARTESIAN_POINT ( 'NONE',  ( -10.58109189495859326, 32.70007430011122551, 10.96580508970283141 ) ) ;
#4902=DIRECTION ( 'NONE',  ( 0.4999999999999933942, -0.8660254037844425934, 0.000000000000000000 ) ) ;
#4903=CARTESIAN_POINT ( 'NONE',  ( -2.231660708550785799, 7.803782283739876036, 10.49999999999999822 ) ) ;
#4906=CARTESIAN_POINT ( 'NONE',  ( 22.37674264578617667, 24.85189042352198641, 7.000000000000000000 ) ) ;
#4907=ORIENTED_EDGE ( 'NONE', *, *, #31190, .T. ) ;
#4912=EDGE_CURVE ( 'NONE', #31959, #18376, #7246, .T. ) ;
#4914=ADVANCED_FACE ( 'NONE', ( #16611 ), #13550, .T. ) ;
#4921=AXIS2_PLACEMENT_3D ( 'NONE', #13465, #3922, #19564 ) ;
#4922=AXIS2_PLACEMENT_3D ( 'NONE', #23321, #35305, #29210 ) ;
#4924=AXIS2_PLACEMENT_3D ( 'NONE', #9695, #540, #6618 ) ;
#4925=CARTESIAN_POINT ( 'NONE',  ( 2.256323172317815207, 14.28970123917151192, 9.000000000000001776 ) ) ;
#4930=DIRECTION ( 'NONE',  ( -0.6691306063588671194, -0.7431448254773861395, 0.000000000000000000 ) ) ;
#4933=EDGE_CURVE ( 'NONE', #3614, #6055, #5766, .T. ) ;
#4935=ORIENTED_EDGE ( 'NONE', *, *, #37681, .T. ) ;
#4941=ORIENTED_EDGE ( 'NONE', *, *, #12213, .T. ) ;
#4945=CARTESIAN_POINT ( 'NONE',  ( 5.198706521309295780, 29.65540566576566661, 9.000000000000001776 ) ) ;
#4951=DIRECTION ( 'NONE',  ( -0.000000000000000000, -0.000000000000000000, 1.000000000000000000 ) ) ;
#4955=CARTESIAN_POINT ( 'NONE',  ( -8.347978306607240384, 10.15934277794837293, 10.82238861112331740 ) ) ;
#4961=CIRCLE ( 'NONE', #38035, 0.5000000000000004441 ) ;
#4963=VECTOR ( 'NONE', #24081, 1000.000000000000000 ) ;
#4964=ORIENTED_EDGE ( 'NONE', *, *, #29902, .T. ) ;
#4967=PLANE ( 'NONE',  #32990 ) ;
#4970=CARTESIAN_POINT ( 'NONE',  ( 2.421689871081641687, 8.701977744317826335, 9.500000000000000000 ) ) ;
#4971=DIRECTION ( 'NONE',  ( 0.000000000000000000, 0.000000000000000000, 1.000000000000000000 ) ) ;
#4975=FACE_OUTER_BOUND ( 'NONE', #21712, .T. ) ;
#4978=CARTESIAN_POINT ( 'NONE',  ( -14.66655470856257182, 20.08105443166860127, 10.49999999999999822 ) ) ;
#4981=FACE_OUTER_BOUND ( 'NONE', #2852, .T. ) ;
#4984=DIRECTION ( 'NONE',  ( 0.3090169943749465631, -0.9510565162951538642, 0.000000000000000000 ) ) ;
#4986=CARTESIAN_POINT ( 'NONE',  ( -13.05736835487441994, 16.11602540378456183, 7.499999999999993783 ) ) ;
#4990=ORIENTED_EDGE ( 'NONE', *, *, #37543, .F. ) ;
#4998=ORIENTED_EDGE ( 'NONE', *, *, #13100, .F. ) ;
#5000=CYLINDRICAL_SURFACE ( 'NONE', #23854, 0.5000000000000004441 ) ;
#5001=LINE ( 'NONE', #8247, #36135 ) ;
#5002=FACE_OUTER_BOUND ( 'NONE', #23601, .T. ) ;
#5007=DIRECTION ( 'NONE',  ( 0.000000000000000000, -0.000000000000000000, 1.000000000000000000 ) ) ;
#5008=CARTESIAN_POINT ( 'NONE',  ( -14.45538749008468038, 26.50521816028845734, 7.489440493383480835 ) ) ;
#5010=AXIS2_PLACEMENT_3D ( 'NONE', #31976, #20198, #28927 ) ;
#5011=VECTOR ( 'NONE', #31034, 1000.000000000000114 ) ;
#5012=EDGE_CURVE ( 'NONE', #20519, #15902, #20814, .T. ) ;
#5013=ORIENTED_EDGE ( 'NONE', *, *, #571, .T. ) ;
#5016=VECTOR ( 'NONE', #7409, 1000.000000000000114 ) ;
#5017=CARTESIAN_POINT ( 'NONE',  ( 16.38619327006176718, 7.072988944186808347, 11.00000000000000000 ) ) ;
#5018=LINE ( 'NONE', #17429, #13189 ) ;
#5021=DIRECTION ( 'NONE',  ( 0.5877852522924796874, 0.8090169943749426773, -0.000000000000000000 ) ) ;
#5022=CARTESIAN_POINT ( 'NONE',  ( 8.411683849014126579, 19.76687823897103868, 9.000000000000001776 ) ) ;
#5023=EDGE_CURVE ( 'NONE', #19849, #1872, #39691, .T. ) ;
#5024=CARTESIAN_POINT ( 'NONE',  ( -5.947717410344452560, 34.62949535663727829, 7.000000000000000000 ) ) ;
#5025=CARTESIAN_POINT ( 'NONE',  ( 11.94134295108989896, 16.18301270189217433, 10.50000000000000000 ) ) ;
#5026=CARTESIAN_POINT ( 'NONE',  ( 9.427394962683440127, 11.06314620782477753, 10.49999999999999822 ) ) ;
#5028=CARTESIAN_POINT ( 'NONE',  ( -6.572794801194226544, 16.58182897866500127, 7.000000000000000000 ) ) ;
#5029=ORIENTED_EDGE ( 'NONE', *, *, #29518, .T. ) ;
#5031=DIRECTION ( 'NONE',  ( 1.000000000000000000, 0.000000000000000000, 0.000000000000000000 ) ) ;
#5032=CARTESIAN_POINT ( 'NONE',  ( -9.831584923911588447, 26.22020669908463830, 11.00000000000000000 ) ) ;
#5037=CARTESIAN_POINT ( 'NONE',  ( -19.23557158514982746, 34.18301270189230934, 11.00000000000000000 ) ) ;
#5038=AXIS2_PLACEMENT_3D ( 'NONE', #27236, #20552, #8549 ) ;
#5044=DIRECTION ( 'NONE',  ( 1.000000000000000000, 0.000000000000000000, 0.000000000000000000 ) ) ;
#5045=EDGE_CURVE ( 'NONE', #11442, #7975, #40083, .T. ) ;
#5048=AXIS2_PLACEMENT_3D ( 'NONE', #16760, #16152, #4561 ) ;
#5049=ORIENTED_EDGE ( 'NONE', *, *, #12811, .T. ) ;
#5051=CARTESIAN_POINT ( 'NONE',  ( -14.61785853667976554, 5.591280219786782801, 9.500000000000000000 ) ) ;
#5052=ORIENTED_EDGE ( 'NONE', *, *, #28478, .T. ) ;
#5053=CARTESIAN_POINT ( 'NONE',  ( 10.54700836463452340, 22.39697303105787540, 10.50000000000000355 ) ) ;
#5054=LINE ( 'NONE', #26991, #17436 ) ;
#5057=ORIENTED_EDGE ( 'NONE', *, *, #23647, .F. ) ;
#5060=CARTESIAN_POINT ( 'NONE',  ( -0.4999999999999998890, 37.44611345180491213, 10.76099332938163755 ) ) ;
#5062=VECTOR ( 'NONE', #1848, 1000.000000000000114 ) ;
#5064=DIRECTION ( 'NONE',  ( -0.5877852522924690293, 0.8090169943749503378, -0.000000000000000000 ) ) ;
#5065=ADVANCED_FACE ( 'NONE', ( #36451 ), #27499, .T. ) ;
#5066=VECTOR ( 'NONE', #2612, 1000.000000000000000 ) ;
#5067=AXIS2_PLACEMENT_3D ( 'NONE', #31572, #4139, #10648 ) ;
#5071=FACE_OUTER_BOUND ( 'NONE', #22935, .T. ) ;
#5072=CARTESIAN_POINT ( 'NONE',  ( 14.57486473880226185, 26.18419839932902349, 11.00000000000000000 ) ) ;
#5073=EDGE_CURVE ( 'NONE', #12092, #4676, #14974, .T. ) ;
#5074=CIRCLE ( 'NONE', #16092, 1.000000000000014655 ) ;
#5077=AXIS2_PLACEMENT_3D ( 'NONE', #22933, #7083, #19896 ) ;
#5080=LINE ( 'NONE', #14419, #12544 ) ;
#5081=FACE_OUTER_BOUND ( 'NONE', #11146, .T. ) ;
#5088=EDGE_CURVE ( 'NONE', #22937, #30242, #17971, .T. ) ;
#5089=DIRECTION ( 'NONE',  ( 0.3090169943749573322, 0.9510565162951504226, -0.000000000000000000 ) ) ;
#5090=EDGE_CURVE ( 'NONE', #3614, #1872, #6158, .T. ) ;
#5091=VERTEX_POINT ( 'NONE', #5959 ) ;
#5094=LINE ( 'NONE', #5292, #37337 ) ;
#5095=DIRECTION ( 'NONE',  ( -0.1045284632676436315, 0.9945218953682742891, 0.000000000000000000 ) ) ;
#5101=CARTESIAN_POINT ( 'NONE',  ( 11.20744270277970855, 31.91841037101594125, 11.00000000000000355 ) ) ;
#5102=FACE_OUTER_BOUND ( 'NONE', #3933, .T. ) ;
#5104=AXIS2_PLACEMENT_3D ( 'NONE', #2526, #39290, #24449 ) ;
#5108=ORIENTED_EDGE ( 'NONE', *, *, #6636, .T. ) ;
#5115=LINE ( 'NONE', #17522, #9812 ) ;
#5119=ORIENTED_EDGE ( 'NONE', *, *, #23443, .T. ) ;
#5120=CARTESIAN_POINT ( 'NONE',  ( 5.473344025737212348, 14.11593743010426394, 10.00000000000000000 ) ) ;
#5125=DIRECTION ( 'NONE',  ( -0.6724985119639661502, -0.2185080122244085765, -0.7071067811865395791 ) ) ;
#5128=CARTESIAN_POINT ( 'NONE',  ( -10.36702044712414938, 31.16169077310601665, 10.00000000000000000 ) ) ;
#5131=CARTESIAN_POINT ( 'NONE',  ( 2.518583951651050867, 7.712953814960687104, 7.499999999999990230 ) ) ;
#5132=EDGE_LOOP ( 'NONE', ( #10626, #13423, #30043, #14936 ) ) ;
#5137=DIRECTION ( 'NONE',  ( -0.6123724356957963577, -0.3535533905932671805, -0.7071067811865491270 ) ) ;
#5145=CARTESIAN_POINT ( 'NONE',  ( 12.30736835487432757, 14.81698729810772441, 11.00000000000000000 ) ) ;
#5146=ADVANCED_FACE ( 'NONE', ( #17780 ), #2527, .T. ) ;
#5147=ORIENTED_EDGE ( 'NONE', *, *, #4164, .T. ) ;
#5151=EDGE_LOOP ( 'NONE', ( #28880, #36655, #18979, #36838 ) ) ;
#5158=CIRCLE ( 'NONE', #12286, 0.4999999999999988898 ) ;
#5162=CIRCLE ( 'NONE', #27861, 1.000000000000004441 ) ;
#5164=ADVANCED_FACE ( 'NONE', ( #27102 ), #11865, .T. ) ;
#5165=CARTESIAN_POINT ( 'NONE',  ( -13.47830981910552772, 21.58612669357095015, 9.500000000000000000 ) ) ;
#5166=DIRECTION ( 'NONE',  ( -0.000000000000000000, 0.000000000000000000, -1.000000000000000000 ) ) ;
#5167=ADVANCED_FACE ( 'NONE', ( #24254 ), #36649, .F. ) ;
#5168=EDGE_CURVE ( 'NONE', #34341, #15686, #31817, .T. ) ;
#5169=DIRECTION ( 'NONE',  ( -0.000000000000000000, -0.000000000000000000, -1.000000000000000000 ) ) ;
#5171=DIRECTION ( 'NONE',  ( 0.7071067811865500152, 0.000000000000000000, -0.7071067811865450192 ) ) ;
#5174=CARTESIAN_POINT ( 'NONE',  ( -9.665073660138977729, 25.11464168560200250, 10.50000000000000000 ) ) ;
#5177=DIRECTION ( 'NONE',  ( 1.000000000000000000, 1.734723475976793684E-15, 0.000000000000000000 ) ) ;
#5178=CARTESIAN_POINT ( 'NONE',  ( 12.19134295108989718, 16.61602540378438775, 9.500000000000000000 ) ) ;
#5181=CIRCLE ( 'NONE', #23367, 15.00000000000000000 ) ;
#5182=ORIENTED_EDGE ( 'NONE', *, *, #13464, .F. ) ;
#5188=CARTESIAN_POINT ( 'NONE',  ( -14.70895476143393488, 21.92515157238299039, 10.49999999999999822 ) ) ;
#5189=CIRCLE ( 'NONE', #27892, 15.00000000000000000 ) ;
#5193=ADVANCED_FACE ( 'NONE', ( #6745 ), #38039, .T. ) ;
#5205=DIRECTION ( 'NONE',  ( 0.6216356077939589886, 0.000000000000000000, -0.7833065626704751594 ) ) ;
#5206=ORIENTED_EDGE ( 'NONE', *, *, #19689, .F. ) ;
#5211=DIRECTION ( 'NONE',  ( -0.000000000000000000, -0.000000000000000000, -1.000000000000000000 ) ) ;
#5212=SURFACE_STYLE_USAGE ( .BOTH. , #1980 ) ;
#5213=EDGE_CURVE ( 'NONE', #1404, #39240, #34398, .T. ) ;
#5217=AXIS2_PLACEMENT_3D ( 'NONE', #32609, #2875, #4767 ) ;
#5218=DIRECTION ( 'NONE',  ( 1.000000000000000000, 0.000000000000000000, 0.000000000000000000 ) ) ;
#5220=DIRECTION ( 'NONE',  ( 0.7771459614569634633, -0.6293203910498466058, 2.315526266344420400E-15 ) ) ;
#5223=DIRECTION ( 'NONE',  ( 0.000000000000000000, 0.000000000000000000, 1.000000000000000000 ) ) ;
#5224=CARTESIAN_POINT ( 'NONE',  ( 5.440908595777817602, 35.94977745735560859, 7.000000000000000000 ) ) ;
#5225=CARTESIAN_POINT ( 'NONE',  ( 7.659620408498160060, 26.92228390473674793, 9.000000000000001776 ) ) ;
#5226=DIRECTION ( 'NONE',  ( 0.000000000000000000, 0.000000000000000000, 1.000000000000000000 ) ) ;
#5227=CARTESIAN_POINT ( 'NONE',  ( 3.000488737323008248, 30.46850471149999962, 9.000000000000001776 ) ) ;
#5229=DIRECTION ( 'NONE',  ( 0.9135454576426004225, -0.4067366430758009854, 0.000000000000000000 ) ) ;
#5230=ORIENTED_EDGE ( 'NONE', *, *, #7321, .F. ) ;
#5231=AXIS2_PLACEMENT_3D ( 'NONE', #28692, #19549, #13450 ) ;
#5233=CARTESIAN_POINT ( 'NONE',  ( -7.096882951594430722, 29.56287847632736288, 10.49999999999999822 ) ) ;
#5234=CARTESIAN_POINT ( 'NONE',  ( -1.000000000000000444, 37.00000000000000711, 10.49999999999999822 ) ) ;
#5235=AXIS2_PLACEMENT_3D ( 'NONE', #9269, #24703, #21653 ) ;
#5238=B_SPLINE_CURVE_WITH_KNOTS ( 'NONE', 3,
 ( #31058, #18665, #379, #16012, #15812, #12757 ),
 .UNSPECIFIED., .F., .F.,
 ( 4, 2, 4 ),
 ( 0.000000000000000000, 0.3000000000367072928, 0.6000000000734145855 ),
 .UNSPECIFIED. ) ;
#5240=CARTESIAN_POINT ( 'NONE',  ( 9.831584923911636409, 26.22020669908449975, 10.00000000000000000 ) ) ;
#5246=CARTESIAN_POINT ( 'NONE',  ( 0.5000000000000001110, 37.00000000000000711, 11.00000000000000000 ) ) ;
#5247=EDGE_CURVE ( 'NONE', #30411, #17610, #30558, .T. ) ;
#5248=VERTEX_POINT ( 'NONE', #18954 ) ;
#5251=CARTESIAN_POINT ( 'NONE',  ( 5.537946624086096392, 36.44027069998188750, 7.500000000000000888 ) ) ;
#5253=DIRECTION ( 'NONE',  ( 0.2876062384759510704, 0.6459741880212550580, -0.7071067811865435759 ) ) ;
#5254=FACE_OUTER_BOUND ( 'NONE', #17209, .T. ) ;
#5255=ORIENTED_EDGE ( 'NONE', *, *, #11339, .T. ) ;
#5259=CIRCLE ( 'NONE', #6548, 0.4999999999999995559 ) ;
#5261=ORIENTED_EDGE ( 'NONE', *, *, #27749, .T. ) ;
#5262=CARTESIAN_POINT ( 'NONE',  ( -0.4999999999999995559, 37.00000000000000711, 11.00000000000000000 ) ) ;
#5263=EDGE_LOOP ( 'NONE', ( #265, #23594, #32859, #9443 ) ) ;
#5264=DIRECTION ( 'NONE',  ( 0.4999999999999933942, -0.8660254037844425934, 0.000000000000000000 ) ) ;
#5265=DIRECTION ( 'NONE',  ( 0.5254827454987650581, -0.4731467892558172683, -0.7071067811865414665 ) ) ;
#5267=ORIENTED_EDGE ( 'NONE', *, *, #33008, .F. ) ;
#5268=CARTESIAN_POINT ( 'NONE',  ( 6.354454053420413473, 35.54304081427980577, 11.00000000000000000 ) ) ;
#5269=CARTESIAN_POINT ( 'NONE',  ( 2.036571916123615100, 8.108948098542045457, 10.49999999999999467 ) ) ;
#5270=ADVANCED_FACE ( 'NONE', ( #12657 ), #25050, .T. ) ;
#5272=DIRECTION ( 'NONE',  ( 0.9945218953682727347, -0.1045284632676597436, -3.469446951953608667E-15 ) ) ;
#5277=DIRECTION ( 'NONE',  ( -0.3090169943749457304, 0.9510565162951540863, 0.000000000000000000 ) ) ;
#5278=CARTESIAN_POINT ( 'NONE',  ( -13.16028273094462975, 27.30176617939698147, 9.500000000000000000 ) ) ;
#5283=VECTOR ( 'NONE', #25347, 1000.000000000000114 ) ;
#5286=VECTOR ( 'NONE', #38388, 1000.000000000000000 ) ;
#5287=ADVANCED_FACE ( 'NONE', ( #16308 ), #25248, .T. ) ;
#5288=CARTESIAN_POINT ( 'NONE',  ( 11.44473057578109021, 31.45924896672603310, 10.49999999999999822 ) ) ;
#5292=CARTESIAN_POINT ( 'NONE',  ( -13.62380822250706736, 25.87518140495425101, 9.500000000000000000 ) ) ;
#5293=ADVANCED_FACE ( 'NONE', ( #21999 ), #4107, .T. ) ;
#5294=DIRECTION ( 'NONE',  ( -0.7032331762534049791, 0.07391278520358846027, -0.7071067811865444641 ) ) ;
#5295=FACE_OUTER_BOUND ( 'NONE', #6973, .T. ) ;
#5296=EDGE_LOOP ( 'NONE', ( #23160, #17802, #16395, #37290 ) ) ;
#5299=DIRECTION ( 'NONE',  ( 1.000000000000000000, 0.000000000000000000, 0.000000000000000000 ) ) ;
#5300=FACE_OUTER_BOUND ( 'NONE', #19706, .T. ) ;
#5301=CARTESIAN_POINT ( 'NONE',  ( -2.061816823438740620, 8.019625857904001620, 10.49999999999999822 ) ) ;
#5302=ADVANCED_FACE ( 'NONE', ( #868 ), #18760, .F. ) ;
#5305=CARTESIAN_POINT ( 'NONE',  ( -5.517564457587356586, 36.12194934191566631, 10.96580508970282430 ) ) ;
#5306=ORIENTED_EDGE ( 'NONE', *, *, #9261, .T. ) ;
#5309=ORIENTED_EDGE ( 'NONE', *, *, #34978, .F. ) ;
#5311=DIRECTION ( 'NONE',  ( 0.000000000000000000, 0.000000000000000000, 1.000000000000000000 ) ) ;
#5312=LINE ( 'NONE', #11810, #29907 ) ;
#5314=LINE ( 'NONE', #29896, #18131 ) ;
#5316=DIRECTION ( 'NONE',  ( 1.000000000000000000, 0.000000000000000000, 0.000000000000000000 ) ) ;
#5317=EDGE_CURVE ( 'NONE', #17826, #34540, #13248, .T. ) ;
#5318=CARTESIAN_POINT ( 'NONE',  ( -8.927394655428429360, 11.06314620770957013, 7.500000000000000888 ) ) ;
#5319=EDGE_CURVE ( 'NONE', #3128, #6055, #19150, .T. ) ;
#5323=VECTOR ( 'NONE', #29632, 1000.000000000000227 ) ;
#5332=VECTOR ( 'NONE', #10036, 1000.000000000000000 ) ;
#5336=VERTEX_POINT ( 'NONE', #25436 ) ;
#5340=CARTESIAN_POINT ( 'NONE',  ( -9.468266739736646898, 17.89951905283841782, 10.74999999999999822 ) ) ;
#5342=ADVANCED_FACE ( 'NONE', ( #666 ), #13047, .F. ) ;
#5343=DIRECTION ( 'NONE',  ( -0.7071067811865524577, 0.000000000000000000, -0.7071067811865426878 ) ) ;
#5349=VERTEX_POINT ( 'NONE', #31746 ) ;
#5351=PLANE ( 'NONE',  #17417 ) ;
#5353=EDGE_LOOP ( 'NONE', ( #24730, #19339, #20809, #22845 ) ) ;
#5355=ORIENTED_EDGE ( 'NONE', *, *, #22653, .F. ) ;
#5358=EDGE_LOOP ( 'NONE', ( #9191, #9766, #40103, #27292 ) ) ;
#5359=AXIS2_PLACEMENT_3D ( 'NONE', #14330, #14531, #11689 ) ;
#5363=VECTOR ( 'NONE', #38421, 1000.000000000000000 ) ;
#5366=DIRECTION ( 'NONE',  ( -0.9135454576426071949, -0.4067366430757861639, 0.000000000000000000 ) ) ;
#5368=DIRECTION ( 'NONE',  ( 0.6037757019622813637, 0.000000000000000000, 0.7971542521494534572 ) ) ;
#5369=ORIENTED_EDGE ( 'NONE', *, *, #22039, .T. ) ;
#5371=DIRECTION ( 'NONE',  ( -0.5000000000000041078, -0.8660254037844362651, 0.000000000000000000 ) ) ;
#5375=CARTESIAN_POINT ( 'NONE',  ( -14.40879062396297883, 19.98622263052321557, 10.49999999999999822 ) ) ;
#5379=EDGE_LOOP ( 'NONE', ( #954, #17255, #39948, #14445, #27629 ) ) ;
#5383=DIRECTION ( 'NONE',  ( -0.000000000000000000, -0.000000000000000000, -1.000000000000000000 ) ) ;
#5385=EDGE_LOOP ( 'NONE', ( #16291, #21565, #14687, #13936 ) ) ;
#5386=CARTESIAN_POINT ( 'NONE',  ( -14.94248101481484170, 21.43223609974793220, 10.68306085400105587 ) ) ;
#5387=ORIENTED_EDGE ( 'NONE', *, *, #1461, .T. ) ;
#5391=EDGE_CURVE ( 'NONE', #31473, #16736, #9901, .T. ) ;
#5392=LINE ( 'NONE', #21037, #9419 ) ;
#5393=VECTOR ( 'NONE', #29957, 1000.000000000000114 ) ;
#5398=VERTEX_POINT ( 'NONE', #35399 ) ;
#5399=EDGE_CURVE ( 'NONE', #10247, #22927, #1272, .T. ) ;
#5401=LINE ( 'NONE', #17814, #15419 ) ;
#5403=CARTESIAN_POINT ( 'NONE',  ( 7.766013557953383106, 28.81973365084986938, 10.50000000000000178 ) ) ;
#5404=ORIENTED_EDGE ( 'NONE', *, *, #14822, .F. ) ;
#5406=VECTOR ( 'NONE', #1129, 1000.000000000000000 ) ;
#5408=ADVANCED_FACE ( 'NONE', ( #26044 ), #29269, .T. ) ;
#5409=DIRECTION ( 'NONE',  ( -0.1045284632676569680, -0.9945218953682729568, 0.000000000000000000 ) ) ;
#5412=AXIS2_PLACEMENT_3D ( 'NONE', #35894, #38937, #20461 ) ;
#5416=EDGE_CURVE ( 'NONE', #24423, #17070, #5259, .T. ) ;
#5420=ADVANCED_FACE ( 'NONE', ( #13860 ), #34460, .T. ) ;
#5425=CARTESIAN_POINT ( 'NONE',  ( -2.568190708544568768, 12.82247983807084957, 10.00000000000000000 ) ) ;
#5426=FACE_OUTER_BOUND ( 'NONE', #21592, .T. ) ;
#5427=FACE_OUTER_BOUND ( 'NONE', #27942, .T. ) ;
#5429=CARTESIAN_POINT ( 'NONE',  ( 12.74038105676654631, 14.56698729810772264, 10.63089969389957545 ) ) ;
#5432=FACE_OUTER_BOUND ( 'NONE', #2471, .T. ) ;
#5433=ORIENTED_EDGE ( 'NONE', *, *, #39892, .T. ) ;
#5435=CARTESIAN_POINT ( 'NONE',  ( 13.63581098909226874, 27.45627467658428955, 7.500000000000000888 ) ) ;
#5436=AXIS2_PLACEMENT_3D ( 'NONE', #36848, #21799, #34202 ) ;
#5437=LINE ( 'NONE', #33682, #14673 ) ;
#5439=LINE ( 'NONE', #5836, #8100 ) ;
#5441=PLANE ( 'NONE',  #28293 ) ;
#5443=EDGE_CURVE ( 'NONE', #32345, #22086, #17528, .T. ) ;
#5444=AXIS2_PLACEMENT_3D ( 'NONE', #34904, #37751, #19455 ) ;
#5448=ADVANCED_FACE ( 'NONE', ( #4314 ), #35604, .T. ) ;
#5450=DIRECTION ( 'NONE',  ( 0.6691306063588570163, -0.7431448254773953543, 0.000000000000000000 ) ) ;
#5452=VERTEX_POINT ( 'NONE', #1883 ) ;
#5453=LINE ( 'NONE', #27383, #36484 ) ;
#5454=ORIENTED_EDGE ( 'NONE', *, *, #16612, .F. ) ;
#5455=CARTESIAN_POINT ( 'NONE',  ( -15.24159360913302841, 8.525723021988211414, 10.00000000000000000 ) ) ;
#5456=CARTESIAN_POINT ( 'NONE',  ( 9.221287281574577221, 10.65863771052202935, 10.59344459855561738 ) ) ;
#5459=EDGE_LOOP ( 'NONE', ( #30077, #15142, #27697, #17278 ) ) ;
#5460=CARTESIAN_POINT ( 'NONE',  ( 9.831584923911634633, 26.22020669908450330, 10.00000000000000000 ) ) ;
#5461=EDGE_LOOP ( 'NONE', ( #23085, #2790, #25221, #22650, #9490 ) ) ;
#5462=DIRECTION ( 'NONE',  ( 0.8660254037844424824, 0.4999999999999932832, 0.000000000000000000 ) ) ;
#5463=CARTESIAN_POINT ( 'NONE',  ( 12.68475447279711510, 27.14725768220934299, 10.00000000000000000 ) ) ;
#5465=DIRECTION ( 'NONE',  ( 0.9135454576425988682, -0.4067366430758048157, 0.000000000000000000 ) ) ;
#5467=DIRECTION ( 'NONE',  ( -1.000000000000000000, 0.000000000000000000, 0.000000000000000000 ) ) ;
#5468=FACE_OUTER_BOUND ( 'NONE', #34879, .T. ) ;
#5472=EDGE_LOOP ( 'NONE', ( #4449, #8392, #18116, #11593, #2574 ) ) ;
#5483=ORIENTED_EDGE ( 'NONE', *, *, #17328, .F. ) ;
#5484=EDGE_CURVE ( 'NONE', #10090, #2692, #16956, .T. ) ;
#5487=LINE ( 'NONE', #20139, #20468 ) ;
#5488=LINE ( 'NONE', #20750, #28241 ) ;
#5489=DIRECTION ( 'NONE',  ( 0.000000000000000000, 0.000000000000000000, 1.000000000000000000 ) ) ;
#5492=CARTESIAN_POINT ( 'NONE',  ( -8.737320611644010526, -1.152986690174108819, 7.499999999999999112 ) ) ;
#5497=DIRECTION ( 'NONE',  ( -0.5000000000000038858, -0.8660254037844364872, 0.000000000000000000 ) ) ;
#5500=AXIS2_PLACEMENT_3D ( 'NONE', #17480, #17280, #32517 ) ;
#5504=LINE ( 'NONE', #10681, #33421 ) ;
#5505=CARTESIAN_POINT ( 'NONE',  ( -5.644276917315532494, 36.40655018617699312, 10.50000000000000000 ) ) ;
#5508=VERTEX_POINT ( 'NONE', #32562 ) ;
#5510=DIRECTION ( 'NONE',  ( 1.000000000000000000, 0.000000000000000000, 0.000000000000000000 ) ) ;
#5512=AXIS2_PLACEMENT_3D ( 'NONE', #13222, #32123, #13829 ) ;
#5515=EDGE_CURVE ( 'NONE', #36822, #2452, #7958, .T. ) ;
#5520=AXIS2_PLACEMENT_3D ( 'NONE', #7013, #19615, #7623 ) ;
#5521=CARTESIAN_POINT ( 'NONE',  ( 8.118377661053324701, 10.47536095541698486, 7.000000000000000000 ) ) ;
#5522=CARTESIAN_POINT ( 'NONE',  ( -0.6108529249776363246, 37.48755679569042343, 7.000000000000000000 ) ) ;
#5523=ORIENTED_EDGE ( 'NONE', *, *, #11997, .F. ) ;
#5526=AXIS2_PLACEMENT_3D ( 'NONE', #5866, #39988, #27805 ) ;
#5530=CARTESIAN_POINT ( 'NONE',  ( -14.19304739008513927, 26.58586953448673285, 10.94611345180490147 ) ) ;
#5534=ORIENTED_EDGE ( 'NONE', *, *, #16258, .T. ) ;
#5536=DIRECTION ( 'NONE',  ( 0.3535533905932645160, -0.6123724356958055726, 0.7071067811865425767 ) ) ;
#5538=DIRECTION ( 'NONE',  ( -0.8090169943749510040, -0.5877852522924683631, -3.469446951953612611E-15 ) ) ;
#5545=FACE_OUTER_BOUND ( 'NONE', #14274, .T. ) ;
#5548=EDGE_CURVE ( 'NONE', #11555, #28022, #9144, .T. ) ;
#5549=ORIENTED_EDGE ( 'NONE', *, *, #25174, .F. ) ;
#5551=ORIENTED_EDGE ( 'NONE', *, *, #9813, .T. ) ;
#5560=VECTOR ( 'NONE', #5095, 1000.000000000000114 ) ;
#5562=CARTESIAN_POINT ( 'NONE',  ( -8.927394655428429360, 11.06314620770957013, 11.00000000000000000 ) ) ;
#5563=ADVANCED_FACE ( 'NONE', ( #19754 ), #32150, .F. ) ;
#5565=CARTESIAN_POINT ( 'NONE',  ( 14.47283171447379502, 21.48159823030311344, 7.000000000000000000 ) ) ;
#5566=ORIENTED_EDGE ( 'NONE', *, *, #18532, .T. ) ;
#5568=CARTESIAN_POINT ( 'NONE',  ( 8.843266739736572291, 16.81698729810774395, 10.50000000000000000 ) ) ;
#5569=FACE_OUTER_BOUND ( 'NONE', #16070, .T. ) ;
#5571=CARTESIAN_POINT ( 'NONE',  ( -8.633502029282189127, 11.46765470489704342, 7.499999999999999112 ) ) ;
#5574=ORIENTED_EDGE ( 'NONE', *, *, #9889, .F. ) ;
#5577=CARTESIAN_POINT ( 'NONE',  ( 10.36702044712426662, 31.16169077310587809, 7.000000000000000000 ) ) ;
#5579=VERTEX_POINT ( 'NONE', #18516 ) ;
#5582=AXIS2_PLACEMENT_3D ( 'NONE', #2644, #2451, #39611 ) ;
#5587=VECTOR ( 'NONE', #3076, 1000.000000000000000 ) ;
#5588=VECTOR ( 'NONE', #23769, 1000.000000000000114 ) ;
#5593=VERTEX_POINT ( 'NONE', #11623 ) ;
#5595=CIRCLE ( 'NONE', #28295, 5.999999999999994671 ) ;
#5596=DIRECTION ( 'NONE',  ( -0.6724985119639655951, -0.2185080122244103806, -0.7071067811865396902 ) ) ;
#5597=ADVANCED_FACE ( 'NONE', ( #36403 ), #2674, .T. ) ;
#5599=EDGE_CURVE ( 'NONE', #19098, #37418, #37000, .T. ) ;
#5600=DIRECTION ( 'NONE',  ( 0.4999999999999920064, -0.8660254037844432595, 0.000000000000000000 ) ) ;
#5601=VERTEX_POINT ( 'NONE', #2481 ) ;
#5604=LINE ( 'NONE', #33462, #15066 ) ;
#5607=CARTESIAN_POINT ( 'NONE',  ( 14.09933648065468503, 26.02968990214155198, 11.00000000000000000 ) ) ;
#5608=ORIENTED_EDGE ( 'NONE', *, *, #20532, .F. ) ;
#5609=DIRECTION ( 'NONE',  ( -0.2876062384759389134, 0.6459741880212461762, -0.7071067811865567876 ) ) ;
#5610=EDGE_CURVE ( 'NONE', #36997, #24077, #27059, .T. ) ;
#5611=CARTESIAN_POINT ( 'NONE',  ( 6.431109915230138085, 35.71521269883979244, 10.96580508970282963 ) ) ;
#5614=LINE ( 'NONE', #2381, #982 ) ;
#5616=CARTESIAN_POINT ( 'NONE',  ( 10.54700836463452340, 22.39697303105787540, 10.50000000000000000 ) ) ;
#5617=EDGE_CURVE ( 'NONE', #15610, #11440, #21553, .T. ) ;
#5618=CARTESIAN_POINT ( 'NONE',  ( -14.52509594610762456, 21.97885917798744870, 7.500000000000004441 ) ) ;
#5620=DIRECTION ( 'NONE',  ( 0.000000000000000000, 0.000000000000000000, -1.000000000000000000 ) ) ;
#5621=DIRECTION ( 'NONE',  ( 0.000000000000000000, 0.000000000000000000, -1.000000000000000000 ) ) ;
#5624=ORIENTED_EDGE ( 'NONE', *, *, #24737, .T. ) ;
#5626=CARTESIAN_POINT ( 'NONE',  ( 13.16028273094469014, 27.30176617939681449, 9.500000000000000000 ) ) ;
#5631=ORIENTED_EDGE ( 'NONE', *, *, #2415, .F. ) ;
#5633=PLANE ( 'NONE',  #38885 ) ;
#5638=DIRECTION ( 'NONE',  ( -0.000000000000000000, -0.000000000000000000, -1.000000000000000000 ) ) ;
#5641=EDGE_LOOP ( 'NONE', ( #23166, #39721, #26480, #2895, #38662 ) ) ;
#5642=EDGE_CURVE ( 'NONE', #14093, #28389, #1368, .T. ) ;
#5643=VECTOR ( 'NONE', #3442, 1000.000000000000000 ) ;
#5648=FACE_OUTER_BOUND ( 'NONE', #15205, .T. ) ;
#5651=CIRCLE ( 'NONE', #31597, 0.5000000000000004441 ) ;
#5652=ORIENTED_EDGE ( 'NONE', *, *, #17367, .F. ) ;
#5655=ORIENTED_EDGE ( 'NONE', *, *, #6911, .F. ) ;
#5656=CARTESIAN_POINT ( 'NONE',  ( 13.95683075005237050, 28.08631143191933432, 7.000000000000000000 ) ) ;
#5658=EDGE_CURVE ( 'NONE', #14950, #31717, #8565, .T. ) ;
#5659=CARTESIAN_POINT ( 'NONE',  ( -4.003793312560516071, 8.307369216259115063, 10.49999999999999822 ) ) ;
#5660=EDGE_LOOP ( 'NONE', ( #1265, #23940, #6848, #24124 ) ) ;
#5661=ADVANCED_FACE ( 'NONE', ( #6110 ), #20773, .T. ) ;
#5662=CARTESIAN_POINT ( 'NONE',  ( -3.503793317224520365, 8.420815634768723967, 11.00000000000000000 ) ) ;
#5664=DIRECTION ( 'NONE',  ( -0.1045284632676437703, 0.9945218953682745111, 0.000000000000000000 ) ) ;
#5667=CIRCLE ( 'NONE', #5010, 0.5000000000000006661 ) ;
#5669=AXIS2_PLACEMENT_3D ( 'NONE', #15191, #5450, #30033 ) ;
#5670=VERTEX_POINT ( 'NONE', #27254 ) ;
#5673=DIRECTION ( 'NONE',  ( -1.000000000000000000, 0.000000000000000000, 0.000000000000000000 ) ) ;
#5674=CYLINDRICAL_SURFACE ( 'NONE', #17931, 0.4999999999999995559 ) ;
#5676=DIRECTION ( 'NONE',  ( 0.7431448254773953543, 0.6691306063588570163, 0.000000000000000000 ) ) ;
#5677=CIRCLE ( 'NONE', #39403, 0.4999999999999995559 ) ;
#5679=AXIS2_PLACEMENT_3D ( 'NONE', #17816, #20047, #35687 ) ;
#5683=CARTESIAN_POINT ( 'NONE',  ( 11.61146752755227141, 31.78078372435978594, 10.49999999999999822 ) ) ;
#5685=ORIENTED_EDGE ( 'NONE', *, *, #2698, .F. ) ;
#5688=CARTESIAN_POINT ( 'NONE',  ( -3.914034194965524183, 30.06176806842423943, 9.000000000000001776 ) ) ;
#5689=CARTESIAN_POINT ( 'NONE',  ( 5.947717410344610656, 34.62949535663720724, 9.500000000000000000 ) ) ;
#5690=EDGE_CURVE ( 'NONE', #6428, #37593, #23447, .T. ) ;
#5691=CARTESIAN_POINT ( 'NONE',  ( -9.221287281574664263, 10.65863771052210396, 10.49999999999999645 ) ) ;
#5692=ORIENTED_EDGE ( 'NONE', *, *, #10041, .T. ) ;
#5694=DIRECTION ( 'NONE',  ( 1.000000000000000000, 0.000000000000000000, 0.000000000000000000 ) ) ;
#5695=DIRECTION ( 'NONE',  ( -0.9135454576426004225, 0.4067366430758009854, 0.000000000000000000 ) ) ;
#5696=AXIS2_PLACEMENT_3D ( 'NONE', #5037, #30231, #39960 ) ;
#5697=ORIENTED_EDGE ( 'NONE', *, *, #38236, .F. ) ;
#5699=FACE_OUTER_BOUND ( 'NONE', #2209, .T. ) ;
#5707=AXIS2_PLACEMENT_3D ( 'NONE', #1219, #19494, #31888 ) ;
#5708=CARTESIAN_POINT ( 'NONE',  ( 0.000000000000000000, 22.50000000000000355, 7.000000000000000000 ) ) ;
#5711=AXIS2_PLACEMENT_3D ( 'NONE', #17509, #24184, #11604 ) ;
#5712=CARTESIAN_POINT ( 'NONE',  ( 1.828660225305861475, 9.087095699275852922, 9.500000000000000000 ) ) ;
#5713=ORIENTED_EDGE ( 'NONE', *, *, #31638, .T. ) ;
#5714=ADVANCED_FACE ( 'NONE', ( #17730 ), #30106, .T. ) ;
#5718=FACE_OUTER_BOUND ( 'NONE', #31189, .T. ) ;
#5726=VECTOR ( 'NONE', #8095, 1000.000000000000114 ) ;
#5727=ORIENTED_EDGE ( 'NONE', *, *, #34094, .T. ) ;
#5729=VECTOR ( 'NONE', #15893, 1000.000000000000000 ) ;
#5732=CARTESIAN_POINT ( 'NONE',  ( -14.42035624161473883, 26.65972665747678860, 10.49999999999999822 ) ) ;
#5739=CARTESIAN_POINT ( 'NONE',  ( 8.258442077957491634, 10.28257882428873771, 10.94387467463492136 ) ) ;
#5742=AXIS2_PLACEMENT_3D ( 'NONE', #34487, #9505, #18651 ) ;
#5743=ORIENTED_EDGE ( 'NONE', *, *, #12137, .F. ) ;
#5746=CARTESIAN_POINT ( 'NONE',  ( 13.77067693704748308, 28.44713853003850801, 7.000000000000000000 ) ) ;
#5747=ORIENTED_EDGE ( 'NONE', *, *, #37150, .F. ) ;
#5749=CARTESIAN_POINT ( 'NONE',  ( -1.000000000000000000, 37.50000000000000711, 11.00000000000000000 ) ) ;
#5751=EDGE_CURVE ( 'NONE', #4123, #29026, #18316, .T. ) ;
#5754=ORIENTED_EDGE ( 'NONE', *, *, #13036, .T. ) ;
#5757=ORIENTED_EDGE ( 'NONE', *, *, #26410, .T. ) ;
#5763=VECTOR ( 'NONE', #24118, 1000.000000000000000 ) ;
#5764=DIRECTION ( 'NONE',  ( 1.000000000000000000, 0.000000000000000000, 0.000000000000000000 ) ) ;
#5766=LINE ( 'NONE', #33420, #13656 ) ;
#5767=AXIS2_PLACEMENT_3D ( 'NONE', #26246, #23204, #32559 ) ;
#5769=FACE_OUTER_BOUND ( 'NONE', #32262, .T. ) ;
#5770=EDGE_LOOP ( 'NONE', ( #17945, #16997, #31115, #16326 ) ) ;
#5772=DIRECTION ( 'NONE',  ( 5.027458560212894738E-15, -0.7071067811865500152, -0.7071067811865450192 ) ) ;
#5782=PLANE ( 'NONE',  #3609 ) ;
#5784=ORIENTED_EDGE ( 'NONE', *, *, #38336, .F. ) ;
#5786=ORIENTED_EDGE ( 'NONE', *, *, #35595, .F. ) ;
#5792=VECTOR ( 'NONE', #11132, 1000.000000000000000 ) ;
#5795=DIRECTION ( 'NONE',  ( 0.000000000000000000, -0.000000000000000000, 1.000000000000000000 ) ) ;
#5797=ORIENTED_EDGE ( 'NONE', *, *, #32081, .F. ) ;
#5799=EDGE_CURVE ( 'NONE', #33798, #21611, #22128, .T. ) ;
#5800=DIRECTION ( 'NONE',  ( -0.9781476007338043566, 0.2079116908177658096, 0.000000000000000000 ) ) ;
#5802=CARTESIAN_POINT ( 'NONE',  ( -22.37798348102460722, 33.25980436007204588, 7.000000000000000000 ) ) ;
#5807=DIRECTION ( 'NONE',  ( 0.4067366430758028728, 0.9135454576425997564, 0.000000000000000000 ) ) ;
#5808=EDGE_CURVE ( 'NONE', #14858, #16847, #26300, .T. ) ;
#5811=DIRECTION ( 'NONE',  ( -0.9135454576426029760, 0.4067366430757954898, 0.000000000000000000 ) ) ;
#5812=CARTESIAN_POINT ( 'NONE',  ( 7.824485034907088021, 10.87986945260446170, 7.499999999999999112 ) ) ;
#5814=CARTESIAN_POINT ( 'NONE',  ( 14.98803198171708218, 21.89746804854020112, 7.339470489435497846 ) ) ;
#5816=PLANE ( 'NONE',  #38295 ) ;
#5817=DIRECTION ( 'NONE',  ( -0.6691306063588570163, 0.7431448254773952433, -0.000000000000000000 ) ) ;
#5819=CARTESIAN_POINT ( 'NONE',  ( 15.02235689379175732, 21.92659494635341844, 7.000000000000000000 ) ) ;
#5821=CARTESIAN_POINT ( 'NONE',  ( 8.118377661053324701, 10.47536095541698486, 7.500000000000000888 ) ) ;
#5823=LINE ( 'NONE', #18223, #14871 ) ;
#5824=AXIS2_PLACEMENT_3D ( 'NONE', #22099, #6261, #15808 ) ;
#5825=DIRECTION ( 'NONE',  ( 0.4067366430758009299, 0.9135454576426005335, 0.000000000000000000 ) ) ;
#5826=CARTESIAN_POINT ( 'NONE',  ( 1.204925152852600378, 12.02153850147727887, 10.50000000000000000 ) ) ;
#5829=CARTESIAN_POINT ( 'NONE',  ( -10.44103466624267185, 32.57396620494226624, 7.000000000000000000 ) ) ;
#5832=PLANE ( 'NONE',  #3181 ) ;
#5836=CARTESIAN_POINT ( 'NONE',  ( 14.84160187385922036, 20.32586711126977619, 7.500000000000010658 ) ) ;
#5838=ORIENTED_EDGE ( 'NONE', *, *, #37633, .T. ) ;
#5840=DIRECTION ( 'NONE',  ( -0.9781476007338043566, 0.2079116908177656708, 0.000000000000000000 ) ) ;
#5845=CARTESIAN_POINT ( 'NONE',  ( 3.813962023474615215, 32.29559562678520024, 10.00000000000000000 ) ) ;
#5849=ADVANCED_FACE ( 'NONE', ( #12411 ), #22544, .T. ) ;
#5850=VECTOR ( 'NONE', #29858, 1000.000000000000000 ) ;
#5853=DIRECTION ( 'NONE',  ( -0.000000000000000000, 0.000000000000000000, 1.000000000000000000 ) ) ;
#5854=PLANE ( 'NONE',  #543 ) ;
#5859=ORIENTED_EDGE ( 'NONE', *, *, #11260, .T. ) ;
#5860=LINE ( 'NONE', #5656, #33992 ) ;
#5863=PLANE ( 'NONE',  #5824 ) ;
#5864=ORIENTED_EDGE ( 'NONE', *, *, #27719, .F. ) ;
#5866=CARTESIAN_POINT ( 'NONE',  ( 8.118377661053324701, 10.47536095541698486, 11.00000000000000000 ) ) ;
#5867=DIRECTION ( 'NONE',  ( -0.6459741880212631626, 0.2876062384759295876, -0.7071067811865451302 ) ) ;
#5868=DIRECTION ( 'NONE',  ( 0.000000000000000000, 0.000000000000000000, 1.000000000000000000 ) ) ;
#5869=B_SPLINE_CURVE_WITH_KNOTS ( 'NONE', 3,
 ( #36475, #8643, #18389, #27526, #24280, #11890 ),
 .UNSPECIFIED., .F., .F.,
 ( 4, 2, 4 ),
 ( 0.000000000000000000, 0.5000000000000000000, 1.000000000000000000 ),
 .UNSPECIFIED. ) ;
#5871=EDGE_CURVE ( 'NONE', #36923, #17177, #20845, .T. ) ;
#5878=CARTESIAN_POINT ( 'NONE',  ( 8.718266739736572291, 16.60048094716163192, 10.74999999999999467 ) ) ;
#5880=CARTESIAN_POINT ( 'NONE',  ( -9.221287281574667816, 10.65863771052209863, 10.49999999999999822 ) ) ;
#5885=ORIENTED_EDGE ( 'NONE', *, *, #22009, .F. ) ;
#5886=ORIENTED_EDGE ( 'NONE', *, *, #18565, .F. ) ;
#5890=DIRECTION ( 'NONE',  ( 0.4067366430758009854, 0.9135454576426005335, 0.000000000000000000 ) ) ;
#5891=CARTESIAN_POINT ( 'NONE',  ( -9.608347198026818248, 2.148595524579384630, 11.00000000000000000 ) ) ;
#5892=ORIENTED_EDGE ( 'NONE', *, *, #11685, .F. ) ;
#5894=ADVANCED_FACE ( 'NONE', ( #229 ), #34953, .T. ) ;
#5895=CONICAL_SURFACE ( 'NONE', #707, 1.000000000000004441, 0.7853981633974583820 ) ;
#5898=ORIENTED_EDGE ( 'NONE', *, *, #8388, .T. ) ;
#5900=LINE ( 'NONE', #21735, #10549 ) ;
#5901=ORIENTED_EDGE ( 'NONE', *, *, #36979, .T. ) ;
#5903=EDGE_CURVE ( 'NONE', #13055, #35073, #31209, .T. ) ;
#5904=VERTEX_POINT ( 'NONE', #21749 ) ;
#5906=VECTOR ( 'NONE', #27405, 1000.000000000000000 ) ;
#5911=VERTEX_POINT ( 'NONE', #34156 ) ;
#5912=LINE ( 'NONE', #12214, #4198 ) ;
#5913=DIRECTION ( 'NONE',  ( -0.9510565162951503115, 0.3090169943749573878, 0.000000000000000000 ) ) ;
#5915=EDGE_CURVE ( 'NONE', #36419, #16093, #5918, .T. ) ;
#5918=CIRCLE ( 'NONE', #1402, 6.000000000000001776 ) ;
#5919=LINE ( 'NONE', #18319, #10109 ) ;
#5922=CARTESIAN_POINT ( 'NONE',  ( -5.400683141673551013, 15.91724817395922997, 9.000000000000001776 ) ) ;
#5929=CIRCLE ( 'NONE', #12425, 1.000000000000004441 ) ;
#5932=ORIENTED_EDGE ( 'NONE', *, *, #21456, .F. ) ;
#5936=CARTESIAN_POINT ( 'NONE',  ( -7.133890061153688400, 30.26901619224549123, 10.50000000000000000 ) ) ;
#5943=EDGE_CURVE ( 'NONE', #22772, #22802, #22153, .T. ) ;
#5944=LINE ( 'NONE', #9197, #20660 ) ;
#5945=CARTESIAN_POINT ( 'NONE',  ( 1.838889047819958655, 31.15129278236397781, 7.000000000000000000 ) ) ;
#5946=EDGE_LOOP ( 'NONE', ( #18149, #14637, #26187, #7315 ) ) ;
#5948=ORIENTED_EDGE ( 'NONE', *, *, #23308, .F. ) ;
#5953=ORIENTED_EDGE ( 'NONE', *, *, #28148, .F. ) ;
#5956=FACE_OUTER_BOUND ( 'NONE', #9030, .T. ) ;
#5958=AXIS2_PLACEMENT_3D ( 'NONE', #794, #28226, #25777 ) ;
#5959=CARTESIAN_POINT ( 'NONE',  ( -9.221287281574667816, 10.65863771052209863, 10.49999999999999822 ) ) ;
#5962=ORIENTED_EDGE ( 'NONE', *, *, #24166, .F. ) ;
#5964=DIRECTION ( 'NONE',  ( 0.000000000000000000, 0.000000000000000000, 1.000000000000000000 ) ) ;
#5965=CARTESIAN_POINT ( 'NONE',  ( 4.577399223880711965, 35.23960032125090436, 10.50000000000000000 ) ) ;
#5967=ADVANCED_FACE ( 'NONE', ( #17281 ), #1629, .T. ) ;
#5974=CARTESIAN_POINT ( 'NONE',  ( -13.16028273094462975, 27.30176617939698147, 7.499999999999994671 ) ) ;
#5976=ORIENTED_EDGE ( 'NONE', *, *, #1870, .T. ) ;
#5978=ORIENTED_EDGE ( 'NONE', *, *, #37651, .F. ) ;
#5980=PLANE ( 'NONE',  #33511 ) ;
#5982=CARTESIAN_POINT ( 'NONE',  ( -10.10646936306323340, 32.94553861768095970, 9.500000000000000000 ) ) ;
#5985=CARTESIAN_POINT ( 'NONE',  ( -11.74460609746112461, 31.83082137946488643, 7.365559175140416137 ) ) ;
#5987=ORIENTED_EDGE ( 'NONE', *, *, #34171, .F. ) ;
#5989=CARTESIAN_POINT ( 'NONE',  ( -7.824485034907249670, 10.87986945260456295, 9.500000000000000000 ) ) ;
#5995=B_SPLINE_CURVE_WITH_KNOTS ( 'NONE', 3,
 ( #7903, #20716, #33110, #20308, #14204, #32706 ),
 .UNSPECIFIED., .F., .F.,
 ( 4, 2, 4 ),
 ( 0.000000000000000000, 0.5000000000000000000, 1.000000000000000000 ),
 .UNSPECIFIED. ) ;
#5997=AXIS2_PLACEMENT_3D ( 'NONE', #38569, #8450, #20848 ) ;
#5998=LINE ( 'NONE', #2371, #35164 ) ;
#6000=ORIENTED_EDGE ( 'NONE', *, *, #36372, .T. ) ;
#6003=VECTOR ( 'NONE', #28500, 1000.000000000000000 ) ;
#6004=ORIENTED_EDGE ( 'NONE', *, *, #13959, .F. ) ;
#6011=DIRECTION ( 'NONE',  ( 0.9135454576426004225, -0.4067366430758009854, 0.000000000000000000 ) ) ;
#6012=EDGE_CURVE ( 'NONE', #13640, #31127, #17073, .T. ) ;
#6014=AXIS2_PLACEMENT_3D ( 'NONE', #23190, #17715, #30090 ) ;
#6015=CARTESIAN_POINT ( 'NONE',  ( 5.564982403289711499, 13.56448261984367676, 10.74999999999999822 ) ) ;
#6016=CARTESIAN_POINT ( 'NONE',  ( 6.557822374958318434, 35.99981354310111925, 10.50000000000000000 ) ) ;
#6017=CARTESIAN_POINT ( 'NONE',  ( 14.11133924723984379, 27.61078317377175750, 7.000000000000000000 ) ) ;
#6020=DIRECTION ( 'NONE',  ( -0.000000000000000000, -0.000000000000000000, -1.000000000000000000 ) ) ;
#6021=ORIENTED_EDGE ( 'NONE', *, *, #37534, .T. ) ;
#6023=DIRECTION ( 'NONE',  ( 0.000000000000000000, -0.000000000000000000, 1.000000000000000000 ) ) ;
#6025=DIRECTION ( 'NONE',  ( 0.000000000000000000, 0.000000000000000000, 1.000000000000000000 ) ) ;
#6031=ORIENTED_EDGE ( 'NONE', *, *, #15748, .F. ) ;
#6037=VECTOR ( 'NONE', #21169, 999.9999999999998863 ) ;
#6041=CARTESIAN_POINT ( 'NONE',  ( 11.60262927932680554, 31.67393310092480618, 10.49999999999999467 ) ) ;
#6043=ORIENTED_EDGE ( 'NONE', *, *, #2575, .T. ) ;
#6045=VECTOR ( 'NONE', #36098, 1000.000000000000000 ) ;
#6047=ORIENTED_EDGE ( 'NONE', *, *, #11888, .T. ) ;
#6048=DIRECTION ( 'NONE',  ( 0.000000000000000000, 0.000000000000000000, 1.000000000000000000 ) ) ;
#6051=DIRECTION ( 'NONE',  ( 0.000000000000000000, 0.000000000000000000, 1.000000000000000000 ) ) ;
#6052=EDGE_CURVE ( 'NONE', #39554, #28465, #37737, .T. ) ;
#6055=VERTEX_POINT ( 'NONE', #32715 ) ;
#6056=CARTESIAN_POINT ( 'NONE',  ( -5.440908595777636414, 35.94977745735568675, 9.000000000000001776 ) ) ;
#6058=DIRECTION ( 'NONE',  ( 0.000000000000000000, 0.000000000000000000, -1.000000000000000000 ) ) ;
#6060=AXIS2_PLACEMENT_3D ( 'NONE', #34650, #19608, #6800 ) ;
#6062=ORIENTED_EDGE ( 'NONE', *, *, #24737, .F. ) ;
#6065=CARTESIAN_POINT ( 'NONE',  ( -12.30736835487442882, 14.81698729810789672, 7.000000000000000000 ) ) ;
#6067=EDGE_CURVE ( 'NONE', #400, #28502, #13608, .T. ) ;
#6071=ORIENTED_EDGE ( 'NONE', *, *, #9109, .F. ) ;
#6076=DIRECTION ( 'NONE',  ( -0.000000000000000000, -0.000000000000000000, 1.000000000000000000 ) ) ;
#6079=CIRCLE ( 'NONE', #15799, 6.000000000000005329 ) ;
#6082=CARTESIAN_POINT ( 'NONE',  ( 11.17899463792469561, 31.89279561836804433, 10.99387789255783332 ) ) ;
#6083=B_SPLINE_CURVE_WITH_KNOTS ( 'NONE', 3,
 ( #10890, #14528, #23672, #26922 ),
 .UNSPECIFIED., .F., .F.,
 ( 4, 4 ),
 ( 0.000000000000000000, 1.000000000000000000 ),
 .UNSPECIFIED. ) ;
#6086=CARTESIAN_POINT ( 'NONE',  ( 0.5000000000000000000, 37.50000000000000711, 10.59344459855570086 ) ) ;
#6088=VECTOR ( 'NONE', #31346, 1000.000000000000114 ) ;
#6089=CARTESIAN_POINT ( 'NONE',  ( -9.428145666828269711, 11.00786382055651202, 10.49999999999999822 ) ) ;
#6090=EDGE_LOOP ( 'NONE', ( #14692, #24896, #25411, #13591 ) ) ;
#6092=DIRECTION ( 'NONE',  ( 0.000000000000000000, 0.000000000000000000, 1.000000000000000000 ) ) ;
#6093=FACE_OUTER_BOUND ( 'NONE', #6287, .T. ) ;
#6095=B_SPLINE_SURFACE_WITH_KNOTS ( 'NONE', 1, 3, ( 
 ( #32576, #23012, #19977, #26870, #32375, #20385, #23224, #17141, #17543, #35414 ),
 ( #7777, #14277, #39259, #27072, #14070, #2097, #20786, #11438, #32985, #36023 ) ),
 .UNSPECIFIED., .F., .F., .F.,
 ( 2, 2 ),
 ( 4, 2, 2, 2, 4 ),
 ( 0.000000000000000000, 1.000000000000000000 ),
 ( 4.486555270693061814, 4.879254352391789951, 5.271953434090517199, 5.664652515789244447, 6.057351597487972583 ),
 .UNSPECIFIED. ) ;
#6096=ORIENTED_EDGE ( 'NONE', *, *, #22508, .T. ) ;
#6099=ORIENTED_EDGE ( 'NONE', *, *, #33633, .T. ) ;
#6107=CARTESIAN_POINT ( 'NONE',  ( 11.19134295108988830, 14.88397459621551100, 9.500000000000000000 ) ) ;
#6110=FACE_OUTER_BOUND ( 'NONE', #20420, .T. ) ;
#6111=CARTESIAN_POINT ( 'NONE',  ( 12.56321727241651764, 14.36790371874248606, 10.49999999999999822 ) ) ;
#6112=ADVANCED_FACE ( 'NONE', ( #20318 ), #4867, .T. ) ;
#6116=DIRECTION ( 'NONE',  ( 0.000000000000000000, 0.000000000000000000, -1.000000000000000000 ) ) ;
#6119=FACE_OUTER_BOUND ( 'NONE', #15682, .T. ) ;
#6120=CARTESIAN_POINT ( 'NONE',  ( 1.400691654708310141, 37.43445890845833901, 7.000000000000000000 ) ) ;
#6122=ORIENTED_EDGE ( 'NONE', *, *, #21193, .F. ) ;
#6127=DIRECTION ( 'NONE',  ( -0.7071067811865531239, 0.000000000000000000, -0.7071067811865417996 ) ) ;
#6128=ORIENTED_EDGE ( 'NONE', *, *, #15043, .T. ) ;
#6129=ORIENTED_EDGE ( 'NONE', *, *, #38612, .T. ) ;
#6134=ORIENTED_EDGE ( 'NONE', *, *, #22755, .F. ) ;
#6139=ORIENTED_EDGE ( 'NONE', *, *, #26697, .F. ) ;
#6141=CARTESIAN_POINT ( 'NONE',  ( 6.980762143445869761, 14.59310681135549537, 10.50000000000000000 ) ) ;
#6142=DIRECTION ( 'NONE',  ( -0.000000000000000000, -0.000000000000000000, -1.000000000000000000 ) ) ;
#6147=ORIENTED_EDGE ( 'NONE', *, *, #3550, .T. ) ;
#6148=ADVANCED_FACE ( 'NONE', ( #28849 ), #1025, .T. ) ;
#6152=ORIENTED_EDGE ( 'NONE', *, *, #25524, .F. ) ;
#6157=DIRECTION ( 'NONE',  ( -0.3535533905932657373, 0.6123724356957934711, 0.7071067811865525687 ) ) ;
#6158=LINE ( 'NONE', #39882, #20167 ) ;
#6160=EDGE_CURVE ( 'NONE', #33983, #30328, #10567, .T. ) ;
#6162=AXIS2_PLACEMENT_3D ( 'NONE', #15361, #23708, #21261 ) ;
#6164=EDGE_CURVE ( 'NONE', #1059, #10078, #16669, .T. ) ;
#6169=LINE ( 'NONE', #9626, #29196 ) ;
#6171=PLANE ( 'NONE',  #27412 ) ;
#6178=ORIENTED_EDGE ( 'NONE', *, *, #18412, .F. ) ;
#6179=CARTESIAN_POINT ( 'NONE',  ( 11.44473057578109199, 31.45924896672603310, 7.499999999999997335 ) ) ;
#6182=CARTESIAN_POINT ( 'NONE',  ( 6.686869517299636634, 14.99761530854296865, 10.49999999999999822 ) ) ;
#6185=AXIS2_PLACEMENT_3D ( 'NONE', #14640, #8134, #26222 ) ;
#6186=ORIENTED_EDGE ( 'NONE', *, *, #14285, .F. ) ;
#6189=CARTESIAN_POINT ( 'NONE',  ( -11.94467491591058916, 31.57458037628605041, 7.130601027986743112 ) ) ;
#6194=CARTESIAN_POINT ( 'NONE',  ( 6.724523273151019609, 35.90846648263063656, 7.485699520496983617 ) ) ;
#6198=EDGE_CURVE ( 'NONE', #855, #4170, #8324, .T. ) ;
#6201=CIRCLE ( 'NONE', #9458, 0.5000000000000004441 ) ;
#6206=DIRECTION ( 'NONE',  ( 0.9781476007338042455, -0.2079116908177664480, 0.000000000000000000 ) ) ;
#6210=CYLINDRICAL_SURFACE ( 'NONE', #22090, 0.4999999999999989453 ) ;
#6213=EDGE_CURVE ( 'NONE', #16505, #20763, #18074, .T. ) ;
#6214=CARTESIAN_POINT ( 'NONE',  ( -6.658969205967785854, 35.40746193325465185, 10.66666666666666607 ) ) ;
#6215=CARTESIAN_POINT ( 'NONE',  ( 5.187504188494417079, 36.60991850771481637, 11.00000000000000000 ) ) ;
#6216=LINE ( 'NONE', #6999, #1947 ) ;
#6217=DIRECTION ( 'NONE',  ( -0.4067366430758009299, -0.9135454576426005335, 0.000000000000000000 ) ) ;
#6218=FACE_OUTER_BOUND ( 'NONE', #29570, .T. ) ;
#6221=DIRECTION ( 'NONE',  ( 1.000000000000000000, 6.938893903907197612E-15, 0.000000000000000000 ) ) ;
#6222=VECTOR ( 'NONE', #25550, 1000.000000000000000 ) ;
#6223=ORIENTED_EDGE ( 'NONE', *, *, #12112, .T. ) ;
#6225=PLANE ( 'NONE',  #22630 ) ;
#6227=CARTESIAN_POINT ( 'NONE',  ( -14.96930490892015797, 21.54088032874991399, 7.000000000000000000 ) ) ;
#6233=VERTEX_POINT ( 'NONE', #5269 ) ;
#6241=FACE_OUTER_BOUND ( 'NONE', #29455, .T. ) ;
#6243=VERTEX_POINT ( 'NONE', #30465 ) ;
#6246=VERTEX_POINT ( 'NONE', #39595 ) ;
#6248=EDGE_CURVE ( 'NONE', #9203, #34232, #39391, .T. ) ;
#6250=AXIS2_PLACEMENT_3D ( 'NONE', #15232, #27226, #15031 ) ;
#6255=EDGE_LOOP ( 'NONE', ( #9151, #11650, #28622, #3994 ) ) ;
#6260=DIRECTION ( 'NONE',  ( 0.000000000000000000, 0.000000000000000000, 1.000000000000000000 ) ) ;
#6261=DIRECTION ( 'NONE',  ( 0.000000000000000000, 0.000000000000000000, -1.000000000000000000 ) ) ;
#6262=EDGE_LOOP ( 'NONE', ( #37176, #10694, #29267, #10179 ) ) ;
#6264=CARTESIAN_POINT ( 'NONE',  ( 4.984135866956514782, 36.15314577889351000, 7.000000000000000000 ) ) ;
#6266=LINE ( 'NONE', #24957, #26673 ) ;
#6273=ADVANCED_FACE ( 'NONE', ( #33722 ), #33521, .T. ) ;
#6277=DIRECTION ( 'NONE',  ( 0.9135454576426050854, 0.4067366430757904938, 0.000000000000000000 ) ) ;
#6281=CARTESIAN_POINT ( 'NONE',  ( -12.49038105676665644, 14.13397459621567798, 7.000000000000000000 ) ) ;
#6284=CARTESIAN_POINT ( 'NONE',  ( 1.000000000000000222, 37.13089969389957901, 10.49999999999999822 ) ) ;
#6285=LINE ( 'NONE', #3249, #4897 ) ;
#6286=CARTESIAN_POINT ( 'NONE',  ( -8.954580980757368636, 11.02572744104269375, 10.99999999999999289 ) ) ;
#6287=EDGE_LOOP ( 'NONE', ( #29533, #16880, #23140 ) ) ;
#6290=DIRECTION ( 'NONE',  ( 1.000000000000000000, 0.000000000000000000, 0.000000000000000000 ) ) ;
#6296=ORIENTED_EDGE ( 'NONE', *, *, #12097, .F. ) ;
#6298=ADVANCED_FACE ( 'NONE', ( #11968 ), #26805, .F. ) ;
#6299=CARTESIAN_POINT ( 'NONE',  ( 4.678013043399745996, 44.50832101651059958, 7.000000000000000000 ) ) ;
#6303=CONICAL_SURFACE ( 'NONE', #21252, 1.000000000000003553, 0.7853981633974514986 ) ;
#6304=CARTESIAN_POINT ( 'NONE',  ( -13.63581098909220479, 27.45627467658446008, 11.00000000000000000 ) ) ;
#6307=CARTESIAN_POINT ( 'NONE',  ( -10.10646936306323518, 32.94553861768095970, 10.49999999999999822 ) ) ;
#6309=AXIS2_PLACEMENT_3D ( 'NONE', #34637, #7396, #6789 ) ;
#6310=DIRECTION ( 'NONE',  ( -0.5254827454987477386, 0.4731467892558253729, -0.7071067811865489050 ) ) ;
#6311=AXIS2_PLACEMENT_3D ( 'NONE', #6799, #35051, #37891 ) ;
#6313=EDGE_CURVE ( 'NONE', #8554, #32472, #760, .T. ) ;
#6316=CARTESIAN_POINT ( 'NONE',  ( -11.11016527260153808, 31.83082137946488643, 9.000000000000001776 ) ) ;
#6317=EDGE_LOOP ( 'NONE', ( #9893, #1133, #28953 ) ) ;
#6322=ORIENTED_EDGE ( 'NONE', *, *, #20212, .T. ) ;
#6323=VERTEX_POINT ( 'NONE', #27010 ) ;
#6327=CIRCLE ( 'NONE', #25794, 0.5000000000000006661 ) ;
#6328=AXIS2_PLACEMENT_3D ( 'NONE', #23887, #29787, #39121 ) ;
#6329=VERTEX_POINT ( 'NONE', #11573 ) ;
#6332=DIRECTION ( 'NONE',  ( -0.2079116908177518763, 0.9781476007338072431, -0.000000000000000000 ) ) ;
#6335=DIRECTION ( 'NONE',  ( -1.000000000000000000, 0.000000000000000000, 0.000000000000000000 ) ) ;
#6336=DIRECTION ( 'NONE',  ( -0.000000000000000000, -0.000000000000000000, -1.000000000000000000 ) ) ;
#6339=B_SPLINE_CURVE_WITH_KNOTS ( 'NONE', 3,
 ( #34038, #37079, #25083, #700 ),
 .UNSPECIFIED., .F., .F.,
 ( 4, 4 ),
 ( 0.000000000000000000, 0.3333333336416847703 ),
 .UNSPECIFIED. ) ;
#6340=ADVANCED_FACE ( 'NONE', ( #5468 ), #2626, .T. ) ;
#6341=ORIENTED_EDGE ( 'NONE', *, *, #14642, .F. ) ;
#6343=AXIS2_PLACEMENT_3D ( 'NONE', #33055, #14347, #11506 ) ;
#6346=ORIENTED_EDGE ( 'NONE', *, *, #37332, .F. ) ;
#6349=DIRECTION ( 'NONE',  ( 0.8660254037844425934, 0.4999999999999933942, 0.000000000000000000 ) ) ;
#6350=FACE_OUTER_BOUND ( 'NONE', #26028, .T. ) ;
#6352=B_SPLINE_CURVE_WITH_KNOTS ( 'NONE', 3,
 ( #9726, #19254, #22699, #3819, #22107, #37353 ),
 .UNSPECIFIED., .F., .F.,
 ( 4, 2, 4 ),
 ( 0.000000000000000000, 0.5000000000000000000, 1.000000000000000000 ),
 .UNSPECIFIED. ) ;
#6354=CIRCLE ( 'NONE', #11569, 0.4999999999999995559 ) ;
#6356=FACE_OUTER_BOUND ( 'NONE', #12359, .T. ) ;
#6359=CARTESIAN_POINT ( 'NONE',  ( 13.37378135583786332, 20.59160479820248923, 10.50000000000000000 ) ) ;
#6362=FACE_OUTER_BOUND ( 'NONE', #34950, .T. ) ;
#6363=ADVANCED_FACE ( 'NONE', ( #15217 ), #23758, .T. ) ;
#6365=AXIS2_PLACEMENT_3D ( 'NONE', #23136, #35535, #4849 ) ;
#6371=ORIENTED_EDGE ( 'NONE', *, *, #7043, .T. ) ;
#6372=FACE_OUTER_BOUND ( 'NONE', #15095, .T. ) ;
#6375=PLANE ( 'NONE',  #9510 ) ;
#6377=CARTESIAN_POINT ( 'NONE',  ( 14.96930490892014731, 21.54088032874976832, 7.000000000000000000 ) ) ;
#6381=DIRECTION ( 'NONE',  ( -0.5254827454987652802, -0.4731467892558137156, -0.7071067811865435759 ) ) ;
#6383=ORIENTED_EDGE ( 'NONE', *, *, #34050, .F. ) ;
#6385=DIRECTION ( 'NONE',  ( -0.3090169943749465631, 0.9510565162951538642, 0.000000000000000000 ) ) ;
#6386=CARTESIAN_POINT ( 'NONE',  ( 11.30736835487432224, 14.81698729810772619, 7.000000000000000000 ) ) ;
#6390=ADVANCED_FACE ( 'NONE', ( #33320 ), #27605, .T. ) ;
#6397=AXIS2_PLACEMENT_3D ( 'NONE', #6056, #36945, #21497 ) ;
#6400=EDGE_CURVE ( 'NONE', #9314, #12011, #14818, .T. ) ;
#6401=VERTEX_POINT ( 'NONE', #22297 ) ;
#6403=DIRECTION ( 'NONE',  ( 0.000000000000000000, 0.000000000000000000, -1.000000000000000000 ) ) ;
#6404=CARTESIAN_POINT ( 'NONE',  ( 9.734896950324680276, 32.61097331450140047, 9.500000000000000000 ) ) ;
#6406=FACE_OUTER_BOUND ( 'NONE', #7619, .T. ) ;
#6407=CARTESIAN_POINT ( 'NONE',  ( 8.910254037844365982, 17.93301270189218855, 10.50000000000000000 ) ) ;
#6408=CARTESIAN_POINT ( 'NONE',  ( -13.63581098909220479, 27.45627467658446008, 9.000000000000001776 ) ) ;
#6409=EDGE_CURVE ( 'NONE', #39958, #30975, #19060, .T. ) ;
#6410=CYLINDRICAL_SURFACE ( 'NONE', #30311, 0.5000000000000011102 ) ;
#6411=CARTESIAN_POINT ( 'NONE',  ( 12.80736835487433289, 15.68301270189216545, 7.000000000000000000 ) ) ;
#6413=EDGE_CURVE ( 'NONE', #11960, #8101, #16215, .T. ) ;
#6416=CARTESIAN_POINT ( 'NONE',  ( 13.28401428800400197, 15.85743772853274969, 10.49999999999999467 ) ) ;
#6417=AXIS2_PLACEMENT_3D ( 'NONE', #31407, #12716, #33872 ) ;
#6421=PLANE ( 'NONE',  #27633 ) ;
#6426=AXIS2_PLACEMENT_3D ( 'NONE', #10817, #22591, #35190 ) ;
#6428=VERTEX_POINT ( 'NONE', #6851 ) ;
#6429=DIRECTION ( 'NONE',  ( 0.5877852522924796874, 0.8090169943749426773, -0.000000000000000000 ) ) ;
#6437=ORIENTED_EDGE ( 'NONE', *, *, #3414, .T. ) ;
#6439=EDGE_CURVE ( 'NONE', #6492, #25420, #28198, .T. ) ;
#6442=ADVANCED_FACE ( 'NONE', ( #15413 ), #18469, .T. ) ;
#6443=PLANE ( 'NONE',  #30410 ) ;
#6444=DIRECTION ( 'NONE',  ( -0.6345370204114130219, -0.5138379476002922219, 0.5773502691896190697 ) ) ;
#6448=AXIS2_PLACEMENT_3D ( 'NONE', #4161, #13706, #32414 ) ;
#6449=ORIENTED_EDGE ( 'NONE', *, *, #8283, .F. ) ;
#6452=VECTOR ( 'NONE', #7909, 1000.000000000000000 ) ;
#6454=DIRECTION ( 'NONE',  ( 0.000000000000000000, 0.000000000000000000, -1.000000000000000000 ) ) ;
#6455=CARTESIAN_POINT ( 'NONE',  ( -9.331903152615899089, 11.35703883385581037, 10.50000000000000533 ) ) ;
#6458=DIRECTION ( 'NONE',  ( 1.000000000000000000, 0.000000000000000000, -0.000000000000000000 ) ) ;
#6459=DIRECTION ( 'NONE',  ( -0.000000000000000000, -0.000000000000000000, -1.000000000000000000 ) ) ;
#6461=DIRECTION ( 'NONE',  ( -1.000000000000000000, 0.000000000000000000, 0.000000000000000000 ) ) ;
#6462=CARTESIAN_POINT ( 'NONE',  ( 2.525645716490524606, 8.212903943950921715, 11.00000000000000000 ) ) ;
#6464=ORIENTED_EDGE ( 'NONE', *, *, #12704, .T. ) ;
#6468=LINE ( 'NONE', #31461, #14608 ) ;
#6469=EDGE_CURVE ( 'NONE', #28502, #34986, #3224, .T. ) ;
#6473=AXIS2_PLACEMENT_3D ( 'NONE', #1032, #2926, #34405 ) ;
#6478=CARTESIAN_POINT ( 'NONE',  ( 7.773262162581151991, 10.11013643092540448, 10.49999999999999822 ) ) ;
#6479=DIRECTION ( 'NONE',  ( -0.9945218953682745111, -0.1045284632676436454, 0.000000000000000000 ) ) ;
#6480=ORIENTED_EDGE ( 'NONE', *, *, #17021, .F. ) ;
#6484=DIRECTION ( 'NONE',  ( -1.000000000000000000, 0.000000000000000000, 0.000000000000000000 ) ) ;
#6487=CARTESIAN_POINT ( 'NONE',  ( 14.51912675677730391, 26.26827554364630402, 7.381627713044570882 ) ) ;
#6488=LINE ( 'NONE', #33549, #14790 ) ;
#6489=ORIENTED_EDGE ( 'NONE', *, *, #39999, .F. ) ;
#6491=DIRECTION ( 'NONE',  ( 0.8090169943749497827, 0.5877852522924698064, 0.000000000000000000 ) ) ;
#6492=VERTEX_POINT ( 'NONE', #34504 ) ;
#6494=ORIENTED_EDGE ( 'NONE', *, *, #30912, .F. ) ;
#6497=DIRECTION ( 'NONE',  ( -0.000000000000000000, -0.000000000000000000, -1.000000000000000000 ) ) ;
#6498=PLANE ( 'NONE',  #29302 ) ;
#6500=PLANE ( 'NONE',  #38891 ) ;
#6501=ORIENTED_EDGE ( 'NONE', *, *, #905, .F. ) ;
#6502=CARTESIAN_POINT ( 'NONE',  ( 4.006135375494214834, 8.432903524120153094, 10.49999999999999822 ) ) ;
#6505=VECTOR ( 'NONE', #6793, 999.9999999999998863 ) ;
#6509=EDGE_CURVE ( 'NONE', #36470, #18790, #36440, .T. ) ;
#6511=CARTESIAN_POINT ( 'NONE',  ( 0.5000000000000000000, 37.50000000000000711, 10.50000000000000000 ) ) ;
#6518=ADVANCED_FACE ( 'NONE', ( #28598 ), #24769, .T. ) ;
#6520=DIRECTION ( 'NONE',  ( 1.000000000000000000, 0.000000000000000000, 0.000000000000000000 ) ) ;
#6521=EDGE_CURVE ( 'NONE', #257, #11836, #31451, .T. ) ;
#6522=ORIENTED_EDGE ( 'NONE', *, *, #28780, .T. ) ;
#6523=ORIENTED_EDGE ( 'NONE', *, *, #39393, .T. ) ;
#6527=ORIENTED_EDGE ( 'NONE', *, *, #23233, .F. ) ;
#6530=DIRECTION ( 'NONE',  ( -0.9135454576425988682, 0.4067366430758048157, 0.000000000000000000 ) ) ;
#6531=VERTEX_POINT ( 'NONE', #3023 ) ;
#6534=CARTESIAN_POINT ( 'NONE',  ( 3.813962023474615215, 32.29559562678520024, 10.50000000000000000 ) ) ;
#6535=AXIS2_PLACEMENT_3D ( 'NONE', #39291, #11468, #32409 ) ;
#6536=ORIENTED_EDGE ( 'NONE', *, *, #18115, .F. ) ;
#6538=ORIENTED_EDGE ( 'NONE', *, *, #16006, .F. ) ;
#6542=EDGE_CURVE ( 'NONE', #37934, #25787, #2078, .T. ) ;
#6543=VERTEX_POINT ( 'NONE', #574 ) ;
#6545=EDGE_CURVE ( 'NONE', #19499, #18941, #40191, .T. ) ;
#6548=AXIS2_PLACEMENT_3D ( 'NONE', #32357, #16919, #8162 ) ;
#6549=DIRECTION ( 'NONE',  ( -0.1045284632676437842, 0.9945218953682744001, -0.000000000000000000 ) ) ;
#6550=AXIS2_PLACEMENT_3D ( 'NONE', #29298, #13855, #7953 ) ;
#6553=CARTESIAN_POINT ( 'NONE',  ( 13.94482798346721353, 26.50521816028912525, 9.000000000000001776 ) ) ;
#6560=ORIENTED_EDGE ( 'NONE', *, *, #9500, .F. ) ;
#6563=CARTESIAN_POINT ( 'NONE',  ( 10.44367147699342091, 33.07775263288196754, 10.49999999999999822 ) ) ;
#6565=ORIENTED_EDGE ( 'NONE', *, *, #17365, .T. ) ;
#6571=CARTESIAN_POINT ( 'NONE',  ( 10.04974741695038354, 22.44923726269170672, 10.50000000000000533 ) ) ;
#6572=AXIS2_PLACEMENT_3D ( 'NONE', #20726, #36551, #17481 ) ;
#6576=FACE_OUTER_BOUND ( 'NONE', #26094, .T. ) ;
#6580=VECTOR ( 'NONE', #25387, 1000.000000000000000 ) ;
#6581=FACE_OUTER_BOUND ( 'NONE', #14752, .T. ) ;
#6584=B_SPLINE_CURVE_WITH_KNOTS ( 'NONE', 3,
 ( #36806, #24809, #21367, #27457 ),
 .UNSPECIFIED., .F., .F.,
 ( 4, 4 ),
 ( 0.0005941180652377696467, 0.0009459474155737164318 ),
 .UNSPECIFIED. ) ;
#6589=ORIENTED_EDGE ( 'NONE', *, *, #1844, .T. ) ;
#6590=VECTOR ( 'NONE', #20939, 1000.000000000000000 ) ;
#6594=ORIENTED_EDGE ( 'NONE', *, *, #28271, .T. ) ;
#6601=DIRECTION ( 'NONE',  ( 0.4067366430758010964, 0.9135454576426005335, 0.000000000000000000 ) ) ;
#6602=CYLINDRICAL_SURFACE ( 'NONE', #20974, 0.4999999999999995559 ) ;
#6606=CARTESIAN_POINT ( 'NONE',  ( -14.51390269127088928, 5.102206419419879957, 7.000000000000000000 ) ) ;
#6609=CARTESIAN_POINT ( 'NONE',  ( -5.400683141673551013, 15.91724817395922997, 9.000000000000001776 ) ) ;
#6612=AXIS2_PLACEMENT_3D ( 'NONE', #32238, #8659, #20661 ) ;
#6617=ORIENTED_EDGE ( 'NONE', *, *, #29099, .F. ) ;
#6618=DIRECTION ( 'NONE',  ( -1.000000000000000000, 0.000000000000000000, 0.000000000000000000 ) ) ;
#6621=ADVANCED_FACE ( 'NONE', ( #28396 ), #15614, .F. ) ;
#6625=ORIENTED_EDGE ( 'NONE', *, *, #22530, .T. ) ;
#6633=ORIENTED_EDGE ( 'NONE', *, *, #18111, .T. ) ;
#6634=CARTESIAN_POINT ( 'NONE',  ( 2.229970528062776403, 7.666518487011187766, 7.381627713044564665 ) ) ;
#6635=CARTESIAN_POINT ( 'NONE',  ( 2.525645716490518389, 8.212903943950921715, 7.000000000000000000 ) ) ;
#6636=EDGE_CURVE ( 'NONE', #22937, #19894, #9723, .T. ) ;
#6638=EDGE_CURVE ( 'NONE', #18932, #2112, #16333, .T. ) ;
#6640=EDGE_CURVE ( 'NONE', #26114, #19442, #12446, .T. ) ;
#6642=VERTEX_POINT ( 'NONE', #22896 ) ;
#6644=EDGE_LOOP ( 'NONE', ( #10715, #17713, #3208, #32996, #32591 ) ) ;
#6647=AXIS2_PLACEMENT_3D ( 'NONE', #1299, #37863, #12880 ) ;
#6648=LINE ( 'NONE', #31447, #22034 ) ;
#6652=DIRECTION ( 'NONE',  ( 0.4067366430758009299, 0.9135454576426005335, 0.000000000000000000 ) ) ;
#6654=FACE_OUTER_BOUND ( 'NONE', #3146, .T. ) ;
#6656=CARTESIAN_POINT ( 'NONE',  ( 2.579909280894411516, 7.957613945008743528, 10.94611345180490858 ) ) ;
#6658=EDGE_LOOP ( 'NONE', ( #33741, #1092, #6997 ) ) ;
#6661=ADVANCED_FACE ( 'NONE', ( #20267 ), #34899, .T. ) ;
#6663=CARTESIAN_POINT ( 'NONE',  ( 6.354454053420411697, 35.54304081427980577, 7.000000000000000000 ) ) ;
#6666=DIRECTION ( 'NONE',  ( -0.5000000000000038858, -0.8660254037844363761, 0.000000000000000000 ) ) ;
#6667=AXIS2_PLACEMENT_3D ( 'NONE', #39498, #2533, #17786 ) ;
#6672=VECTOR ( 'NONE', #16058, 1000.000000000000114 ) ;
#6673=FACE_OUTER_BOUND ( 'NONE', #12882, .T. ) ;
#6675=ORIENTED_EDGE ( 'NONE', *, *, #6509, .T. ) ;
#6677=CARTESIAN_POINT ( 'NONE',  ( -7.910872327081295730, 10.00199400870863187, 10.49999999999999822 ) ) ;
#6679=CYLINDRICAL_SURFACE ( 'NONE', #35807, 15.00000000000000000 ) ;
#6682=CARTESIAN_POINT ( 'NONE',  ( -14.44975846301057310, 26.39485539169832506, 10.49999999999999467 ) ) ;
#6683=CYLINDRICAL_SURFACE ( 'NONE', #34940, 6.000000000000003553 ) ;
#6690=CIRCLE ( 'NONE', #29413, 1.000000000000000444 ) ;
#6691=VERTEX_POINT ( 'NONE', #16621 ) ;
#6693=DIRECTION ( 'NONE',  ( -0.7431448254773862505, 0.6691306063588672304, -0.000000000000000000 ) ) ;
#6699=DIRECTION ( 'NONE',  ( -0.000000000000000000, -0.000000000000000000, -1.000000000000000000 ) ) ;
#6702=DIRECTION ( 'NONE',  ( 0.000000000000000000, 0.000000000000000000, 1.000000000000000000 ) ) ;
#6703=CARTESIAN_POINT ( 'NONE',  ( -3.000488737322915878, 30.46850471150003159, 9.000000000000001776 ) ) ;
#6706=VECTOR ( 'NONE', #20516, 1000.000000000000000 ) ;
#6708=CARTESIAN_POINT ( 'NONE',  ( 9.997483185316555776, 21.95197631500756685, 10.50000000000000000 ) ) ;
#6709=CARTESIAN_POINT ( 'NONE',  ( -14.52509594610762456, 21.97885917798744870, 10.49999999999999467 ) ) ;
#6710=ORIENTED_EDGE ( 'NONE', *, *, #39152, .T. ) ;
#6712=AXIS2_PLACEMENT_3D ( 'NONE', #36212, #14463, #2084 ) ;
#6716=ORIENTED_EDGE ( 'NONE', *, *, #15796, .T. ) ;
#6721=AXIS2_PLACEMENT_3D ( 'NONE', #14574, #11925, #39353 ) ;
#6724=DIRECTION ( 'NONE',  ( 0.6459741880212575005, 0.2876062384759433543, -0.7071067811865445751 ) ) ;
#6725=EDGE_LOOP ( 'NONE', ( #31565, #9056, #32529, #5697, #3716, #29240, #31276 ) ) ;
#6728=FACE_OUTER_BOUND ( 'NONE', #9714, .T. ) ;
#6729=B_SPLINE_CURVE_WITH_KNOTS ( 'NONE', 3,
 ( #15470, #16068, #15670, #15872, #9377, #31113 ),
 .UNSPECIFIED., .F., .F.,
 ( 4, 2, 4 ),
 ( 0.000000000000000000, 0.5000000000000000000, 1.000000000000000000 ),
 .UNSPECIFIED. ) ;
#6730=B_SPLINE_CURVE_WITH_KNOTS ( 'NONE', 3,
 ( #6307, #27852, #21552, #36999 ),
 .UNSPECIFIED., .F., .F.,
 ( 4, 4 ),
 ( 0.000000000000000000, 1.000000000000000000 ),
 .UNSPECIFIED. ) ;
#6733=VERTEX_POINT ( 'NONE', #4215 ) ;
#6735=AXIS2_PLACEMENT_3D ( 'NONE', #26555, #17220, #38743 ) ;
#6738=EDGE_CURVE ( 'NONE', #31599, #20519, #26717, .T. ) ;
#6740=DIRECTION ( 'NONE',  ( 1.000000000000000000, 0.000000000000000000, 0.000000000000000000 ) ) ;
#6742=VECTOR ( 'NONE', #20071, 1000.000000000000000 ) ;
#6744=ADVANCED_FACE ( 'NONE', ( #10929 ), #5895, .T. ) ;
#6745=FACE_OUTER_BOUND ( 'NONE', #12798, .T. ) ;
#6747=B_SPLINE_SURFACE_WITH_KNOTS ( 'NONE', 1, 3, ( 
 ( #36340, #5456, #27191, #23138, #11153, #35740, #38780, #4652, #10958, #32698 ),
 ( #23345, #20099, #8504, #29835, #33102, #8308, #11557, #29635, #20901, #14194 ) ),
 .UNSPECIFIED., .F., .F., .F.,
 ( 2, 2 ),
 ( 4, 2, 2, 2, 4 ),
 ( 0.000000000000000000, 1.000000000000000000 ),
 ( -1.096214744126243978, -0.7035156624275198389, -0.3108165807287956994, 0.08188250096992841232, 0.4745815826686525241 ),
 .UNSPECIFIED. ) ;
#6756=AXIS2_PLACEMENT_3D ( 'NONE', #30904, #24402, #30706 ) ;
#6759=ADVANCED_FACE ( 'NONE', ( #28999 ), #26562, .F. ) ;
#6761=CARTESIAN_POINT ( 'NONE',  ( -3.357189294653179612, 32.49896394832315849, 10.50000000000000000 ) ) ;
#6767=CARTESIAN_POINT ( 'NONE',  ( -14.60301432615393047, 21.46791548645777326, 11.00000000000000000 ) ) ;
#6769=CARTESIAN_POINT ( 'NONE',  ( 0.000000000000000000, 22.50000000000000355, 7.000000000000000000 ) ) ;
#6773=DIRECTION ( 'NONE',  ( -0.000000000000000000, -0.000000000000000000, -1.000000000000000000 ) ) ;
#6775=ORIENTED_EDGE ( 'NONE', *, *, #24897, .F. ) ;
#6777=DIRECTION ( 'NONE',  ( 0.000000000000000000, 0.000000000000000000, 1.000000000000000000 ) ) ;
#6779=CARTESIAN_POINT ( 'NONE',  ( -13.16028273094462975, 27.30176617939698147, 7.499999999999994671 ) ) ;
#6780=ORIENTED_EDGE ( 'NONE', *, *, #3316, .T. ) ;
#6782=AXIS2_PLACEMENT_3D ( 'NONE', #34962, #631, #16474 ) ;
#6787=EDGE_CURVE ( 'NONE', #36443, #31380, #10327, .T. ) ;
#6789=DIRECTION ( 'NONE',  ( 0.3090169943749448977, -0.9510565162951543083, 0.000000000000000000 ) ) ;
#6791=ORIENTED_EDGE ( 'NONE', *, *, #4610, .T. ) ;
#6792=LINE ( 'NONE', #518, #10640 ) ;
#6793=DIRECTION ( 'NONE',  ( -0.7431448254773863615, 0.6691306063588671194, 0.000000000000000000 ) ) ;
#6796=CARTESIAN_POINT ( 'NONE',  ( -6.811226782241547539, 35.33967249274200384, 10.50000000000000355 ) ) ;
#6797=DIRECTION ( 'NONE',  ( 0.6123724356957939152, -0.3535533905932699561, -0.7071067811865499042 ) ) ;
#6798=DIRECTION ( 'NONE',  ( -0.5000000000000038858, -0.8660254037844363761, 0.000000000000000000 ) ) ;
#6799=CARTESIAN_POINT ( 'NONE',  ( -7.014595103779441843, 35.79644522156330311, 11.00000000000000000 ) ) ;
#6800=DIRECTION ( 'NONE',  ( -0.1045284632676415082, 0.9945218953682745111, 0.000000000000000000 ) ) ;
#6802=VECTOR ( 'NONE', #10528, 1000.000000000000000 ) ;
#6804=CARTESIAN_POINT ( 'NONE',  ( 0.000000000000000000, 22.50000000000000355, 7.000000000000000000 ) ) ;
#6805=VERTEX_POINT ( 'NONE', #4623 ) ;
#6807=DIRECTION ( 'NONE',  ( -0.2876062384759714985, -0.6459741880212498399, -0.7071067811865401342 ) ) ;
#6809=ADVANCED_FACE ( 'NONE', ( #29403 ), #10117, .T. ) ;
#6812=CARTESIAN_POINT ( 'NONE',  ( -1.204925152852743597, 12.02153850147729486, 10.50000000000000355 ) ) ;
#6814=ORIENTED_EDGE ( 'NONE', *, *, #6738, .F. ) ;
#6817=CIRCLE ( 'NONE', #29544, 1.000000000000004441 ) ;
#6822=AXIS2_PLACEMENT_3D ( 'NONE', #17949, #2305, #5538 ) ;
#6826=ORIENTED_EDGE ( 'NONE', *, *, #31867, .F. ) ;
#6828=CARTESIAN_POINT ( 'NONE',  ( 11.44473057578109199, 31.45924896672603310, 10.50000000000000178 ) ) ;
#6830=ORIENTED_EDGE ( 'NONE', *, *, #5808, .F. ) ;
#6835=CARTESIAN_POINT ( 'NONE',  ( 10.29511041547405625, 24.79362192464176573, 10.50000000000000000 ) ) ;
#6837=ADVANCED_FACE ( 'NONE', ( #975 ), #13356, .T. ) ;
#6841=ORIENTED_EDGE ( 'NONE', *, *, #18962, .F. ) ;
#6842=DIRECTION ( 'NONE',  ( -0.6691306063588569053, 0.7431448254773954654, 0.000000000000000000 ) ) ;
#6843=VECTOR ( 'NONE', #6127, 1000.000000000000114 ) ;
#6847=CARTESIAN_POINT ( 'NONE',  ( 7.530592408760851342, 11.28437794979193853, 7.000000000000000000 ) ) ;
#6848=ORIENTED_EDGE ( 'NONE', *, *, #31935, .F. ) ;
#6850=PLANE ( 'NONE',  #13291 ) ;
#6851=CARTESIAN_POINT ( 'NONE',  ( -9.427394655428429360, 11.06314620770957013, 7.500000000000000888 ) ) ;
#6852=CARTESIAN_POINT ( 'NONE',  ( -10.73859285986284640, 31.49625607628545154, 7.000000000000000000 ) ) ;
#6853=PLANE ( 'NONE',  #2223 ) ;
#6854=CARTESIAN_POINT ( 'NONE',  ( 13.94482798346721353, 26.50521816028912525, 7.500000000000000888 ) ) ;
#6856=CARTESIAN_POINT ( 'NONE',  ( -11.87435565298220475, 15.06698729810788961, 7.499999999999993783 ) ) ;
#6857=EDGE_LOOP ( 'NONE', ( #26177, #27169, #14502, #32129 ) ) ;
#6859=CARTESIAN_POINT ( 'NONE',  ( -8.843266739736657556, 16.81698729810786830, 10.50000000000000000 ) ) ;
#6862=CARTESIAN_POINT ( 'NONE',  ( 1.500000000000000888, 37.00000000000000711, 7.000000000000000000 ) ) ;
#6866=CARTESIAN_POINT ( 'NONE',  ( 7.713869163865850531, 10.18146832927074996, 9.500000000000000000 ) ) ;
#6867=ADVANCED_FACE ( 'NONE', ( #24109 ), #2383, .T. ) ;
#6872=CARTESIAN_POINT ( 'NONE',  ( -6.811226782241547539, 35.33967249274200384, 10.50000000000000355 ) ) ;
#6874=ORIENTED_EDGE ( 'NONE', *, *, #24797, .T. ) ;
#6876=AXIS2_PLACEMENT_3D ( 'NONE', #35570, #5089, #19931 ) ;
#6877=VECTOR ( 'NONE', #35474, 1000.000000000000114 ) ;
#6878=CARTESIAN_POINT ( 'NONE',  ( 14.81003276707481575, 21.44615697153870570, 10.87262190629277825 ) ) ;
#6879=ORIENTED_EDGE ( 'NONE', *, *, #25880, .F. ) ;
#6881=DIRECTION ( 'NONE',  ( -0.3090169943749574988, -0.9510565162951503115, 0.000000000000000000 ) ) ;
#6883=DIRECTION ( 'NONE',  ( -0.9986295347545744994, -0.05233595624293203852, 0.000000000000000000 ) ) ;
#6886=DIRECTION ( 'NONE',  ( -0.9135454576426059736, -0.4067366430757887730, 0.000000000000000000 ) ) ;
#6890=EDGE_CURVE ( 'NONE', #959, #2993, #25984, .T. ) ;
#6891=ORIENTED_EDGE ( 'NONE', *, *, #18373, .F. ) ;
#6893=CARTESIAN_POINT ( 'NONE',  ( 16.72075857324119141, 7.444561356925491147, 7.000000000000000000 ) ) ;
#6894=CARTESIAN_POINT ( 'NONE',  ( 6.864468484318075880, 35.45925531351068116, 10.49999999999999822 ) ) ;
#6896=EDGE_CURVE ( 'NONE', #40197, #1489, #23414, .T. ) ;
#6897=LINE ( 'NONE', #13402, #13589 ) ;
#6899=CARTESIAN_POINT ( 'NONE',  ( 3.553336972204391042, 8.187731063815824939, 10.94387467463491959 ) ) ;
#6902=DIRECTION ( 'NONE',  ( -0.9135454576426051965, -0.4067366430757904938, 0.000000000000000000 ) ) ;
#6905=VECTOR ( 'NONE', #22817, 1000.000000000000000 ) ;
#6906=VERTEX_POINT ( 'NONE', #5022 ) ;
#6909=ADVANCED_FACE ( 'NONE', ( #20873 ), #18222, .T. ) ;
#6910=CARTESIAN_POINT ( 'NONE',  ( 0.7624269476132105039, 37.48077593123142748, 7.455539900862801161 ) ) ;
#6911=EDGE_CURVE ( 'NONE', #2141, #22956, #30007, .T. ) ;
#6917=ORIENTED_EDGE ( 'NONE', *, *, #26253, .F. ) ;
#6923=DIRECTION ( 'NONE',  ( 0.9781476007338042455, -0.2079116908177663647, 0.000000000000000000 ) ) ;
#6928=VERTEX_POINT ( 'NONE', #30614 ) ;
#6931=EDGE_CURVE ( 'NONE', #9898, #751, #37044, .T. ) ;
#6932=EDGE_LOOP ( 'NONE', ( #8435, #35748, #18153, #18927 ) ) ;
#6934=AXIS2_PLACEMENT_3D ( 'NONE', #14750, #21046, #27139 ) ;
#6937=EDGE_CURVE ( 'NONE', #1084, #24976, #23355, .T. ) ;
#6940=AXIS2_PLACEMENT_3D ( 'NONE', #17424, #2174, #29592 ) ;
#6941=CARTESIAN_POINT ( 'NONE',  ( 5.537946624086020009, 36.44027069998191593, 7.000000000000000000 ) ) ;
#6943=CARTESIAN_POINT ( 'NONE',  ( 10.36702044712426840, 31.16169077310587809, 10.00000000000000000 ) ) ;
#6944=CARTESIAN_POINT ( 'NONE',  ( 11.69134295108989008, 15.74999999999995204, 7.000000000000000000 ) ) ;
#6950=VECTOR ( 'NONE', #38679, 999.9999999999998863 ) ;
#6951=ORIENTED_EDGE ( 'NONE', *, *, #6248, .F. ) ;
#6953=CIRCLE ( 'NONE', #3750, 6.000000000000003553 ) ;
#6955=CARTESIAN_POINT ( 'NONE',  ( 10.61811999842815801, 32.73341455422742285, 10.94387467463499242 ) ) ;
#6957=VERTEX_POINT ( 'NONE', #5616 ) ;
#6959=ADVANCED_FACE ( 'NONE', ( #11327 ), #31188, .T. ) ;
#6960=DIRECTION ( 'NONE',  ( 0.7431448254773862505, -0.6691306063588670083, 0.000000000000000000 ) ) ;
#6961=ORIENTED_EDGE ( 'NONE', *, *, #26501, .F. ) ;
#6964=DIRECTION ( 'NONE',  ( 0.6459741880212486187, -0.2876062384759502932, -0.7071067811865500152 ) ) ;
#6966=CARTESIAN_POINT ( 'NONE',  ( 12.60100158617205857, 14.64745807297493663, 10.87262190629442671 ) ) ;
#6967=AXIS2_PLACEMENT_3D ( 'NONE', #8856, #21047, #8653 ) ;
#6968=ORIENTED_EDGE ( 'NONE', *, *, #290, .F. ) ;
#6973=EDGE_LOOP ( 'NONE', ( #20708, #30992, #5057, #11296 ) ) ;
#6978=ORIENTED_EDGE ( 'NONE', *, *, #29239, .F. ) ;
#6983=CIRCLE ( 'NONE', #29709, 0.5000000000000004441 ) ;
#6985=CARTESIAN_POINT ( 'NONE',  ( 0.5000000000000012212, 31.00000000000000355, 9.000000000000001776 ) ) ;
#6988=VERTEX_POINT ( 'NONE', #18026 ) ;
#6989=EDGE_CURVE ( 'NONE', #9581, #39411, #3948, .T. ) ;
#6990=CARTESIAN_POINT ( 'NONE',  ( -7.951799764322637465, 28.98701630243970229, 10.74999999999999467 ) ) ;
#6991=AXIS2_PLACEMENT_3D ( 'NONE', #17674, #30048, #27393 ) ;
#6992=AXIS2_PLACEMENT_3D ( 'NONE', #7490, #19283, #1006 ) ;
#6993=CARTESIAN_POINT ( 'NONE',  ( -11.44473057578097475, 31.45924896672618587, 10.49999999999999822 ) ) ;
#6996=LINE ( 'NONE', #21651, #17235 ) ;
#6997=ORIENTED_EDGE ( 'NONE', *, *, #37595, .T. ) ;
#6999=CARTESIAN_POINT ( 'NONE',  ( -3.610593701936590350, 31.83882289796395426, 10.50000000000000533 ) ) ;
#7002=DIRECTION ( 'NONE',  ( 0.000000000000000000, 0.000000000000000000, -1.000000000000000000 ) ) ;
#7003=LINE ( 'NONE', #4368, #211 ) ;
#7004=CARTESIAN_POINT ( 'NONE',  ( 10.49474413300069386, 21.89971208337374264, 10.00000000000000000 ) ) ;
#7006=DIRECTION ( 'NONE',  ( -0.5877852522924796874, -0.8090169943749426773, 0.000000000000000000 ) ) ;
#7009=CARTESIAN_POINT ( 'NONE',  ( 2.141014423449929094, 7.887532638883552494, 10.49999999999999822 ) ) ;
#7011=ADVANCED_FACE ( 'NONE', ( #5426 ), #7420, .T. ) ;
#7013=CARTESIAN_POINT ( 'NONE',  ( -11.11016527260153808, 31.83082137946488643, 7.000000000000000000 ) ) ;
#7017=ORIENTED_EDGE ( 'NONE', *, *, #32946, .T. ) ;
#7019=CARTESIAN_POINT ( 'NONE',  ( 14.26801110064894829, 26.12045026487100330, 10.49999999999999822 ) ) ;
#7029=CARTESIAN_POINT ( 'NONE',  ( -11.69134295108998245, 15.75000000000011191, 7.000000000000000000 ) ) ;
#7030=EDGE_CURVE ( 'NONE', #14313, #10247, #33863, .T. ) ;
#7032=AXIS2_PLACEMENT_3D ( 'NONE', #33419, #8819, #17969 ) ;
#7042=ORIENTED_EDGE ( 'NONE', *, *, #28148, .T. ) ;
#7043=EDGE_CURVE ( 'NONE', #11758, #12092, #24904, .T. ) ;
#7044=ORIENTED_EDGE ( 'NONE', *, *, #15955, .T. ) ;
#7045=EDGE_CURVE ( 'NONE', #37653, #6642, #12119, .T. ) ;
#7048=AXIS2_PLACEMENT_3D ( 'NONE', #25360, #34918, #9932 ) ;
#7049=CIRCLE ( 'NONE', #23949, 1.000000000000009548 ) ;
#7050=CYLINDRICAL_SURFACE ( 'NONE', #30485, 0.5000000000000004441 ) ;
#7057=CARTESIAN_POINT ( 'NONE',  ( -1.000000000000000000, 37.00000000000000711, 7.500000000000000888 ) ) ;
#7058=CARTESIAN_POINT ( 'NONE',  ( 6.980762143445869761, 14.59310681135549537, 10.49999999999999645 ) ) ;
#7060=DIRECTION ( 'NONE',  ( 0.6123724356958033521, 0.3535533905932687349, -0.7071067811865423547 ) ) ;
#7061=ORIENTED_EDGE ( 'NONE', *, *, #32229, .F. ) ;
#7063=CARTESIAN_POINT ( 'NONE',  ( -12.30736835487443415, 14.81698729810790560, 11.00000000000000000 ) ) ;
#7064=CARTESIAN_POINT ( 'NONE',  ( 3.503793317224329851, 8.420815634768676006, 7.000000000000000000 ) ) ;
#7066=CARTESIAN_POINT ( 'NONE',  ( -3.399837471815634338, 8.909889435135630364, 9.500000000000000000 ) ) ;
#7069=EDGE_CURVE ( 'NONE', #4297, #9720, #31591, .T. ) ;
#7075=DIRECTION ( 'NONE',  ( 0.8090169943749505599, 0.5877852522924689183, -0.000000000000000000 ) ) ;
#7076=CARTESIAN_POINT ( 'NONE',  ( -8.412270287199726582, 10.07085245822961994, 10.49999999999999822 ) ) ;
#7080=CARTESIAN_POINT ( 'NONE',  ( 14.96161608456799463, 21.61429412723660093, 10.49999999999999822 ) ) ;
#7083=DIRECTION ( 'NONE',  ( -0.000000000000000000, 0.000000000000000000, -1.000000000000000000 ) ) ;
#7084=CARTESIAN_POINT ( 'NONE',  ( -0.5000000000000005551, 31.00000000000000355, 7.000000000000000000 ) ) ;
#7085=B_SPLINE_CURVE_WITH_KNOTS ( 'NONE', 3,
 ( #25751, #22304, #16417, #9923, #40039, #36803 ),
 .UNSPECIFIED., .F., .F.,
 ( 4, 2, 4 ),
 ( 0.000000000000000000, 0.5000000000000008882, 1.000000000000000000 ),
 .UNSPECIFIED. ) ;
#7090=DIRECTION ( 'NONE',  ( -0.2588190451025098593, 0.9659258262890711988, -1.387778780781446292E-17 ) ) ;
#7091=ORIENTED_EDGE ( 'NONE', *, *, #29703, .T. ) ;
#7096=EDGE_CURVE ( 'NONE', #22335, #28046, #36903, .T. ) ;
#7097=CARTESIAN_POINT ( 'NONE',  ( -12.82065967939308848, 40.99677499958261961, 11.00000000000000000 ) ) ;
#7098=CARTESIAN_POINT ( 'NONE',  ( -3.860444543167080855, 8.005107441538555690, 7.455539900862796721 ) ) ;
#7099=B_SPLINE_CURVE_WITH_KNOTS ( 'NONE', 3,
 ( #29076, #10190, #4087, #16692, #12835, #7329 ),
 .UNSPECIFIED., .F., .F.,
 ( 4, 2, 4 ),
 ( 0.0001748523089235895619, 0.0005603998622486582688, 0.0009459474155737269485 ),
 .UNSPECIFIED. ) ;
#7100=ADVANCED_FACE ( 'NONE', ( #18815 ), #12315, .T. ) ;
#7102=DIRECTION ( 'NONE',  ( -1.000000000000000000, 0.000000000000000000, 0.000000000000000000 ) ) ;
#7103=EDGE_LOOP ( 'NONE', ( #15945, #38581, #792, #1542 ) ) ;
#7106=CARTESIAN_POINT ( 'NONE',  ( 3.503793317224327186, 8.420815634768674229, 11.00000000000000000 ) ) ;
#7111=DIRECTION ( 'NONE',  ( -0.000000000000000000, -0.000000000000000000, -1.000000000000000000 ) ) ;
#7114=CIRCLE ( 'NONE', #20100, 15.00000000000000000 ) ;
#7115=CARTESIAN_POINT ( 'NONE',  ( -12.30736835487442882, 14.81698729810789672, 11.00000000000000000 ) ) ;
#7116=ADVANCED_FACE ( 'NONE', ( #31398 ), #3565, .T. ) ;
#7121=EDGE_CURVE ( 'NONE', #30787, #36810, #34452, .T. ) ;
#7122=CARTESIAN_POINT ( 'NONE',  ( -12.19134295108997890, 16.61602540378455117, 10.50000000000000000 ) ) ;
#7126=DIRECTION ( 'NONE',  ( 0.9135454576426005335, -0.4067366430758010964, 0.000000000000000000 ) ) ;
#7128=EDGE_CURVE ( 'NONE', #8399, #23608, #32504, .T. ) ;
#7130=DIRECTION ( 'NONE',  ( -0.9781476007338041345, 0.2079116908177663370, 0.000000000000000000 ) ) ;
#7135=ORIENTED_EDGE ( 'NONE', *, *, #27023, .T. ) ;
#7137=CARTESIAN_POINT ( 'NONE',  ( -5.644276917315534270, 36.40655018617698602, 10.49999999999999822 ) ) ;
#7144=EDGE_CURVE ( 'NONE', #12750, #22676, #37297, .T. ) ;
#7145=VECTOR ( 'NONE', #9265, 1000.000000000000000 ) ;
#7148=ADVANCED_FACE ( 'NONE', ( #37500 ), #20016, .T. ) ;
#7150=CARTESIAN_POINT ( 'NONE',  ( -13.32679399471724935, 28.40733119287961728, 7.000000000000000000 ) ) ;
#7151=DIRECTION ( 'NONE',  ( 1.000000000000000000, 0.000000000000000000, 0.000000000000000000 ) ) ;
#7152=AXIS2_PLACEMENT_3D ( 'NONE', #22889, #35294, #13752 ) ;
#7155=AXIS2_PLACEMENT_3D ( 'NONE', #2772, #20675, #2183 ) ;
#7159=ORIENTED_EDGE ( 'NONE', *, *, #39641, .T. ) ;
#7160=EDGE_CURVE ( 'NONE', #9720, #37009, #29350, .T. ) ;
#7162=VERTEX_POINT ( 'NONE', #16771 ) ;
#7166=CARTESIAN_POINT ( 'NONE',  ( 13.94482798346721353, 26.50521816028912525, 7.000000000000000000 ) ) ;
#7168=VERTEX_POINT ( 'NONE', #4570 ) ;
#7170=CARTESIAN_POINT ( 'NONE',  ( -12.49038105676665644, 14.13397459621567798, 11.00000000000000000 ) ) ;
#7172=ORIENTED_EDGE ( 'NONE', *, *, #21690, .T. ) ;
#7174=CARTESIAN_POINT ( 'NONE',  ( 8.070499922308650653, 9.855951069525808350, 7.381627713044574435 ) ) ;
#7184=FACE_OUTER_BOUND ( 'NONE', #35137, .T. ) ;
#7185=CARTESIAN_POINT ( 'NONE',  ( 6.404490139165910811, 34.42612703509929872, 10.50000000000000000 ) ) ;
#7191=AXIS2_PLACEMENT_3D ( 'NONE', #23201, #29696, #7755 ) ;
#7192=ORIENTED_EDGE ( 'NONE', *, *, #31263, .T. ) ;
#7194=CARTESIAN_POINT ( 'NONE',  ( 13.13581098909226874, 27.45627467658428955, 9.500000000000000000 ) ) ;
#7196=AXIS2_PLACEMENT_3D ( 'NONE', #16825, #16622, #31849 ) ;
#7198=DIRECTION ( 'NONE',  ( 0.000000000000000000, 0.000000000000000000, 1.000000000000000000 ) ) ;
#7200=CARTESIAN_POINT ( 'NONE',  ( 13.24038105676655341, 15.43301270189216368, 10.63089969389957368 ) ) ;
#7203=FACE_OUTER_BOUND ( 'NONE', #19291, .T. ) ;
#7205=DIRECTION ( 'NONE',  ( 0.000000000000000000, 0.000000000000000000, -1.000000000000000000 ) ) ;
#7206=PLANE ( 'NONE',  #6060 ) ;
#7208=LINE ( 'NONE', #10885, #32771 ) ;
#7209=ORIENTED_EDGE ( 'NONE', *, *, #24311, .T. ) ;
#7210=VECTOR ( 'NONE', #14415, 1000.000000000000114 ) ;
#7215=LINE ( 'NONE', #16578, #37316 ) ;
#7219=ORIENTED_EDGE ( 'NONE', *, *, #1413, .T. ) ;
#7230=CIRCLE ( 'NONE', #22799, 0.9999999999999997780 ) ;
#7233=ORIENTED_EDGE ( 'NONE', *, *, #13082, .T. ) ;
#7241=AXIS2_PLACEMENT_3D ( 'NONE', #6065, #34305, #21505 ) ;
#7242=ADVANCED_FACE ( 'NONE', ( #31795 ), #19491, .T. ) ;
#7246=LINE ( 'NONE', #19646, #667 ) ;
#7247=CARTESIAN_POINT ( 'NONE',  ( 5.494150297854179854, 36.06936027812436407, 10.99999999999999822 ) ) ;
#7248=VERTEX_POINT ( 'NONE', #16361 ) ;
#7251=CARTESIAN_POINT ( 'NONE',  ( 12.80736835487433289, 15.68301270189216545, 7.000000000000000000 ) ) ;
#7252=DIRECTION ( 'NONE',  ( -0.6691306063588670083, -0.7431448254773863615, 0.000000000000000000 ) ) ;
#7253=EDGE_CURVE ( 'NONE', #24087, #4731, #29244, .T. ) ;
#7255=DIRECTION ( 'NONE',  ( 0.000000000000000000, 0.000000000000000000, 1.000000000000000000 ) ) ;
#7256=DIRECTION ( 'NONE',  ( -1.000000000000000000, 0.000000000000000000, 0.000000000000000000 ) ) ;
#7258=CARTESIAN_POINT ( 'NONE',  ( -0.5000000000000004441, 36.00000000000000711, 9.500000000000000000 ) ) ;
#7259=EDGE_LOOP ( 'NONE', ( #23837, #4853, #25551, #16128 ) ) ;
#7261=DIRECTION ( 'NONE',  ( -0.3535533905932645160, 0.6123724356957913617, -0.7071067811865550112 ) ) ;
#7273=EDGE_CURVE ( 'NONE', #6805, #9357, #18233, .T. ) ;
#7275=DIRECTION ( 'NONE',  ( -0.000000000000000000, -0.000000000000000000, -1.000000000000000000 ) ) ;
#7277=ORIENTED_EDGE ( 'NONE', *, *, #26619, .F. ) ;
#7279=ORIENTED_EDGE ( 'NONE', *, *, #1565, .F. ) ;
#7280=CARTESIAN_POINT ( 'NONE',  ( 13.36830325120611995, 20.48707633493483371, 7.000000000000000000 ) ) ;
#7281=ORIENTED_EDGE ( 'NONE', *, *, #30104, .T. ) ;
#7283=LINE ( 'NONE', #29033, #22583 ) ;
#7284=CYLINDRICAL_SURFACE ( 'NONE', #3117, 6.000000000000000000 ) ;
#7285=ORIENTED_EDGE ( 'NONE', *, *, #22674, .F. ) ;
#7287=LINE ( 'NONE', #1011, #4040 ) ;
#7290=VECTOR ( 'NONE', #28122, 1000.000000000000227 ) ;
#7291=EDGE_LOOP ( 'NONE', ( #17897, #11334, #21016, #1165 ) ) ;
#7294=CARTESIAN_POINT ( 'NONE',  ( 4.984135866956516558, 36.15314577889351000, 10.49999999999999822 ) ) ;
#7295=FACE_OUTER_BOUND ( 'NONE', #39339, .T. ) ;
#7300=( NAMED_UNIT ( * ) SI_UNIT ( $, .STERADIAN. ) SOLID_ANGLE_UNIT ( ) );
#7303=AXIS2_PLACEMENT_3D ( 'NONE', #18524, #30916, #5811 ) ;
#7304=DIRECTION ( 'NONE',  ( -1.000000000000000000, 0.000000000000000000, 0.000000000000000000 ) ) ;
#7306=CIRCLE ( 'NONE', #14453, 15.00000000000000000 ) ;
#7308=ORIENTED_EDGE ( 'NONE', *, *, #33845, .T. ) ;
#7309=CARTESIAN_POINT ( 'NONE',  ( 10.81260707898150386, 32.90853150812155548, 10.49999999999999822 ) ) ;
#7310=CARTESIAN_POINT ( 'NONE',  ( -4.481940917958321613, 8.628727325586488917, 7.000000000000000000 ) ) ;
#7311=VECTOR ( 'NONE', #6699, 1000.000000000000000 ) ;
#7314=CARTESIAN_POINT ( 'NONE',  ( 13.42604558747167687, 21.08886574588663620, 7.000000000000000000 ) ) ;
#7315=ORIENTED_EDGE ( 'NONE', *, *, #28199, .F. ) ;
#7317=AXIS2_PLACEMENT_3D ( 'NONE', #11846, #50, #24829 ) ;
#7320=DIRECTION ( 'NONE',  ( 0.8090169943749426773, -0.5877852522924796874, 0.000000000000000000 ) ) ;
#7321=EDGE_CURVE ( 'NONE', #36981, #38107, #13810, .T. ) ;
#7322=EDGE_LOOP ( 'NONE', ( #31173, #33965, #10379 ) ) ;
#7325=CARTESIAN_POINT ( 'NONE',  ( -9.892954722048926897, 20.95745441963943279, 10.49999999999999289 ) ) ;
#7326=CARTESIAN_POINT ( 'NONE',  ( -8.339609403135950672, 11.87216320208450959, 10.50000000000000000 ) ) ;
#7329=CARTESIAN_POINT ( 'NONE',  ( -13.63396663385394803, 16.24580510161721847, 7.000000000000000000 ) ) ;
#7330=ORIENTED_EDGE ( 'NONE', *, *, #3846, .F. ) ;
#7332=CARTESIAN_POINT ( 'NONE',  ( 8.694801740383951483, 1.741858881503469902, 11.00000000000000000 ) ) ;
#7333=DIRECTION ( 'NONE',  ( -0.000000000000000000, -0.000000000000000000, -1.000000000000000000 ) ) ;
#7334=EDGE_LOOP ( 'NONE', ( #13613, #26262, #9061 ) ) ;
#7336=DIRECTION ( 'NONE',  ( -0.000000000000000000, -0.000000000000000000, -1.000000000000000000 ) ) ;
#7339=VECTOR ( 'NONE', #16676, 1000.000000000000000 ) ;
#7340=CARTESIAN_POINT ( 'NONE',  ( -8.401171878996500197, 21.11424711454089476, 9.000000000000001776 ) ) ;
#7342=ORIENTED_EDGE ( 'NONE', *, *, #38826, .F. ) ;
#7346=ADVANCED_FACE ( 'NONE', ( #31996 ), #24591, .T. ) ;
#7348=CARTESIAN_POINT ( 'NONE',  ( -14.52509594610762456, 21.97885917798744515, 7.500000000000004441 ) ) ;
#7350=EDGE_CURVE ( 'NONE', #27233, #21190, #2139, .T. ) ;
#7354=AXIS2_PLACEMENT_3D ( 'NONE', #29756, #20621, #1729 ) ;
#7358=CARTESIAN_POINT ( 'NONE',  ( 4.678013043399745996, 44.50832101651059958, 11.00000000000000000 ) ) ;
#7361=CIRCLE ( 'NONE', #22947, 1.000000000000004441 ) ;
#7362=ORIENTED_EDGE ( 'NONE', *, *, #12790, .T. ) ;
#7365=DIRECTION ( 'NONE',  ( -0.000000000000000000, -0.000000000000000000, -1.000000000000000000 ) ) ;
#7369=CARTESIAN_POINT ( 'NONE',  ( -14.09933648065464240, 26.02968990214173317, 10.49999999999999822 ) ) ;
#7372=FACE_OUTER_BOUND ( 'NONE', #9429, .T. ) ;
#7375=CARTESIAN_POINT ( 'NONE',  ( 13.87104230352200140, 20.53934056656866147, 7.500000000000010658 ) ) ;
#7376=ADVANCED_FACE ( 'NONE', ( #14112 ), #26137, .T. ) ;
#7378=ORIENTED_EDGE ( 'NONE', *, *, #5247, .T. ) ;
#7383=ORIENTED_EDGE ( 'NONE', *, *, #24165, .F. ) ;
#7386=CARTESIAN_POINT ( 'NONE',  ( 11.54666566735224364, 32.07468077621332725, 7.000000000000000000 ) ) ;
#7387=ORIENTED_EDGE ( 'NONE', *, *, #27749, .F. ) ;
#7390=CIRCLE ( 'NONE', #28826, 0.5000000000000003331 ) ;
#7394=ADVANCED_FACE ( 'NONE', ( #17977 ), #2767, .T. ) ;
#7395=AXIS2_PLACEMENT_3D ( 'NONE', #34651, #12710, #31012 ) ;
#7396=DIRECTION ( 'NONE',  ( -0.6724985119639504960, -0.2185080122244063561, 0.7071067811865553443 ) ) ;
#7397=DIRECTION ( 'NONE',  ( -0.3090169943749589976, -0.9510565162951498674, 0.000000000000000000 ) ) ;
#7399=DIRECTION ( 'NONE',  ( -0.7431448254773862505, 0.6691306063588671194, 0.000000000000000000 ) ) ;
#7400=VECTOR ( 'NONE', #10305, 1000.000000000000000 ) ;
#7401=EDGE_CURVE ( 'NONE', #26220, #21421, #25459, .T. ) ;
#7403=CYLINDRICAL_SURFACE ( 'NONE', #33346, 5.999999999999994671 ) ;
#7405=EDGE_LOOP ( 'NONE', ( #12610, #13437, #14609 ) ) ;
#7406=CARTESIAN_POINT ( 'NONE',  ( -6.856644039074812014, 35.52575270032661336, 10.49999999999999822 ) ) ;
#7407=FACE_OUTER_BOUND ( 'NONE', #36891, .T. ) ;
#7409=DIRECTION ( 'NONE',  ( -0.9135454576426004225, 0.4067366430758009854, 0.000000000000000000 ) ) ;
#7410=CARTESIAN_POINT ( 'NONE',  ( 11.11016527260166420, 31.83082137946473367, 9.500000000000000000 ) ) ;
#7412=ORIENTED_EDGE ( 'NONE', *, *, #34849, .T. ) ;
#7414=CARTESIAN_POINT ( 'NONE',  ( 1.000000000000000000, 37.00000000000000711, 9.500000000000000000 ) ) ;
#7416=CARTESIAN_POINT ( 'NONE',  ( 8.843266739736581172, 16.81698729810774395, 11.00000000000000000 ) ) ;
#7420=B_SPLINE_SURFACE_WITH_KNOTS ( 'NONE', 1, 3, ( 
 ( #14966, #32868, #1989, #34257, #2974, #524, #12512, #3760, #9863, #19007 ),
 ( #24504, #9675, #9072, #31007, #12906, #37695, #18419, #34056, #15962, #21457 ) ),
 .UNSPECIFIED., .F., .F., .F.,
 ( 2, 2 ),
 ( 4, 2, 2, 2, 4 ),
 ( 0.000000000000000000, 1.000000000000000000 ),
 ( 1.644979861859638293, 2.037678943558364875, 2.430378025257091235, 2.823077106955818039, 3.215776188654544399 ),
 .UNSPECIFIED. ) ;
#7421=ORIENTED_EDGE ( 'NONE', *, *, #26501, .T. ) ;
#7423=CARTESIAN_POINT ( 'NONE',  ( 14.42035624161478324, 26.65972665747659676, 10.49999999999999822 ) ) ;
#7433=CARTESIAN_POINT ( 'NONE',  ( -4.984135866956331817, 36.15314577889358105, 11.00000000000000000 ) ) ;
#7434=CARTESIAN_POINT ( 'NONE',  ( -12.67417846324130259, 14.47720745114830443, 7.499999999999993783 ) ) ;
#7437=B_SPLINE_CURVE_WITH_KNOTS ( 'NONE', 3,
 ( #32670, #33277, #4825, #29607, #5429, #38953 ),
 .UNSPECIFIED., .F., .F.,
 ( 4, 2, 4 ),
 ( 0.000000000000000000, 0.5000000000000000000, 1.000000000000000000 ),
 .UNSPECIFIED. ) ;
#7438=ORIENTED_EDGE ( 'NONE', *, *, #11994, .T. ) ;
#7442=ORIENTED_EDGE ( 'NONE', *, *, #8372, .T. ) ;
#7444=CARTESIAN_POINT ( 'NONE',  ( -14.31603901957233660, 19.98981538725089990, 10.49999999999999467 ) ) ;
#7448=EDGE_CURVE ( 'NONE', #16860, #31812, #38901, .T. ) ;
#7449=ORIENTED_EDGE ( 'NONE', *, *, #6052, .T. ) ;
#7453=CARTESIAN_POINT ( 'NONE',  ( 1.590043107810628076, 12.61456814725305442, 10.49999999999999467 ) ) ;
#7454=ORIENTED_EDGE ( 'NONE', *, *, #35332, .T. ) ;
#7456=LINE ( 'NONE', #33669, #25616 ) ;
#7458=CONICAL_SURFACE ( 'NONE', #13318, 1.000000000000004441, 0.7853981633974517207 ) ;
#7459=LINE ( 'NONE', #32257, #23428 ) ;
#7461=FACE_OUTER_BOUND ( 'NONE', #34326, .T. ) ;
#7465=ORIENTED_EDGE ( 'NONE', *, *, #31511, .F. ) ;
#7467=VECTOR ( 'NONE', #29728, 1000.000000000000000 ) ;
#7468=PLANE ( 'NONE',  #14843 ) ;
#7469=CARTESIAN_POINT ( 'NONE',  ( -13.48130249190472973, 27.93180293473202980, 10.49999999999999822 ) ) ;
#7471=PLANE ( 'NONE',  #38605 ) ;
#7480=DIRECTION ( 'NONE',  ( 1.000000000000000000, 1.224646799147351235E-16, -0.000000000000000000 ) ) ;
#7482=EDGE_CURVE ( 'NONE', #10104, #24743, #35859, .T. ) ;
#7485=ORIENTED_EDGE ( 'NONE', *, *, #996, .T. ) ;
#7487=CARTESIAN_POINT ( 'NONE',  ( 15.00000000000000000, 22.50000000000000711, 0.000000000000000000 ) ) ;
#7488=VERTEX_POINT ( 'NONE', #11675 ) ;
#7490=CARTESIAN_POINT ( 'NONE',  ( -14.36830325120615548, 20.48707633493503621, 9.500000000000000000 ) ) ;
#7491=DIRECTION ( 'NONE',  ( 1.000000000000000000, -3.469446951953611033E-15, 0.000000000000000000 ) ) ;
#7492=EDGE_CURVE ( 'NONE', #30242, #37387, #21212, .T. ) ;
#7497=CIRCLE ( 'NONE', #34738, 0.5000000000000004441 ) ;
#7498=VECTOR ( 'NONE', #5343, 1000.000000000000000 ) ;
#7499=EDGE_LOOP ( 'NONE', ( #25020, #12541, #12407, #11804 ) ) ;
#7503=CARTESIAN_POINT ( 'NONE',  ( -10.81260707898136708, 32.90853150812170469, 11.00000000000000000 ) ) ;
#7505=DIRECTION ( 'NONE',  ( -1.000000000000000000, 0.000000000000000000, 0.000000000000000000 ) ) ;
#7507=CARTESIAN_POINT ( 'NONE',  ( -8.315274455032216849, 10.01576150750520888, 7.000000000000000000 ) ) ;
#7510=DIRECTION ( 'NONE',  ( 0.9510565162951504226, -0.3090169943749573322, -0.000000000000000000 ) ) ;
#7513=ORIENTED_EDGE ( 'NONE', *, *, #6012, .F. ) ;
#7515=DIRECTION ( 'NONE',  ( 0.1045284632676566766, 0.9945218953682730678, 0.000000000000000000 ) ) ;
#7518=VECTOR ( 'NONE', #20338, 1000.000000000000114 ) ;
#7519=CARTESIAN_POINT ( 'NONE',  ( -14.86556419889029357, 20.43481210330121556, 10.63089969389957545 ) ) ;
#7520=ORIENTED_EDGE ( 'NONE', *, *, #4933, .T. ) ;
#7521=CIRCLE ( 'NONE', #8166, 0.5000000000000002220 ) ;
#7523=AXIS2_PLACEMENT_3D ( 'NONE', #26770, #29820, #23525 ) ;
#7526=VECTOR ( 'NONE', #36516, 999.9999999999998863 ) ;
#7527=ADVANCED_FACE ( 'NONE', ( #20625 ), #23860, .T. ) ;
#7528=CARTESIAN_POINT ( 'NONE',  ( -9.892954722048921568, 20.95745441963943279, 10.50000000000000000 ) ) ;
#7529=ORIENTED_EDGE ( 'NONE', *, *, #32131, .T. ) ;
#7530=ORIENTED_EDGE ( 'NONE', *, *, #14496, .T. ) ;
#7533=EDGE_CURVE ( 'NONE', #25736, #8130, #17582, .T. ) ;
#7536=CARTESIAN_POINT ( 'NONE',  ( -4.940908595777639967, 35.94977745735568675, 9.500000000000000000 ) ) ;
#7539=EDGE_CURVE ( 'NONE', #13411, #17829, #39296, .T. ) ;
#7542=DIRECTION ( 'NONE',  ( 1.000000000000000000, 0.000000000000000000, 0.000000000000000000 ) ) ;
#7543=EDGE_CURVE ( 'NONE', #24016, #22931, #15117, .T. ) ;
#7544=EDGE_LOOP ( 'NONE', ( #38628, #27785, #36390, #16649, #8851 ) ) ;
#7546=DIRECTION ( 'NONE',  ( 0.000000000000000000, -0.000000000000000000, -1.000000000000000000 ) ) ;
#7547=ORIENTED_EDGE ( 'NONE', *, *, #28007, .F. ) ;
#7551=ORIENTED_EDGE ( 'NONE', *, *, #37220, .F. ) ;
#7554=CARTESIAN_POINT ( 'NONE',  ( 14.36830325120613239, 20.48707633493482660, 11.00000000000000000 ) ) ;
#7560=DIRECTION ( 'NONE',  ( -0.2876062384759434654, 0.6459741880212587217, -0.7071067811865433539 ) ) ;
#7561=EDGE_CURVE ( 'NONE', #12323, #35381, #22005, .T. ) ;
#7566=DIRECTION ( 'NONE',  ( -0.7431448254773862505, 0.6691306063588672304, 0.000000000000000000 ) ) ;
#7567=VERTEX_POINT ( 'NONE', #21803 ) ;
#7569=EDGE_LOOP ( 'NONE', ( #816, #3331, #39784, #16057 ) ) ;
#7577=ORIENTED_EDGE ( 'NONE', *, *, #24739, .T. ) ;
#7579=DIRECTION ( 'NONE',  ( -1.000000000000000000, 0.000000000000000000, 0.000000000000000000 ) ) ;
#7581=ADVANCED_FACE ( 'NONE', ( #12066 ), #37050, .T. ) ;
#7582=CARTESIAN_POINT ( 'NONE',  ( 12.34742388243071964, 14.79386122849051155, 11.00000000000000000 ) ) ;
#7587=CYLINDRICAL_SURFACE ( 'NONE', #38419, 0.5000000000000004441 ) ;
#7591=DIRECTION ( 'NONE',  ( -0.2079116908177663092, -0.9781476007338042455, 0.000000000000000000 ) ) ;
#7593=VERTEX_POINT ( 'NONE', #28098 ) ;
#7598=EDGE_LOOP ( 'NONE', ( #10632, #18395, #19344, #39125 ) ) ;
#7601=CARTESIAN_POINT ( 'NONE',  ( -14.57486473880221745, 26.18419839932921533, 10.50000000000000000 ) ) ;
#7602=DIRECTION ( 'NONE',  ( -0.1045284632676570929, -0.9945218953682730678, 0.000000000000000000 ) ) ;
#7603=EDGE_CURVE ( 'NONE', #7885, #25412, #15313, .T. ) ;
#7606=LINE ( 'NONE', #39090, #38943 ) ;
#7608=LINE ( 'NONE', #22640, #21136 ) ;
#7614=DIRECTION ( 'NONE',  ( -0.000000000000000000, -0.000000000000000000, -1.000000000000000000 ) ) ;
#7615=CARTESIAN_POINT ( 'NONE',  ( -11.07315816304227774, 31.12468366354675808, 9.500000000000000000 ) ) ;
#7617=VECTOR ( 'NONE', #32443, 1000.000000000000000 ) ;
#7619=EDGE_LOOP ( 'NONE', ( #2923, #38133, #16100, #37772 ) ) ;
#7623=DIRECTION ( 'NONE',  ( 1.000000000000000000, 0.000000000000000000, 0.000000000000000000 ) ) ;
#7625=ORIENTED_EDGE ( 'NONE', *, *, #33229, .F. ) ;
#7627=VERTEX_POINT ( 'NONE', #24455 ) ;
#7636=VERTEX_POINT ( 'NONE', #277 ) ;
#7640=DIRECTION ( 'NONE',  ( 0.000000000000000000, 0.000000000000000000, 1.000000000000000000 ) ) ;
#7642=AXIS2_PLACEMENT_3D ( 'NONE', #14384, #26771, #39161 ) ;
#7643=VERTEX_POINT ( 'NONE', #39889 ) ;
#7645=VECTOR ( 'NONE', #11996, 1000.000000000000000 ) ;
#7651=CARTESIAN_POINT ( 'NONE',  ( 11.11016527260166420, 31.83082137946473367, 7.000000000000000000 ) ) ;
#7652=VECTOR ( 'NONE', #38988, 1000.000000000000000 ) ;
#7656=AXIS2_PLACEMENT_3D ( 'NONE', #31480, #21730, #37581 ) ;
#7658=DIRECTION ( 'NONE',  ( -1.000000000000000000, 0.000000000000000000, 0.000000000000000000 ) ) ;
#7660=ADVANCED_FACE ( 'NONE', ( #3518 ), #36852, .T. ) ;
#7662=DIRECTION ( 'NONE',  ( -1.000000000000000000, -1.224646799147353947E-16, 0.000000000000000000 ) ) ;
#7663=VERTEX_POINT ( 'NONE', #9024 ) ;
#7665=DIRECTION ( 'NONE',  ( -0.000000000000000000, -0.000000000000000000, -1.000000000000000000 ) ) ;
#7666=CARTESIAN_POINT ( 'NONE',  ( 14.11133924723984379, 27.61078317377175750, 10.49999999999999822 ) ) ;
#7670=VECTOR ( 'NONE', #14151, 1000.000000000000114 ) ;
#7672=DIRECTION ( 'NONE',  ( -0.000000000000000000, -0.000000000000000000, -1.000000000000000000 ) ) ;
#7677=FACE_OUTER_BOUND ( 'NONE', #14358, .T. ) ;
#7679=FACE_OUTER_BOUND ( 'NONE', #22830, .T. ) ;
#7684=EDGE_CURVE ( 'NONE', #36577, #34387, #77, .T. ) ;
#7685=CONICAL_SURFACE ( 'NONE', #20011, 1.000000000000000444, 0.7853981633974482790 ) ;
#7691=LINE ( 'NONE', #29226, #18615 ) ;
#7694=ORIENTED_EDGE ( 'NONE', *, *, #38411, .T. ) ;
#7695=CARTESIAN_POINT ( 'NONE',  ( 2.525645716490518833, 8.212903943950921715, 7.000000000000000000 ) ) ;
#7698=CARTESIAN_POINT ( 'NONE',  ( -8.195318570657255108, 10.36946087849385378, 11.00000000000000000 ) ) ;
#7699=ORIENTED_EDGE ( 'NONE', *, *, #33414, .T. ) ;
#7701=VERTEX_POINT ( 'NONE', #9625 ) ;
#7703=AXIS2_PLACEMENT_3D ( 'NONE', #13373, #17040, #1596 ) ;
#7709=CARTESIAN_POINT ( 'NONE',  ( -5.034171952701850472, 35.03623199971307400, 9.500000000000000000 ) ) ;
#7710=DIRECTION ( 'NONE',  ( -0.9510565162951503115, 0.3090169943749573878, -0.000000000000000000 ) ) ;
#7712=CARTESIAN_POINT ( 'NONE',  ( -11.61633080063096379, 31.93537370176186840, 10.49999999999999467 ) ) ;
#7713=VERTEX_POINT ( 'NONE', #18766 ) ;
#7714=CARTESIAN_POINT ( 'NONE',  ( -11.48173768534023154, 32.16538668264431777, 11.00000000000000000 ) ) ;
#7717=DIRECTION ( 'NONE',  ( -0.000000000000000000, -0.000000000000000000, -1.000000000000000000 ) ) ;
#7720=VERTEX_POINT ( 'NONE', #31349 ) ;
#7725=DIRECTION ( 'NONE',  ( -0.000000000000000000, -0.000000000000000000, -1.000000000000000000 ) ) ;
#7726=VECTOR ( 'NONE', #6807, 1000.000000000000000 ) ;
#7731=CARTESIAN_POINT ( 'NONE',  ( -7.530592408761010326, 11.28437794979203268, 9.500000000000000000 ) ) ;
#7732=ORIENTED_EDGE ( 'NONE', *, *, #20844, .T. ) ;
#7734=AXIS2_PLACEMENT_3D ( 'NONE', #22948, #22540, #3862 ) ;
#7736=FACE_OUTER_BOUND ( 'NONE', #32776, .T. ) ;
#7739=DIRECTION ( 'NONE',  ( 0.000000000000000000, 0.000000000000000000, 1.000000000000000000 ) ) ;
#7740=ORIENTED_EDGE ( 'NONE', *, *, #21958, .T. ) ;
#7742=CARTESIAN_POINT ( 'NONE',  ( -10.61811999842798038, 32.73341455422775681, 10.94387467463492847 ) ) ;
#7743=CARTESIAN_POINT ( 'NONE',  ( -14.63635198741550347, 25.78286467897752487, 7.000000000000000000 ) ) ;
#7744=DIRECTION ( 'NONE',  ( -0.000000000000000000, -0.000000000000000000, -1.000000000000000000 ) ) ;
#7747=DIRECTION ( 'NONE',  ( -0.4999999999999920064, 0.8660254037844432595, 0.000000000000000000 ) ) ;
#7752=ORIENTED_EDGE ( 'NONE', *, *, #2916, .F. ) ;
#7755=DIRECTION ( 'NONE',  ( -1.000000000000000000, 0.000000000000000000, 0.000000000000000000 ) ) ;
#7758=DIRECTION ( 'NONE',  ( -0.000000000000000000, -0.000000000000000000, -1.000000000000000000 ) ) ;
#7760=EDGE_CURVE ( 'NONE', #28177, #35442, #7306, .T. ) ;
#7761=CARTESIAN_POINT ( 'NONE',  ( 14.47283171447379146, 21.48159823030311344, 11.00000000000000000 ) ) ;
#7764=DIRECTION ( 'NONE',  ( -1.000000000000000000, 0.000000000000000000, 0.000000000000000000 ) ) ;
#7765=ADVANCED_FACE ( 'NONE', ( #26609 ), #38467, .T. ) ;
#7767=ADVANCED_FACE ( 'NONE', ( #38399 ), #17725, .T. ) ;
#7771=DIRECTION ( 'NONE',  ( 1.000000000000000000, 0.000000000000000000, 0.000000000000000000 ) ) ;
#7777=CARTESIAN_POINT ( 'NONE',  ( -14.42035624161472640, 26.65972665747679216, 10.49999999999999822 ) ) ;
#7779=EDGE_LOOP ( 'NONE', ( #38746, #29521, #5886, #8980 ) ) ;
#7783=CARTESIAN_POINT ( 'NONE',  ( 13.63581098909226519, 27.45627467658428600, 11.00000000000000000 ) ) ;
#7785=FACE_OUTER_BOUND ( 'NONE', #19336, .T. ) ;
#7786=VECTOR ( 'NONE', #35156, 1000.000000000000000 ) ;
#7787=VERTEX_POINT ( 'NONE', #4270 ) ;
#7796=CARTESIAN_POINT ( 'NONE',  ( -11.87435565298220830, 15.06698729810789139, 9.500000000000000000 ) ) ;
#7797=ADVANCED_FACE ( 'NONE', ( #10574 ), #10774, .T. ) ;
#7798=AXIS2_PLACEMENT_3D ( 'NONE', #22841, #3754, #31791 ) ;
#7803=VERTEX_POINT ( 'NONE', #39003 ) ;
#7806=DIRECTION ( 'NONE',  ( 1.000000000000000000, 0.000000000000000000, 0.000000000000000000 ) ) ;
#7808=DIRECTION ( 'NONE',  ( -1.000000000000000000, 0.000000000000000000, 0.000000000000000000 ) ) ;
#7809=EDGE_CURVE ( 'NONE', #12521, #17600, #5080, .T. ) ;
#7811=DIRECTION ( 'NONE',  ( -0.1045284632676437842, 0.9945218953682744001, 0.000000000000000000 ) ) ;
#7812=CARTESIAN_POINT ( 'NONE',  ( 1.100969307443724343, 12.51061230184417816, 10.49999999999999467 ) ) ;
#7813=ORIENTED_EDGE ( 'NONE', *, *, #8412, .T. ) ;
#7819=CARTESIAN_POINT ( 'NONE',  ( -14.60528968261104055, 20.46216805729389066, 10.94387467463490360 ) ) ;
#7821=ORIENTED_EDGE ( 'NONE', *, *, #35727, .F. ) ;
#7823=DIRECTION ( 'NONE',  ( -0.9510565162951544194, -0.3090169943749450643, 0.000000000000000000 ) ) ;
#7837=ORIENTED_EDGE ( 'NONE', *, *, #37876, .F. ) ;
#7839=VECTOR ( 'NONE', #13705, 1000.000000000000000 ) ;
#7848=DIRECTION ( 'NONE',  ( 0.9876883405951395467, 0.1564344650402197390, 0.000000000000000000 ) ) ;
#7849=AXIS2_PLACEMENT_3D ( 'NONE', #36156, #39793, #17880 ) ;
#7858=CARTESIAN_POINT ( 'NONE',  ( 6.451376067921989588, 35.76073122305122354, 10.94387467463335639 ) ) ;
#7863=CARTESIAN_POINT ( 'NONE',  ( 14.06009009443824986, 27.59413131461127833, 10.76099332938163577 ) ) ;
#7864=FACE_OUTER_BOUND ( 'NONE', #9694, .T. ) ;
#7866=LINE ( 'NONE', #22901, #8008 ) ;
#7868=DIRECTION ( 'NONE',  ( 0.6691306063588569053, -0.7431448254773954654, 0.000000000000000000 ) ) ;
#7869=EDGE_LOOP ( 'NONE', ( #27521, #19781, #7308, #24719 ) ) ;
#7872=DIRECTION ( 'NONE',  ( -0.9781476007338042455, 0.2079116908177663370, 0.000000000000000000 ) ) ;
#7875=DIRECTION ( 'NONE',  ( 0.9135454576426059736, 0.4067366430757889395, -0.000000000000000000 ) ) ;
#7878=PLANE ( 'NONE',  #25877 ) ;
#7883=CARTESIAN_POINT ( 'NONE',  ( -3.713592597587352717, 7.966960743906856379, 7.499999999999997335 ) ) ;
#7884=EDGE_CURVE ( 'NONE', #11472, #12432, #2041, .T. ) ;
#7885=VERTEX_POINT ( 'NONE', #8119 ) ;
#7888=EDGE_LOOP ( 'NONE', ( #17702, #12787, #29692 ) ) ;
#7890=AXIS2_PLACEMENT_3D ( 'NONE', #15013, #8923, #2824 ) ;
#7892=EDGE_LOOP ( 'NONE', ( #10844, #5182, #6489, #16210 ) ) ;
#7893=VECTOR ( 'NONE', #29846, 1000.000000000000000 ) ;
#7894=FACE_OUTER_BOUND ( 'NONE', #15800, .T. ) ;
#7895=DIRECTION ( 'NONE',  ( -1.000000000000000000, 0.000000000000000000, 0.000000000000000000 ) ) ;
#7898=VERTEX_POINT ( 'NONE', #1635 ) ;
#7903=CARTESIAN_POINT ( 'NONE',  ( 13.48130249190479191, 27.93180293473185927, 10.50000000000000533 ) ) ;
#7904=ORIENTED_EDGE ( 'NONE', *, *, #24739, .F. ) ;
#7905=DIRECTION ( 'NONE',  ( 0.000000000000000000, 0.000000000000000000, -1.000000000000000000 ) ) ;
#7907=EDGE_CURVE ( 'NONE', #32385, #1779, #11245, .T. ) ;
#7909=DIRECTION ( 'NONE',  ( 0.7431448254773953543, 0.6691306063588570163, 0.000000000000000000 ) ) ;
#7910=VERTEX_POINT ( 'NONE', #38805 ) ;
#7912=( LENGTH_UNIT ( ) NAMED_UNIT ( * ) SI_UNIT ( .MILLI., .METRE. ) );
#7918=ORIENTED_EDGE ( 'NONE', *, *, #13621, .F. ) ;
#7919=DIRECTION ( 'NONE',  ( 0.3090169943749450643, -0.9510565162951544194, 0.000000000000000000 ) ) ;
#7920=CARTESIAN_POINT ( 'NONE',  ( -2.363107919609845009, 7.722275577009013681, 10.49999999999999467 ) ) ;
#7923=LINE ( 'NONE', #39007, #24383 ) ;
#7924=ORIENTED_EDGE ( 'NONE', *, *, #21335, .T. ) ;
#7928=CARTESIAN_POINT ( 'NONE',  ( 1.000000000000000222, 36.00000000000000711, 9.500000000000000000 ) ) ;
#7930=VERTEX_POINT ( 'NONE', #26002 ) ;
#7934=VECTOR ( 'NONE', #22321, 1000.000000000000000 ) ;
#7936=LINE ( 'NONE', #23180, #23487 ) ;
#7937=ORIENTED_EDGE ( 'NONE', *, *, #14773, .F. ) ;
#7940=DIRECTION ( 'NONE',  ( -0.6691306063588560171, 0.7431448254773962425, 0.000000000000000000 ) ) ;
#7948=AXIS2_PLACEMENT_3D ( 'NONE', #37253, #21413, #2536 ) ;
#7950=ORIENTED_EDGE ( 'NONE', *, *, #29798, .T. ) ;
#7953=DIRECTION ( 'NONE',  ( 1.000000000000000000, 0.000000000000000000, 0.000000000000000000 ) ) ;
#7957=VECTOR ( 'NONE', #30892, 1000.000000000000000 ) ;
#7958=LINE ( 'NONE', #29702, #35092 ) ;
#7961=DIRECTION ( 'NONE',  ( 0.000000000000000000, 0.000000000000000000, -1.000000000000000000 ) ) ;
#7964=CARTESIAN_POINT ( 'NONE',  ( 5.440908595777814050, 35.94977745735560859, 7.000000000000000000 ) ) ;
#7965=CARTESIAN_POINT ( 'NONE',  ( -13.24038105676664401, 15.43301270189234309, 10.50000000000000355 ) ) ;
#7968=CIRCLE ( 'NONE', #30052, 6.000000000000003553 ) ;
#7970=ORIENTED_EDGE ( 'NONE', *, *, #7045, .F. ) ;
#7973=CARTESIAN_POINT ( 'NONE',  ( 13.63581098909227052, 27.45627467658428600, 9.500000000000000000 ) ) ;
#7975=VERTEX_POINT ( 'NONE', #1842 ) ;
#7977=ORIENTED_EDGE ( 'NONE', *, *, #26033, .T. ) ;
#7979=LINE ( 'NONE', #1906, #2409 ) ;
#7981=CARTESIAN_POINT ( 'NONE',  ( 0.000000000000000000, 22.50000000000000355, 7.000000000000000000 ) ) ;
#7986=LINE ( 'NONE', #14490, #28060 ) ;
#7990=EDGE_CURVE ( 'NONE', #11320, #9704, #31622, .T. ) ;
#7991=LINE ( 'NONE', #17559, #39457 ) ;
#7994=ORIENTED_EDGE ( 'NONE', *, *, #16600, .F. ) ;
#7997=AXIS2_PLACEMENT_3D ( 'NONE', #15656, #6693, #22337 ) ;
#8000=EDGE_LOOP ( 'NONE', ( #22407, #31886, #21543, #39311 ) ) ;
#8002=EDGE_CURVE ( 'NONE', #11250, #31137, #8526, .T. ) ;
#8004=CIRCLE ( 'NONE', #39147, 0.5000000000000004441 ) ;
#8005=DIRECTION ( 'NONE',  ( -0.4999999999999921729, 0.8660254037844432595, 0.000000000000000000 ) ) ;
#8008=VECTOR ( 'NONE', #35302, 1000.000000000000114 ) ;
#8009=DIRECTION ( 'NONE',  ( -0.4067366430757888285, 0.9135454576426059736, -0.000000000000000000 ) ) ;
#8010=CARTESIAN_POINT ( 'NONE',  ( 0.000000000000000000, 22.50000000000000355, 0.000000000000000000 ) ) ;
#8012=ORIENTED_EDGE ( 'NONE', *, *, #26918, .T. ) ;
#8015=ADVANCED_FACE ( 'NONE', ( #39603 ), #30270, .T. ) ;
#8016=FACE_OUTER_BOUND ( 'NONE', #39782, .T. ) ;
#8018=LINE ( 'NONE', #17789, #26820 ) ;
#8023=AXIS2_PLACEMENT_3D ( 'NONE', #7709, #35345, #16660 ) ;
#8027=DIRECTION ( 'NONE',  ( -0.000000000000000000, -0.000000000000000000, 1.000000000000000000 ) ) ;
#8030=CARTESIAN_POINT ( 'NONE',  ( -14.52509594610762278, 21.97885917798745226, 10.49999999999999822 ) ) ;
#8033=DIRECTION ( 'NONE',  ( -0.000000000000000000, -0.000000000000000000, 1.000000000000000000 ) ) ;
#8041=LINE ( 'NONE', #36088, #30996 ) ;
#8046=EDGE_CURVE ( 'NONE', #10907, #38994, #31990, .T. ) ;
#8048=LINE ( 'NONE', #32853, #11820 ) ;
#8051=DIRECTION ( 'NONE',  ( -0.9945218953682744001, -0.1045284632676437564, 0.000000000000000000 ) ) ;
#8052=ADVANCED_FACE ( 'NONE', ( #11777 ), #2438, .F. ) ;
#8053=LINE ( 'NONE', #26744, #29421 ) ;
#8056=CONICAL_SURFACE ( 'NONE', #30770, 0.5000000000000046629, 0.7853981633974503884 ) ;
#8058=LINE ( 'NONE', #4615, #7400 ) ;
#8059=PLANE ( 'NONE',  #37001 ) ;
#8061=CONICAL_SURFACE ( 'NONE', #38542, 0.5000000000000108802, 0.7853981633974482790 ) ;
#8065=CARTESIAN_POINT ( 'NONE',  ( -13.94482798346716201, 26.50521816028930644, 7.000000000000000000 ) ) ;
#8066=ADVANCED_FACE ( 'NONE', ( #2633 ), #17689, .T. ) ;
#8067=LINE ( 'NONE', #33475, #12156 ) ;
#8068=DIRECTION ( 'NONE',  ( 0.5877852522924796874, 0.8090169943749426773, 0.000000000000000000 ) ) ;
#8072=CARTESIAN_POINT ( 'NONE',  ( 14.52509594610761923, 21.97885917798724975, 7.000000000000000000 ) ) ;
#8075=CARTESIAN_POINT ( 'NONE',  ( 14.26584774442731884, 27.13525491562417713, 7.000000000000000000 ) ) ;
#8076=CARTESIAN_POINT ( 'NONE',  ( -0.4999999999999998890, 37.00000000000000711, 10.99999999999999645 ) ) ;
#8080=DIRECTION ( 'NONE',  ( -1.000000000000000000, 0.000000000000000000, 0.000000000000000000 ) ) ;
#8081=FACE_OUTER_BOUND ( 'NONE', #22730, .T. ) ;
#8088=EDGE_LOOP ( 'NONE', ( #26285, #32721, #26591, #27744 ) ) ;
#8092=CARTESIAN_POINT ( 'NONE',  ( -0.4999999999999998890, 37.50000000000000711, 11.00000000000000000 ) ) ;
#8094=DIRECTION ( 'NONE',  ( -0.9135454576426059736, -0.4067366430757889395, 0.000000000000000000 ) ) ;
#8095=DIRECTION ( 'NONE',  ( 0.6724985119639536046, -0.2185080122244175416, -0.7071067811865489050 ) ) ;
#8100=VECTOR ( 'NONE', #17847, 1000.000000000000000 ) ;
#8101=VERTEX_POINT ( 'NONE', #5008 ) ;
#8103=ORIENTED_EDGE ( 'NONE', *, *, #35561, .T. ) ;
#8104=DIRECTION ( 'NONE',  ( -1.000000000000000000, 0.000000000000000000, 0.000000000000000000 ) ) ;
#8105=CIRCLE ( 'NONE', #34073, 0.5000000000000002220 ) ;
#8106=CARTESIAN_POINT ( 'NONE',  ( -7.096882951594430722, 29.56287847632736288, 10.49999999999999822 ) ) ;
#8109=CARTESIAN_POINT ( 'NONE',  ( -3.963760424820539363, 8.194319839800240146, 10.49999999999999467 ) ) ;
#8114=DIRECTION ( 'NONE',  ( 0.1045284632676569680, 0.9945218953682729568, -0.000000000000000000 ) ) ;
#8115=EDGE_CURVE ( 'NONE', #38307, #3978, #23700, .T. ) ;
#8119=CARTESIAN_POINT ( 'NONE',  ( -9.831584923911583118, 26.22020669908462764, 10.00000000000000000 ) ) ;
#8120=CARTESIAN_POINT ( 'NONE',  ( -2.629601561899595374, 7.723830143584053509, 10.49999999999999822 ) ) ;
#8122=PLANE ( 'NONE',  #35982 ) ;
#8123=B_SPLINE_CURVE_WITH_KNOTS ( 'NONE', 3,
 ( #902, #38275, #34824, #16341 ),
 .UNSPECIFIED., .F., .F.,
 ( 4, 4 ),
 ( 0.6666666663583977748, 1.000000000000000000 ),
 .UNSPECIFIED. ) ;
#8124=DIRECTION ( 'NONE',  ( 0.5000000000000043299, 0.8660254037844361541, 0.000000000000000000 ) ) ;
#8125=VECTOR ( 'NONE', #20543, 999.9999999999998863 ) ;
#8129=DIRECTION ( 'NONE',  ( -0.000000000000000000, -0.000000000000000000, -1.000000000000000000 ) ) ;
#8130=VERTEX_POINT ( 'NONE', #32242 ) ;
#8131=VERTEX_POINT ( 'NONE', #32450 ) ;
#8133=VECTOR ( 'NONE', #38506, 1000.000000000000000 ) ;
#8134=DIRECTION ( 'NONE',  ( -0.9945218953682745111, -0.1045284632676436454, 0.000000000000000000 ) ) ;
#8139=AXIS2_PLACEMENT_3D ( 'NONE', #12588, #31081, #31279 ) ;
#8141=ORIENTED_EDGE ( 'NONE', *, *, #39373, .F. ) ;
#8144=CARTESIAN_POINT ( 'NONE',  ( 8.927394655428276593, 11.06314620770945290, 7.500000000000000888 ) ) ;
#8145=CARTESIAN_POINT ( 'NONE',  ( -8.593266739736661108, 16.38397459621564067, 10.50000000000000000 ) ) ;
#8146=CARTESIAN_POINT ( 'NONE',  ( -5.362728154696096539, 13.41753630677062148, 10.50000000000000711 ) ) ;
#8149=CARTESIAN_POINT ( 'NONE',  ( -13.60579549876895911, 27.97225316470548862, 10.49999999999999822 ) ) ;
#8152=EDGE_CURVE ( 'NONE', #13390, #4137, #1769, .T. ) ;
#8155=MANIFOLD_SOLID_BREP ( 'Boss-Extrude2', #19662 ) ;
#8158=CARTESIAN_POINT ( 'NONE',  ( -10.36702044712414938, 31.16169077310601665, 10.50000000000000000 ) ) ;
#8160=CARTESIAN_POINT ( 'NONE',  ( 8.718890067807359756, 5.003589289612210500, 10.00000000000000000 ) ) ;
#8161=ORIENTED_EDGE ( 'NONE', *, *, #2172, .F. ) ;
#8162=DIRECTION ( 'NONE',  ( 0.5877852522924691403, -0.8090169943749503378, -6.938893903907234689E-15 ) ) ;
#8163=CIRCLE ( 'NONE', #20505, 15.00000000000000000 ) ;
#8164=EDGE_CURVE ( 'NONE', #38004, #29091, #38531, .T. ) ;
#8166=AXIS2_PLACEMENT_3D ( 'NONE', #11333, #20479, #20273 ) ;
#8169=DIRECTION ( 'NONE',  ( -0.6691306063588569053, 0.7431448254773954654, 0.000000000000000000 ) ) ;
#8173=DIRECTION ( 'NONE',  ( -0.000000000000000000, -0.000000000000000000, -1.000000000000000000 ) ) ;
#8174=CARTESIAN_POINT ( 'NONE',  ( -13.21633681164003171, 15.44689465328864486, 10.68306113187833084 ) ) ;
#8187=DIRECTION ( 'NONE',  ( -0.9510565162951497564, 0.3090169943749591086, -3.469446951953608667E-15 ) ) ;
#8189=ADVANCED_FACE ( 'NONE', ( #23301 ), #26551, .T. ) ;
#8195=ORIENTED_EDGE ( 'NONE', *, *, #6787, .T. ) ;
#8198=DIRECTION ( 'NONE',  ( -0.000000000000000000, -0.000000000000000000, -1.000000000000000000 ) ) ;
#8201=ORIENTED_EDGE ( 'NONE', *, *, #12790, .F. ) ;
#8203=B_SPLINE_CURVE_WITH_KNOTS ( 'NONE', 3,
 ( #27273, #31120, #21177, #18730, #33781, #36814 ),
 .UNSPECIFIED., .F., .F.,
 ( 4, 2, 4 ),
 ( 0.1333333595060078314, 0.5666666797530039990, 1.000000000000000000 ),
 .UNSPECIFIED. ) ;
#8205=TOROIDAL_SURFACE ( 'NONE', #28315, 1.000000000000000000, 0.5000000000000000000 ) ;
#8208=EDGE_LOOP ( 'NONE', ( #39982, #740, #203 ) ) ;
#8211=CARTESIAN_POINT ( 'NONE',  ( 14.81901435602781802, 20.17583222033112733, 7.455539900862803826 ) ) ;
#8212=FACE_OUTER_BOUND ( 'NONE', #3229, .T. ) ;
#8213=DIRECTION ( 'NONE',  ( 0.4067366430757888840, -0.9135454576426058626, -0.000000000000000000 ) ) ;
#8215=CARTESIAN_POINT ( 'NONE',  ( 12.63581098909226341, 27.45627467658428955, 7.000000000000000000 ) ) ;
#8216=EDGE_LOOP ( 'NONE', ( #33894, #16935, #17059, #27761 ) ) ;
#8219=CARTESIAN_POINT ( 'NONE',  ( -12.80736835487442349, 15.68301270189233954, 7.000000000000000000 ) ) ;
#8221=EDGE_CURVE ( 'NONE', #11661, #32239, #20056, .T. ) ;
#8222=LINE ( 'NONE', #39098, #5393 ) ;
#8223=PLANE ( 'NONE',  #11264 ) ;
#8225=CIRCLE ( 'NONE', #3035, 0.5000000000000015543 ) ;
#8227=EDGE_LOOP ( 'NONE', ( #22984, #24437, #12555 ) ) ;
#8231=DIRECTION ( 'NONE',  ( -0.000000000000000000, -0.000000000000000000, -1.000000000000000000 ) ) ;
#8237=FACE_OUTER_BOUND ( 'NONE', #18181, .T. ) ;
#8242=DIRECTION ( 'NONE',  ( 0.6691306063588671194, 0.7431448254773863615, -0.000000000000000000 ) ) ;
#8247=CARTESIAN_POINT ( 'NONE',  ( 6.151085731882511176, 35.08626808545850650, 7.500000000000000000 ) ) ;
#8248=CARTESIAN_POINT ( 'NONE',  ( -9.356056665764020508, 26.06569820189716324, 10.50000000000000533 ) ) ;
#8249=ORIENTED_EDGE ( 'NONE', *, *, #20447, .F. ) ;
#8252=DIRECTION ( 'NONE',  ( 1.000000000000000000, 0.000000000000000000, 0.000000000000000000 ) ) ;
#8254=DIRECTION ( 'NONE',  ( -0.000000000000000000, -0.000000000000000000, 1.000000000000000000 ) ) ;
#8255=ADVANCED_FACE ( 'NONE', ( #17216 ), #29590, .T. ) ;
#8256=FILL_AREA_STYLE ('',( #23496 ) ) ;
#8257=PLANE ( 'NONE',  #6940 ) ;
#8260=ORIENTED_EDGE ( 'NONE', *, *, #10994, .T. ) ;
#8261=CARTESIAN_POINT ( 'NONE',  ( 14.99496371230769931, 22.09054546458561674, 7.203056206335837430 ) ) ;
#8262=AXIS2_PLACEMENT_3D ( 'NONE', #24137, #8905, #15997 ) ;
#8264=CARTESIAN_POINT ( 'NONE',  ( 6.807850151676529293, 35.76876263333484474, 10.49999999999999822 ) ) ;
#8265=LINE ( 'NONE', #29803, #24851 ) ;
#8267=DIRECTION ( 'NONE',  ( -0.2876062384759483503, -0.6459741880212440668, 0.7071067811865547892 ) ) ;
#8268=EDGE_CURVE ( 'NONE', #29799, #16943, #8053, .T. ) ;
#8269=DIRECTION ( 'NONE',  ( 1.000000000000000000, 0.000000000000000000, 0.000000000000000000 ) ) ;
#8270=DIRECTION ( 'NONE',  ( 0.5720614028176917998, 0.4156269377774556295, 0.7071067811865402453 ) ) ;
#8272=CARTESIAN_POINT ( 'NONE',  ( 12.30736835487432757, 14.81698729810772441, 7.499999999999997335 ) ) ;
#8273=EDGE_CURVE ( 'NONE', #9944, #4851, #28203, .T. ) ;
#8276=FACE_OUTER_BOUND ( 'NONE', #20752, .T. ) ;
#8280=EDGE_CURVE ( 'NONE', #24136, #11401, #3464, .T. ) ;
#8281=CARTESIAN_POINT ( 'NONE',  ( -14.11133924723977628, 27.61078317377193159, 10.49999999999999822 ) ) ;
#8283=EDGE_CURVE ( 'NONE', #21540, #23024, #34584, .T. ) ;
#8284=CARTESIAN_POINT ( 'NONE',  ( -14.11133924723978517, 27.61078317377194580, 10.63089969389956835 ) ) ;
#8286=LINE ( 'NONE', #5240, #2357 ) ;
#8288=AXIS2_PLACEMENT_3D ( 'NONE', #22980, #25622, #38021 ) ;
#8289=CIRCLE ( 'NONE', #26465, 0.5000000000000004441 ) ;
#8298=CIRCLE ( 'NONE', #10878, 1.000000000000004441 ) ;
#8299=ORIENTED_EDGE ( 'NONE', *, *, #16305, .F. ) ;
#8301=CIRCLE ( 'NONE', #31002, 0.5000000000000004441 ) ;
#8304=ORIENTED_EDGE ( 'NONE', *, *, #1407, .T. ) ;
#8307=ADVANCED_FACE ( 'NONE', ( #979 ), #25749, .T. ) ;
#8308=CARTESIAN_POINT ( 'NONE',  ( 9.426561227484755889, 11.13126706419770073, 10.49999999999999822 ) ) ;
#8309=EDGE_CURVE ( 'NONE', #37532, #39789, #2173, .T. ) ;
#8314=VERTEX_POINT ( 'NONE', #37948 ) ;
#8319=VECTOR ( 'NONE', #33506, 1000.000000000000000 ) ;
#8324=LINE ( 'NONE', #39989, #16303 ) ;
#8325=AXIS2_PLACEMENT_3D ( 'NONE', #10864, #35650, #7806 ) ;
#8326=CARTESIAN_POINT ( 'NONE',  ( -2.421689871081829537, 8.701977744317861863, 7.499999999999997335 ) ) ;
#8327=ADVANCED_FACE ( 'NONE', ( #12763 ), #24958, .F. ) ;
#8329=VECTOR ( 'NONE', #23591, 1000.000000000000000 ) ;
#8333=CARTESIAN_POINT ( 'NONE',  ( 10.53831209642084943, 32.66155519649334593, 11.00000000000000178 ) ) ;
#8334=DIRECTION ( 'NONE',  ( 0.000000000000000000, 0.000000000000000000, 1.000000000000000000 ) ) ;
#8337=LINE ( 'NONE', #11584, #17268 ) ;
#8341=CARTESIAN_POINT ( 'NONE',  ( -9.303655249773276736, 10.73386218874833631, 7.500000000000000888 ) ) ;
#8342=ORIENTED_EDGE ( 'NONE', *, *, #24492, .F. ) ;
#8345=PLANE ( 'NONE',  #9442 ) ;
#8346=CARTESIAN_POINT ( 'NONE',  ( -12.23768179954928392, 14.31935546172410412, 10.49999999999999822 ) ) ;
#8347=CIRCLE ( 'NONE', #25212, 15.00000000000000000 ) ;
#8349=CARTESIAN_POINT ( 'NONE',  ( -15.02235689379176087, 21.92659494635362449, 10.49999999999999822 ) ) ;
#8350=ORIENTED_EDGE ( 'NONE', *, *, #30112, .F. ) ;
#8352=DIRECTION ( 'NONE',  ( 0.000000000000000000, 0.000000000000000000, 1.000000000000000000 ) ) ;
#8353=CYLINDRICAL_SURFACE ( 'NONE', #31711, 0.5000000000000001110 ) ;
#8356=AXIS2_PLACEMENT_3D ( 'NONE', #36842, #30153, #5764 ) ;
#8359=DIRECTION ( 'NONE',  ( 0.000000000000000000, 0.000000000000000000, 1.000000000000000000 ) ) ;
#8360=EDGE_LOOP ( 'NONE', ( #15103, #27841, #22949 ) ) ;
#8371=DIRECTION ( 'NONE',  ( 0.1470157664651937091, -0.6916548014802239575, -0.7071067811865501263 ) ) ;
#8372=EDGE_CURVE ( 'NONE', #37754, #17829, #6352, .T. ) ;
#8373=VECTOR ( 'NONE', #30438, 1000.000000000000000 ) ;
#8375=AXIS2_PLACEMENT_3D ( 'NONE', #5233, #14782, #23324 ) ;
#8376=CARTESIAN_POINT ( 'NONE',  ( 12.05736835487432579, 14.38397459621550567, 11.00000000000000000 ) ) ;
#8377=EDGE_CURVE ( 'NONE', #17859, #11555, #21903, .T. ) ;
#8383=CARTESIAN_POINT ( 'NONE',  ( 2.575189371470594235, 7.979819372998081306, 10.94387467463492492 ) ) ;
#8386=ORIENTED_EDGE ( 'NONE', *, *, #8309, .F. ) ;
#8388=EDGE_CURVE ( 'NONE', #17187, #37715, #25350, .T. ) ;
#8390=CARTESIAN_POINT ( 'NONE',  ( 3.994223993665185546, 8.041403552485290263, 7.382773698552457020 ) ) ;
#8392=ORIENTED_EDGE ( 'NONE', *, *, #32277, .T. ) ;
#8394=ORIENTED_EDGE ( 'NONE', *, *, #22580, .T. ) ;
#8399=VERTEX_POINT ( 'NONE', #10120 ) ;
#8402=CARTESIAN_POINT ( 'NONE',  ( 0.000000000000000000, 22.50000000000000355, 7.000000000000000000 ) ) ;
#8403=ORIENTED_EDGE ( 'NONE', *, *, #9769, .F. ) ;
#8405=DIRECTION ( 'NONE',  ( -0.000000000000000000, -0.000000000000000000, -1.000000000000000000 ) ) ;
#8407=EDGE_CURVE ( 'NONE', #31812, #4123, #11190, .T. ) ;
#8409=EDGE_CURVE ( 'NONE', #747, #24654, #28802, .T. ) ;
#8412=EDGE_CURVE ( 'NONE', #13055, #5349, #3621, .T. ) ;
#8417=DIRECTION ( 'NONE',  ( 0.7431448254773953543, 0.6691306063588570163, 0.000000000000000000 ) ) ;
#8418=CARTESIAN_POINT ( 'NONE',  ( 14.83020139230451662, 20.24804233373097873, 7.485699520496988946 ) ) ;
#8420=EDGE_CURVE ( 'NONE', #17593, #27237, #33357, .T. ) ;
#8421=LINE ( 'NONE', #14511, #33130 ) ;
#8422=CARTESIAN_POINT ( 'NONE',  ( 6.557822374958316658, 35.99981354310111215, 10.49999999999999822 ) ) ;
#8424=PLANE ( 'NONE',  #12026 ) ;
#8425=ORIENTED_EDGE ( 'NONE', *, *, #38771, .F. ) ;
#8428=CARTESIAN_POINT ( 'NONE',  ( -1.838889047819898037, 31.15129278236396360, 7.000000000000000000 ) ) ;
#8431=CARTESIAN_POINT ( 'NONE',  ( -14.31603901957233660, 19.98981538725089635, 10.49999999999999822 ) ) ;
#8435=ORIENTED_EDGE ( 'NONE', *, *, #32229, .T. ) ;
#8438=CARTESIAN_POINT ( 'NONE',  ( -0.6108529249776363246, 37.48755679569042343, 7.000000000000000000 ) ) ;
#8440=ORIENTED_EDGE ( 'NONE', *, *, #25743, .F. ) ;
#8441=CARTESIAN_POINT ( 'NONE',  ( -14.97986028244562107, 21.52226669793691727, 10.49999999999999822 ) ) ;
#8442=AXIS2_PLACEMENT_3D ( 'NONE', #2032, #1832, #27399 ) ;
#8445=LINE ( 'NONE', #4790, #1719 ) ;
#8447=DIRECTION ( 'NONE',  ( -0.000000000000000000, -0.000000000000000000, -1.000000000000000000 ) ) ;
#8450=DIRECTION ( 'NONE',  ( 0.000000000000000000, -0.000000000000000000, 1.000000000000000000 ) ) ;
#8456=FACE_OUTER_BOUND ( 'NONE', #27339, .T. ) ;
#8460=CARTESIAN_POINT ( 'NONE',  ( -14.36830325120615548, 20.48707633493503621, 7.500000000000004441 ) ) ;
#8462=FACE_OUTER_BOUND ( 'NONE', #18004, .T. ) ;
#8465=ORIENTED_EDGE ( 'NONE', *, *, #2639, .F. ) ;
#8466=B_SPLINE_CURVE_WITH_KNOTS ( 'NONE', 3,
 ( #12712, #28753, #928, #6416, #12913, #3373 ),
 .UNSPECIFIED., .F., .F.,
 ( 4, 2, 4 ),
 ( 0.000000000000000000, 0.3333333331791988874, 0.6666666663583977748 ),
 .UNSPECIFIED. ) ;
#8467=CONICAL_SURFACE ( 'NONE', #36367, 0.5000000000000069944, 0.7853981633974450594 ) ;
#8469=CARTESIAN_POINT ( 'NONE',  ( 6.811226782241717181, 35.33967249274190436, 10.49999999999999822 ) ) ;
#8472=DIRECTION ( 'NONE',  ( -0.4731467892558149924, 0.5254827454987555102, 0.7071067811865500152 ) ) ;
#8476=DIRECTION ( 'NONE',  ( 0.5000000000000015543, 0.8660254037844377084, 0.000000000000000000 ) ) ;
#8477=CARTESIAN_POINT ( 'NONE',  ( -6.811226782241547539, 35.33967249274200384, 10.49999999999999822 ) ) ;
#8479=CARTESIAN_POINT ( 'NONE',  ( 12.80736835487433289, 15.68301270189216545, 7.499999999999997335 ) ) ;
#8480=ORIENTED_EDGE ( 'NONE', *, *, #22198, .F. ) ;
#8484=DIRECTION ( 'NONE',  ( 0.6691306063588570163, -0.7431448254773953543, 0.000000000000000000 ) ) ;
#8485=VECTOR ( 'NONE', #37102, 1000.000000000000000 ) ;
#8489=FACE_OUTER_BOUND ( 'NONE', #30174, .T. ) ;
#8496=EDGE_LOOP ( 'NONE', ( #35047, #14933, #28934 ) ) ;
#8499=ORIENTED_EDGE ( 'NONE', *, *, #12564, .F. ) ;
#8503=EDGE_CURVE ( 'NONE', #14734, #39078, #248, .T. ) ;
#8504=CARTESIAN_POINT ( 'NONE',  ( 9.353067506536371312, 10.78869951827618046, 10.49999999999999822 ) ) ;
#8507=AXIS2_PLACEMENT_3D ( 'NONE', #7106, #25004, #15462 ) ;
#8509=VECTOR ( 'NONE', #13244, 1000.000000000000000 ) ;
#8511=DIRECTION ( 'NONE',  ( -0.5000000000000038858, -0.8660254037844364872, 0.000000000000000000 ) ) ;
#8512=ORIENTED_EDGE ( 'NONE', *, *, #35460, .T. ) ;
#8513=EDGE_CURVE ( 'NONE', #16864, #20155, #13628, .T. ) ;
#8514=DIRECTION ( 'NONE',  ( -1.000000000000000000, 0.000000000000000000, 0.000000000000000000 ) ) ;
#8515=CARTESIAN_POINT ( 'NONE',  ( -9.427394655428429360, 11.06314620770957013, 11.00000000000000000 ) ) ;
#8516=CARTESIAN_POINT ( 'NONE',  ( -11.94134295108998600, 16.18301270189233776, 9.500000000000000000 ) ) ;
#8517=ORIENTED_EDGE ( 'NONE', *, *, #33999, .T. ) ;
#8518=LINE ( 'NONE', #24358, #2292 ) ;
#8519=DIRECTION ( 'NONE',  ( -0.7431448254773953543, -0.6691306063588570163, 0.000000000000000000 ) ) ;
#8520=TOROIDAL_SURFACE ( 'NONE', #33187, 1.000000000000000000, 0.5000000000000000000 ) ;
#8521=LINE ( 'NONE', #8326, #55 ) ;
#8524=VERTEX_POINT ( 'NONE', #26565 ) ;
#8526=LINE ( 'NONE', #20733, #19670 ) ;
#8527=CARTESIAN_POINT ( 'NONE',  ( -7.659620408498105881, 26.92228390473685096, 7.000000000000000000 ) ) ;
#8528=EDGE_CURVE ( 'NONE', #16847, #14003, #7361, .T. ) ;
#8529=EDGE_CURVE ( 'NONE', #32217, #19954, #26359, .T. ) ;
#8531=CARTESIAN_POINT ( 'NONE',  ( -13.14827996435949053, 25.72067290776677950, 10.50000000000000000 ) ) ;
#8534=AXIS2_PLACEMENT_3D ( 'NONE', #32518, #22951, #13406 ) ;
#8537=DIRECTION ( 'NONE',  ( -1.000000000000000000, 0.000000000000000000, 0.000000000000000000 ) ) ;
#8539=ORIENTED_EDGE ( 'NONE', *, *, #28099, .T. ) ;
#8543=CARTESIAN_POINT ( 'NONE',  ( -12.05736835487443059, 14.38397459621567087, 10.49999999999999822 ) ) ;
#8544=DIRECTION ( 'NONE',  ( 0.1045284632676559550, 0.9945218953682730678, 0.000000000000000000 ) ) ;
#8547=CARTESIAN_POINT ( 'NONE',  ( 10.44103466624280685, 32.57396620494213124, 7.000000000000000000 ) ) ;
#8548=CIRCLE ( 'NONE', #26049, 1.000000000000000888 ) ;
#8549=DIRECTION ( 'NONE',  ( 1.000000000000000000, 0.000000000000000000, 0.000000000000000000 ) ) ;
#8553=FACE_OUTER_BOUND ( 'NONE', #30194, .T. ) ;
#8554=VERTEX_POINT ( 'NONE', #13561 ) ;
#8557=ORIENTED_EDGE ( 'NONE', *, *, #29266, .T. ) ;
#8560=CARTESIAN_POINT ( 'NONE',  ( 12.30736835487432579, 14.81698729810772619, 9.000000000000001776 ) ) ;
#8564=DIRECTION ( 'NONE',  ( -0.9781476007338067991, -0.2079116908177533474, 0.000000000000000000 ) ) ;
#8565=LINE ( 'NONE', #36210, #9810 ) ;
#8572=DIRECTION ( 'NONE',  ( -0.4067366430757889395, 0.9135454576426059736, 0.000000000000000000 ) ) ;
#8573=DIRECTION ( 'NONE',  ( -0.8064441531181035794, 0.1277282058446102819, 0.5773502691896329475 ) ) ;
#8575=VERTEX_POINT ( 'NONE', #16827 ) ;
#8577=ORIENTED_EDGE ( 'NONE', *, *, #26018, .T. ) ;
#8579=AXIS2_PLACEMENT_3D ( 'NONE', #9940, #6479, #37571 ) ;
#8582=CARTESIAN_POINT ( 'NONE',  ( -3.987511920225224937, 8.280017797930396384, 10.49999999999999822 ) ) ;
#8584=ORIENTED_EDGE ( 'NONE', *, *, #11565, .F. ) ;
#8586=EDGE_LOOP ( 'NONE', ( #11516, #18612, #24429 ) ) ;
#8588=DIRECTION ( 'NONE',  ( -0.3090169943749573322, -0.9510565162951505336, 0.000000000000000000 ) ) ;
#8590=CARTESIAN_POINT ( 'NONE',  ( 8.927394655428274817, 11.06314620770945290, 7.000000000000000000 ) ) ;
#8597=ORIENTED_EDGE ( 'NONE', *, *, #9116, .T. ) ;
#8600=CARTESIAN_POINT ( 'NONE',  ( 8.118377661053324701, 10.47536095541698486, 7.000000000000000000 ) ) ;
#8602=ORIENTED_EDGE ( 'NONE', *, *, #8152, .F. ) ;
#8605=ORIENTED_EDGE ( 'NONE', *, *, #14748, .T. ) ;
#8609=AXIS2_PLACEMENT_3D ( 'NONE', #36469, #14934, #27322 ) ;
#8613=DIRECTION ( 'NONE',  ( -0.8660254037844431485, -0.4999999999999921729, 0.000000000000000000 ) ) ;
#8614=ADVANCED_FACE ( 'NONE', ( #38752 ), #16624, .F. ) ;
#8617=CARTESIAN_POINT ( 'NONE',  ( -14.97009266215794554, 21.42933399866948463, 10.50000000000000000 ) ) ;
#8619=CARTESIAN_POINT ( 'NONE',  ( -11.61999097910615930, 31.98625350855128247, 7.479114585244767355 ) ) ;
#8623=DIRECTION ( 'NONE',  ( -1.000000000000000000, 0.000000000000000000, 0.000000000000000000 ) ) ;
#8624=DIRECTION ( 'NONE',  ( -0.000000000000000000, -0.000000000000000000, -1.000000000000000000 ) ) ;
#8626=EDGE_CURVE ( 'NONE', #40197, #21179, #29208, .T. ) ;
#8628=EDGE_CURVE ( 'NONE', #38824, #31959, #7866, .T. ) ;
#8630=VECTOR ( 'NONE', #25807, 1000.000000000000000 ) ;
#8638=CYLINDRICAL_SURFACE ( 'NONE', #5359, 0.5000000000000004441 ) ;
#8639=ORIENTED_EDGE ( 'NONE', *, *, #30031, .T. ) ;
#8641=DIRECTION ( 'NONE',  ( 0.7032331762534055342, 0.07391278520357008608, -0.7071067811865457964 ) ) ;
#8643=CARTESIAN_POINT ( 'NONE',  ( 9.221287281574507944, 10.65863771052197606, 10.63089969389957190 ) ) ;
#8644=AXIS2_PLACEMENT_3D ( 'NONE', #25587, #31889, #12800 ) ;
#8649=ORIENTED_EDGE ( 'NONE', *, *, #15507, .F. ) ;
#8651=LINE ( 'NONE', #21045, #10911 ) ;
#8653=DIRECTION ( 'NONE',  ( 0.9781476007338042455, -0.2079116908177664758, 0.000000000000000000 ) ) ;
#8656=ADVANCED_FACE ( 'NONE', ( #7461 ), #1379, .T. ) ;
#8657=AXIS2_PLACEMENT_3D ( 'NONE', #328, #37300, #33673 ) ;
#8659=DIRECTION ( 'NONE',  ( 0.000000000000000000, 0.000000000000000000, 1.000000000000000000 ) ) ;
#8660=VECTOR ( 'NONE', #5817, 1000.000000000000114 ) ;
#8667=ORIENTED_EDGE ( 'NONE', *, *, #38159, .T. ) ;
#8668=CARTESIAN_POINT ( 'NONE',  ( -15.00000000000000000, 22.50000000000000355, 7.000000000000000000 ) ) ;
#8673=CARTESIAN_POINT ( 'NONE',  ( -4.984135866956331817, 36.15314577889358105, 10.50000000000000533 ) ) ;
#8674=DIRECTION ( 'NONE',  ( 1.000000000000000000, 0.000000000000000000, 0.000000000000000000 ) ) ;
#8676=EDGE_CURVE ( 'NONE', #4778, #30884, #19064, .T. ) ;
#8679=DIRECTION ( 'NONE',  ( 0.000000000000000000, 0.000000000000000000, 1.000000000000000000 ) ) ;
#8682=LINE ( 'NONE', #15171, #30155 ) ;
#8686=VECTOR ( 'NONE', #5125, 1000.000000000000114 ) ;
#8691=VERTEX_POINT ( 'NONE', #30618 ) ;
#8692=CARTESIAN_POINT ( 'NONE',  ( 1.693998953219503667, 12.12549434688615513, 10.50000000000000000 ) ) ;
#8694=AXIS2_PLACEMENT_3D ( 'NONE', #8477, #2777, #27758 ) ;
#8699=CARTESIAN_POINT ( 'NONE',  ( 12.23327497914553597, 13.81973598992451713, 7.000000000000000000 ) ) ;
#8701=EDGE_LOOP ( 'NONE', ( #22685, #14837, #26602, #25476 ) ) ;
#8702=AXIS2_PLACEMENT_3D ( 'NONE', #35293, #966, #10711 ) ;
#8703=DIRECTION ( 'NONE',  ( -0.9781476007338042455, 0.2079116908177663647, 0.000000000000000000 ) ) ;
#8704=ORIENTED_EDGE ( 'NONE', *, *, #36880, .F. ) ;
#8706=PLANE ( 'NONE',  #30969 ) ;
#8707=CARTESIAN_POINT ( 'NONE',  ( -6.354454053420243831, 35.54304081427989814, 7.500000000000000888 ) ) ;
#8709=B_SPLINE_CURVE_WITH_KNOTS ( 'NONE', 3,
 ( #29317, #29917, #35817, #29719, #8390, #17747, #14683, #13878 ),
 .UNSPECIFIED., .F., .F.,
 ( 4, 2, 2, 4 ),
 ( 0.000000000000000000, 0.0004726692273637063640, 0.0007090038410455602779, 0.0009453384547274142459 ),
 .UNSPECIFIED. ) ;
#8712=ORIENTED_EDGE ( 'NONE', *, *, #4405, .F. ) ;
#8715=DIRECTION ( 'NONE',  ( -0.000000000000000000, -0.000000000000000000, -1.000000000000000000 ) ) ;
#8716=DIRECTION ( 'NONE',  ( 0.000000000000000000, 0.000000000000000000, -1.000000000000000000 ) ) ;
#8717=AXIS2_PLACEMENT_3D ( 'NONE', #7964, #30316, #10826 ) ;
#8718=CARTESIAN_POINT ( 'NONE',  ( 11.19134295108988830, 14.88397459621551100, 10.50000000000000000 ) ) ;
#8719=VERTEX_POINT ( 'NONE', #33867 ) ;
#8721=CARTESIAN_POINT ( 'NONE',  ( -3.992867117591420545, 8.524771480177605554, 10.50000000000000533 ) ) ;
#8723=CARTESIAN_POINT ( 'NONE',  ( 0.000000000000000000, 22.50000000000000355, 7.000000000000000000 ) ) ;
#8727=TOROIDAL_SURFACE ( 'NONE', #11345, 1.000000000000000000, 0.5000000000000000000 ) ;
#8728=EDGE_LOOP ( 'NONE', ( #28105, #28795, #8999, #4578, #36428 ) ) ;
#8730=DIRECTION ( 'NONE',  ( 0.9781476007338069101, 0.2079116908177532363, 0.000000000000000000 ) ) ;
#8731=LINE ( 'NONE', #11976, #25049 ) ;
#8732=EDGE_CURVE ( 'NONE', #31582, #32385, #26196, .T. ) ;
#8735=EDGE_CURVE ( 'NONE', #8719, #13029, #15367, .T. ) ;
#8740=CARTESIAN_POINT ( 'NONE',  ( 11.58359689081945021, 32.01076807263225987, 10.49999999999999822 ) ) ;
#8742=ORIENTED_EDGE ( 'NONE', *, *, #22009, .T. ) ;
#8746=FACE_OUTER_BOUND ( 'NONE', #37062, .T. ) ;
#8748=LINE ( 'NONE', #5891, #26701 ) ;
#8749=VERTEX_POINT ( 'NONE', #33077 ) ;
#8751=CARTESIAN_POINT ( 'NONE',  ( 11.48173768534036121, 32.16538668264416145, 10.49999999999999822 ) ) ;
#8753=ORIENTED_EDGE ( 'NONE', *, *, #34014, .T. ) ;
#8756=DIRECTION ( 'NONE',  ( -1.000000000000000000, 0.000000000000000000, 0.000000000000000000 ) ) ;
#8760=ORIENTED_EDGE ( 'NONE', *, *, #4408, .F. ) ;
#8766=DIRECTION ( 'NONE',  ( 0.000000000000000000, 0.000000000000000000, 1.000000000000000000 ) ) ;
#8768=CARTESIAN_POINT ( 'NONE',  ( 1.828660225305865250, 9.087095699275852922, 10.00000000000000000 ) ) ;
#8771=DIRECTION ( 'NONE',  ( 0.07391278520356048265, 0.7032331762534029806, 0.7071067811865493491 ) ) ;
#8773=EDGE_CURVE ( 'NONE', #16261, #6733, #27360, .T. ) ;
#8775=DIRECTION ( 'NONE',  ( 1.224646799147351235E-16, -1.000000000000000000, 0.000000000000000000 ) ) ;
#8776=AXIS2_PLACEMENT_3D ( 'NONE', #28561, #19414, #32009 ) ;
#8777=DIRECTION ( 'NONE',  ( 0.3090169943749573878, 0.9510565162951503115, 0.000000000000000000 ) ) ;
#8778=CARTESIAN_POINT ( 'NONE',  ( 2.606860170653414244, 7.830819977571334078, 10.82238861112336714 ) ) ;
#8783=VECTOR ( 'NONE', #32815, 1000.000000000000114 ) ;
#8788=ADVANCED_FACE ( 'NONE', ( #24113 ), #39551, .T. ) ;
#8791=ADVANCED_FACE ( 'NONE', ( #36315 ), #20877, .T. ) ;
#8792=ORIENTED_EDGE ( 'NONE', *, *, #3316, .F. ) ;
#8796=CARTESIAN_POINT ( 'NONE',  ( -6.868154521567742421, 35.60001939699343865, 10.49999999999999822 ) ) ;
#8803=EDGE_LOOP ( 'NONE', ( #22277, #39704, #11451, #20806 ) ) ;
#8809=EDGE_LOOP ( 'NONE', ( #4323, #22463, #6589, #9829 ) ) ;
#8812=EDGE_CURVE ( 'NONE', #11532, #7488, #19182, .T. ) ;
#8813=ORIENTED_EDGE ( 'NONE', *, *, #450, .F. ) ;
#8815=EDGE_CURVE ( 'NONE', #11592, #36019, #35282, .T. ) ;
#8816=VECTOR ( 'NONE', #37460, 1000.000000000000000 ) ;
#8817=CARTESIAN_POINT ( 'NONE',  ( -10.62272290917004192, 33.09068932351447501, 7.455539900862802938 ) ) ;
#8818=CARTESIAN_POINT ( 'NONE',  ( 5.139519228946050511, 36.36965741570532629, 10.49999999999999822 ) ) ;
#8819=DIRECTION ( 'NONE',  ( -0.000000000000000000, -0.000000000000000000, -1.000000000000000000 ) ) ;
#8820=CARTESIAN_POINT ( 'NONE',  ( 7.935100905948329064, 11.57827057593817344, 7.000000000000000000 ) ) ;
#8825=CARTESIAN_POINT ( 'NONE',  ( -6.811226782241549316, 35.33967249274201095, 10.49999999999999822 ) ) ;
#8830=EDGE_CURVE ( 'NONE', #17580, #17841, #25106, .T. ) ;
#8833=ORIENTED_EDGE ( 'NONE', *, *, #38942, .F. ) ;
#8838=ORIENTED_EDGE ( 'NONE', *, *, #5168, .F. ) ;
#8840=VERTEX_POINT ( 'NONE', #5227 ) ;
#8843=LINE ( 'NONE', #25070, #38685 ) ;
#8845=DIRECTION ( 'NONE',  ( -0.4067366430757919926, 0.9135454576426046414, 0.000000000000000000 ) ) ;
#8846=VECTOR ( 'NONE', #942, 999.9999999999998863 ) ;
#8849=CARTESIAN_POINT ( 'NONE',  ( 12.80736835487433289, 15.68301270189216545, 9.000000000000001776 ) ) ;
#8851=ORIENTED_EDGE ( 'NONE', *, *, #13621, .T. ) ;
#8853=VECTOR ( 'NONE', #36916, 1000.000000000000114 ) ;
#8855=DIRECTION ( 'NONE',  ( -0.6691306063588672304, -0.7431448254773862505, 0.000000000000000000 ) ) ;
#8856=CARTESIAN_POINT ( 'NONE',  ( 4.678013043399745996, 44.50832101651059958, 7.000000000000000000 ) ) ;
#8860=DIRECTION ( 'NONE',  ( 0.9135454576426005335, -0.4067366430758009299, 0.000000000000000000 ) ) ;
#8871=CARTESIAN_POINT ( 'NONE',  ( -5.644276917315534270, 36.40655018617698602, 10.49999999999999822 ) ) ;
#8872=DIRECTION ( 'NONE',  ( 0.8660254037844432595, 0.4999999999999921729, 0.000000000000000000 ) ) ;
#8873=DIRECTION ( 'NONE',  ( 0.9135454576426005335, -0.4067366430758008744, 0.000000000000000000 ) ) ;
#8874=DIRECTION ( 'NONE',  ( -0.9945218953682742891, -0.1045284632676437425, 0.000000000000000000 ) ) ;
#8875=CYLINDRICAL_SURFACE ( 'NONE', #28733, 0.5000000000000004441 ) ;
#8879=CARTESIAN_POINT ( 'NONE',  ( 9.821458659721804096, 11.16186433357816910, 7.102637441331451917 ) ) ;
#8882=CARTESIAN_POINT ( 'NONE',  ( 9.665073660139015033, 25.11464168560187460, 10.49999999999999822 ) ) ;
#8883=DIRECTION ( 'NONE',  ( 0.4999999999999920064, -0.8660254037844432595, 0.000000000000000000 ) ) ;
#8884=EDGE_CURVE ( 'NONE', #13564, #15556, #4117, .T. ) ;
#8889=ORIENTED_EDGE ( 'NONE', *, *, #7128, .T. ) ;
#8890=CARTESIAN_POINT ( 'NONE',  ( -2.317734025672945286, 9.191051544684766483, 10.00000000000000000 ) ) ;
#8897=FACE_OUTER_BOUND ( 'NONE', #35463, .T. ) ;
#8899=ORIENTED_EDGE ( 'NONE', *, *, #23183, .T. ) ;
#8902=CONICAL_SURFACE ( 'NONE', #28375, 0.4999999999999970024, 0.7853981633974447263 ) ;
#8904=ORIENTED_EDGE ( 'NONE', *, *, #28856, .T. ) ;
#8905=DIRECTION ( 'NONE',  ( -0.7431448254773863615, 0.6691306063588671194, 0.000000000000000000 ) ) ;
#8906=DIRECTION ( 'NONE',  ( 0.6729908358753765585, 0.000000000000000000, 0.7396508195275403041 ) ) ;
#8907=ADVANCED_FACE ( 'NONE', ( #3570 ), #10067, .F. ) ;
#8908=VECTOR ( 'NONE', #3209, 999.9999999999998863 ) ;
#8912=EDGE_CURVE ( 'NONE', #29040, #4287, #34855, .T. ) ;
#8915=PLANE ( 'NONE',  #25195 ) ;
#8916=VERTEX_POINT ( 'NONE', #15966 ) ;
#8918=DIRECTION ( 'NONE',  ( 1.000000000000000000, 0.000000000000000000, 0.000000000000000000 ) ) ;
#8919=DIRECTION ( 'NONE',  ( 0.9135454576426059736, 0.4067366430757889395, -0.000000000000000000 ) ) ;
#8920=ORIENTED_EDGE ( 'NONE', *, *, #6400, .F. ) ;
#8922=CARTESIAN_POINT ( 'NONE',  ( -9.736411649803377699, 11.65093146000205770, 7.000000000000000000 ) ) ;
#8923=DIRECTION ( 'NONE',  ( 0.000000000000000000, 0.000000000000000000, -1.000000000000000000 ) ) ;
#8924=CYLINDRICAL_SURFACE ( 'NONE', #7849, 0.5000000000000005551 ) ;
#8926=EDGE_CURVE ( 'NONE', #20981, #7910, #1481, .T. ) ;
#8928=AXIS2_PLACEMENT_3D ( 'NONE', #2705, #39276, #36637 ) ;
#8930=AXIS2_PLACEMENT_3D ( 'NONE', #2952, #34037, #6385 ) ;
#8933=DIRECTION ( 'NONE',  ( 0.000000000000000000, 0.000000000000000000, -1.000000000000000000 ) ) ;
#8934=EDGE_CURVE ( 'NONE', #23537, #35497, #11963, .T. ) ;
#8936=DIRECTION ( 'NONE',  ( 1.000000000000000000, 0.000000000000000000, 0.000000000000000000 ) ) ;
#8937=AXIS2_PLACEMENT_3D ( 'NONE', #2572, #20864, #24300 ) ;
#8942=CARTESIAN_POINT ( 'NONE',  ( 11.50946345163907836, 31.52577281809587717, 10.49999999999999822 ) ) ;
#8944=ORIENTED_EDGE ( 'NONE', *, *, #24546, .F. ) ;
#8947=CARTESIAN_POINT ( 'NONE',  ( -11.44134295108998245, 15.31698729810788251, 7.000000000000000000 ) ) ;
#8948=LINE ( 'NONE', #33747, #13735 ) ;
#8949=ORIENTED_EDGE ( 'NONE', *, *, #1205, .T. ) ;
#8952=DIRECTION ( 'NONE',  ( -0.000000000000000000, -0.000000000000000000, 1.000000000000000000 ) ) ;
#8953=CONICAL_SURFACE ( 'NONE', #3746, 1.000000000000002665, 0.7853981633974543852 ) ;
#8954=ORIENTED_EDGE ( 'NONE', *, *, #33389, .T. ) ;
#8957=ORIENTED_EDGE ( 'NONE', *, *, #25566, .T. ) ;
#8959=AXIS2_PLACEMENT_3D ( 'NONE', #27634, #18301, #18696 ) ;
#8961=ORIENTED_EDGE ( 'NONE', *, *, #5090, .F. ) ;
#8964=TOROIDAL_SURFACE ( 'NONE', #20664, 1.000000000000000000, 0.5000000000000000000 ) ;
#8966=B_SPLINE_CURVE_WITH_KNOTS ( 'NONE', 3,
 ( #3171, #21453, #37293, #2971 ),
 .UNSPECIFIED., .F., .F.,
 ( 4, 4 ),
 ( 0.000000000000000000, 1.000000000000000000 ),
 .UNSPECIFIED. ) ;
#8967=LINE ( 'NONE', #30302, #34464 ) ;
#8969=VECTOR ( 'NONE', #21534, 1000.000000000000000 ) ;
#8970=CARTESIAN_POINT ( 'NONE',  ( -3.531008893910706714, 8.292776413244068223, 11.00000000000000355 ) ) ;
#8971=ORIENTED_EDGE ( 'NONE', *, *, #21797, .F. ) ;
#8977=CYLINDRICAL_SURFACE ( 'NONE', #30758, 0.5000000000000000000 ) ;
#8978=DIRECTION ( 'NONE',  ( -1.000000000000000000, 0.000000000000000000, 0.000000000000000000 ) ) ;
#8980=ORIENTED_EDGE ( 'NONE', *, *, #37188, .F. ) ;
#8987=ORIENTED_EDGE ( 'NONE', *, *, #16350, .T. ) ;
#8988=ORIENTED_EDGE ( 'NONE', *, *, #36476, .T. ) ;
#8989=AXIS2_PLACEMENT_3D ( 'NONE', #13698, #1726, #7808 ) ;
#8994=AXIS2_PLACEMENT_3D ( 'NONE', #5455, #17862, #21097 ) ;
#8998=CARTESIAN_POINT ( 'NONE',  ( 0.5000000000000000000, 37.13089969389957901, 11.00000000000000355 ) ) ;
#8999=ORIENTED_EDGE ( 'NONE', *, *, #39624, .T. ) ;
#9001=CARTESIAN_POINT ( 'NONE',  ( -0.5000000000000004441, 37.00000000000000711, 7.500000000000000888 ) ) ;
#9002=CARTESIAN_POINT ( 'NONE',  ( 8.411683849014126579, 19.76687823897103868, 9.000000000000001776 ) ) ;
#9003=VERTEX_POINT ( 'NONE', #3178 ) ;
#9005=ORIENTED_EDGE ( 'NONE', *, *, #9813, .F. ) ;
#9009=ORIENTED_EDGE ( 'NONE', *, *, #11946, .F. ) ;
#9011=CARTESIAN_POINT ( 'NONE',  ( 14.86556419889027048, 20.43481210330100240, 11.00000000000000000 ) ) ;
#9012=CARTESIAN_POINT ( 'NONE',  ( 14.47283171447379146, 21.48159823030311344, 7.000000000000000000 ) ) ;
#9013=AXIS2_PLACEMENT_3D ( 'NONE', #23592, #23787, #14243 ) ;
#9017=EDGE_CURVE ( 'NONE', #11250, #26597, #15763, .T. ) ;
#9021=CARTESIAN_POINT ( 'NONE',  ( -5.396718838163291565, 36.49572678120085811, 7.455539900862802050 ) ) ;
#9022=ORIENTED_EDGE ( 'NONE', *, *, #36962, .T. ) ;
#9024=CARTESIAN_POINT ( 'NONE',  ( 8.744117900323280068, 12.16605582823063791, 10.50000000000000000 ) ) ;
#9025=CARTESIAN_POINT ( 'NONE',  ( 14.42035624161478857, 26.65972665747660031, 7.000000000000000000 ) ) ;
#9030=EDGE_LOOP ( 'NONE', ( #20448, #36548, #25426, #34755 ) ) ;
#9041=FACE_OUTER_BOUND ( 'NONE', #5358, .T. ) ;
#9043=CARTESIAN_POINT ( 'NONE',  ( -3.153820973115281312, 32.04219121950185212, 10.50000000000000533 ) ) ;
#9045=AXIS2_PLACEMENT_3D ( 'NONE', #1999, #20484, #30430 ) ;
#9048=DIRECTION ( 'NONE',  ( -1.000000000000000000, 0.000000000000000000, 0.000000000000000000 ) ) ;
#9050=ORIENTED_EDGE ( 'NONE', *, *, #1461, .F. ) ;
#9055=VECTOR ( 'NONE', #38592, 1000.000000000000000 ) ;
#9056=ORIENTED_EDGE ( 'NONE', *, *, #28865, .T. ) ;
#9061=ORIENTED_EDGE ( 'NONE', *, *, #19718, .F. ) ;
#9062=EDGE_CURVE ( 'NONE', #25521, #11885, #4149, .T. ) ;
#9064=CARTESIAN_POINT ( 'NONE',  ( 0.4999999999999995559, 37.00000000000000711, 11.00000000000000000 ) ) ;
#9065=EDGE_LOOP ( 'NONE', ( #18325, #34333, #16018, #2256 ) ) ;
#9067=VECTOR ( 'NONE', #34057, 1000.000000000000000 ) ;
#9071=CARTESIAN_POINT ( 'NONE',  ( 4.980911888400610721, 31.22871793335020385, 10.49999999999999822 ) ) ;
#9072=CARTESIAN_POINT ( 'NONE',  ( 14.83795255154715598, 20.43771420437945352, 10.68306085400105943 ) ) ;
#9073=DIRECTION ( 'NONE',  ( 0.000000000000000000, 0.000000000000000000, -1.000000000000000000 ) ) ;
#9074=AXIS2_PLACEMENT_3D ( 'NONE', #38540, #26144, #10714 ) ;
#9075=CARTESIAN_POINT ( 'NONE',  ( 9.221287281574507944, 10.65863771052197784, 7.000000000000000000 ) ) ;
#9077=DIRECTION ( 'NONE',  ( -1.000000000000000000, 0.000000000000000000, 0.000000000000000000 ) ) ;
#9080=ORIENTED_EDGE ( 'NONE', *, *, #5484, .T. ) ;
#9089=VERTEX_POINT ( 'NONE', #4726 ) ;
#9097=DIRECTION ( 'NONE',  ( 0.4999999999999930056, -0.8660254037844428154, 0.000000000000000000 ) ) ;
#9104=DIRECTION ( 'NONE',  ( 0.000000000000000000, 0.000000000000000000, -1.000000000000000000 ) ) ;
#9105=AXIS2_PLACEMENT_3D ( 'NONE', #15958, #19003, #3955 ) ;
#9107=ADVANCED_FACE ( 'NONE', ( #32770 ), #17133, .T. ) ;
#9109=EDGE_CURVE ( 'NONE', #38623, #10038, #2486, .T. ) ;
#9110=ORIENTED_EDGE ( 'NONE', *, *, #6439, .F. ) ;
#9111=CARTESIAN_POINT ( 'NONE',  ( 7.353987181296509412, 35.57359447655183970, 7.000000000000000000 ) ) ;
#9112=ORIENTED_EDGE ( 'NONE', *, *, #30569, .T. ) ;
#9113=FACE_OUTER_BOUND ( 'NONE', #35329, .T. ) ;
#9115=AXIS2_PLACEMENT_3D ( 'NONE', #8820, #21206, #33613 ) ;
#9116=EDGE_CURVE ( 'NONE', #10226, #31380, #23214, .T. ) ;
#9120=CARTESIAN_POINT ( 'NONE',  ( -4.503793317224517700, 8.420815634768723967, 7.000000000000000000 ) ) ;
#9122=CARTESIAN_POINT ( 'NONE',  ( 19.48557158514997667, 33.74999999999982236, 11.00000000000000000 ) ) ;
#9134=B_SPLINE_CURVE_WITH_KNOTS ( 'NONE', 3,
 ( #24479, #101, #12090, #24678, #36875, #37072 ),
 .UNSPECIFIED., .F., .F.,
 ( 4, 2, 4 ),
 ( 0.06666641432897602026, 0.5333332071644880656, 1.000000000000000000 ),
 .UNSPECIFIED. ) ;
#9135=ADVANCED_FACE ( 'NONE', ( #39249 ), #33382, .T. ) ;
#9139=CARTESIAN_POINT ( 'NONE',  ( 11.25022250131758383, 31.95692947463369649, 10.96580508970282608 ) ) ;
#9142=CARTESIAN_POINT ( 'NONE',  ( 1.000000000000000444, 37.00000000000000711, 10.49999999999999822 ) ) ;
#9143=CARTESIAN_POINT ( 'NONE',  ( -7.713869163866016621, 10.18146832927085121, 10.50000000000000711 ) ) ;
#9144=CIRCLE ( 'NONE', #28592, 15.00000000000000000 ) ;
#9148=VECTOR ( 'NONE', #6797, 1000.000000000000114 ) ;
#9150=PLANE ( 'NONE',  #40058 ) ;
#9151=ORIENTED_EDGE ( 'NONE', *, *, #39624, .F. ) ;
#9153=CARTESIAN_POINT ( 'NONE',  ( 13.94482798346721175, 26.50521816028912525, 7.000000000000000000 ) ) ;
#9155=ORIENTED_EDGE ( 'NONE', *, *, #17474, .T. ) ;
#9157=ADVANCED_FACE ( 'NONE', ( #23617 ), #9986, .T. ) ;
#9158=EDGE_CURVE ( 'NONE', #33341, #22260, #20577, .T. ) ;
#9161=AXIS2_PLACEMENT_3D ( 'NONE', #36957, #381, #9526 ) ;
#9166=VERTEX_POINT ( 'NONE', #5128 ) ;
#9167=CARTESIAN_POINT ( 'NONE',  ( 9.356056665764066693, 26.06569820189703179, 10.50000000000000000 ) ) ;
#9169=DIRECTION ( 'NONE',  ( 0.000000000000000000, -0.6445931928399465383, 0.7645257456386955752 ) ) ;
#9170=DIRECTION ( 'NONE',  ( 0.000000000000000000, 0.000000000000000000, -1.000000000000000000 ) ) ;
#9173=FACE_OUTER_BOUND ( 'NONE', #5151, .T. ) ;
#9176=CARTESIAN_POINT ( 'NONE',  ( 14.97009266215792778, 21.42933399866928568, 10.49999999999999822 ) ) ;
#9177=LINE ( 'NONE', #21563, #9926 ) ;
#9179=ADVANCED_FACE ( 'NONE', ( #17535 ), #29909, .T. ) ;
#9185=CARTESIAN_POINT ( 'NONE',  ( -13.94482798346716557, 26.50521816028930289, 11.00000000000000000 ) ) ;
#9186=ORIENTED_EDGE ( 'NONE', *, *, #19305, .T. ) ;
#9187=ORIENTED_EDGE ( 'NONE', *, *, #2099, .F. ) ;
#9190=CARTESIAN_POINT ( 'NONE',  ( 13.97557076678965693, 21.53386246193694475, 7.500000000000010658 ) ) ;
#9191=ORIENTED_EDGE ( 'NONE', *, *, #21052, .T. ) ;
#9194=CARTESIAN_POINT ( 'NONE',  ( -12.80736835487442349, 15.68301270189233954, 7.499999999999993783 ) ) ;
#9195=ORIENTED_EDGE ( 'NONE', *, *, #39045, .F. ) ;
#9197=CARTESIAN_POINT ( 'NONE',  ( -7.014595103779441843, 35.79644522156330311, 10.50000000000000355 ) ) ;
#9199=B_SPLINE_CURVE_WITH_KNOTS ( 'NONE', 3,
 ( #38809, #7519, #29665, #25811, #35564, #29062 ),
 .UNSPECIFIED., .F., .F.,
 ( 4, 2, 4 ),
 ( 0.000000000000000000, 0.5000000000000000000, 1.000000000000000000 ),
 .UNSPECIFIED. ) ;
#9200=B_SPLINE_CURVE_WITH_KNOTS ( 'NONE', 3,
 ( #38497, #1530, #16364, #10673, #10466, #20019 ),
 .UNSPECIFIED., .F., .F.,
 ( 4, 2, 4 ),
 ( 0.000000000000000000, 0.5000000000000000000, 1.000000000000000000 ),
 .UNSPECIFIED. ) ;
#9201=ORIENTED_EDGE ( 'NONE', *, *, #39040, .T. ) ;
#9203=VERTEX_POINT ( 'NONE', #40043 ) ;
#9205=VECTOR ( 'NONE', #9918, 1000.000000000000227 ) ;
#9209=VERTEX_POINT ( 'NONE', #27659 ) ;
#9211=FACE_OUTER_BOUND ( 'NONE', #15019, .T. ) ;
#9212=CARTESIAN_POINT ( 'NONE',  ( 13.24038105676655164, 15.43301270189216368, 11.00000000000000000 ) ) ;
#9213=CARTESIAN_POINT ( 'NONE',  ( -6.354454053420243831, 35.54304081427989814, 7.000000000000000000 ) ) ;
#9214=AXIS2_PLACEMENT_3D ( 'NONE', #2759, #33260, #26946 ) ;
#9215=CARTESIAN_POINT ( 'NONE',  ( 13.05736835487433467, 16.11602540378438420, 11.00000000000000000 ) ) ;
#9220=CARTESIAN_POINT ( 'NONE',  ( 15.02235689379175732, 21.92659494635341844, 11.00000000000000000 ) ) ;
#9223=CARTESIAN_POINT ( 'NONE',  ( 5.473344025737212348, 14.11593743010426572, 10.49999999999999822 ) ) ;
#9225=ORIENTED_EDGE ( 'NONE', *, *, #27995, .F. ) ;
#9232=ORIENTED_EDGE ( 'NONE', *, *, #31119, .T. ) ;
#9234=ORIENTED_EDGE ( 'NONE', *, *, #29646, .F. ) ;
#9238=DIRECTION ( 'NONE',  ( -0.9135454576426046414, -0.4067366430757919371, 0.000000000000000000 ) ) ;
#9241=CARTESIAN_POINT ( 'NONE',  ( 14.31603901957230462, 19.98981538725069740, 11.00000000000000000 ) ) ;
#9243=ADVANCED_FACE ( 'NONE', ( #24412 ), #8977, .T. ) ;
#9244=VERTEX_POINT ( 'NONE', #9176 ) ;
#9246=CARTESIAN_POINT ( 'NONE',  ( 10.10646936306337729, 32.94553861768082470, 7.000000000000000000 ) ) ;
#9248=DIRECTION ( 'NONE',  ( 0.9510565162951504226, -0.3090169943749573322, 0.000000000000000000 ) ) ;
#9251=ORIENTED_EDGE ( 'NONE', *, *, #24548, .F. ) ;
#9254=CIRCLE ( 'NONE', #37144, 6.000000000000014211 ) ;
#9257=ORIENTED_EDGE ( 'NONE', *, *, #7539, .F. ) ;
#9259=DIRECTION ( 'NONE',  ( -1.000000000000000000, 0.000000000000000000, 0.000000000000000000 ) ) ;
#9260=EDGE_LOOP ( 'NONE', ( #1441, #6565, #16317, #17399 ) ) ;
#9261=EDGE_CURVE ( 'NONE', #1897, #4338, #15669, .T. ) ;
#9265=DIRECTION ( 'NONE',  ( -0.000000000000000000, -0.000000000000000000, 1.000000000000000000 ) ) ;
#9266=CARTESIAN_POINT ( 'NONE',  ( 13.99633081586303796, 26.34670874090659609, 10.83333333333333215 ) ) ;
#9268=CARTESIAN_POINT ( 'NONE',  ( -13.58430815669637859, 27.61478409596699279, 10.83333333333333570 ) ) ;
#9269=CARTESIAN_POINT ( 'NONE',  ( 13.22516817658079802, 40.70288237343621063, 7.000000000000000000 ) ) ;
#9270=AXIS2_PLACEMENT_3D ( 'NONE', #7170, #22612, #10429 ) ;
#9272=DIRECTION ( 'NONE',  ( 1.224646799147351235E-16, -1.000000000000000000, -0.000000000000000000 ) ) ;
#9273=CARTESIAN_POINT ( 'NONE',  ( 7.096882951594525757, 29.56287847632727050, 10.50000000000000000 ) ) ;
#9276=DIRECTION ( 'NONE',  ( -0.8660254037844432595, -0.4999999999999920064, 0.000000000000000000 ) ) ;
#9277=ORIENTED_EDGE ( 'NONE', *, *, #30760, .F. ) ;
#9278=AXIS2_PLACEMENT_3D ( 'NONE', #898, #4545, #13480 ) ;
#9281=CARTESIAN_POINT ( 'NONE',  ( 11.44473057578109199, 31.45924896672603310, 10.50000000000000178 ) ) ;
#9286=ORIENTED_EDGE ( 'NONE', *, *, #6931, .T. ) ;
#9288=EDGE_CURVE ( 'NONE', #19542, #8554, #6584, .T. ) ;
#9290=CONICAL_SURFACE ( 'NONE', #13830, 1.000000000000011324, 0.7853981633974549403 ) ;
#9297=LINE ( 'NONE', #19229, #34841 ) ;
#9300=AXIS2_PLACEMENT_3D ( 'NONE', #11908, #30200, #24491 ) ;
#9303=AXIS2_PLACEMENT_3D ( 'NONE', #25547, #28004, #19656 ) ;
#9306=DIRECTION ( 'NONE',  ( 0.9945218953682742891, 0.1045284632676437425, -0.000000000000000000 ) ) ;
#9312=EDGE_CURVE ( 'NONE', #31096, #31127, #27387, .T. ) ;
#9313=CARTESIAN_POINT ( 'NONE',  ( -8.633502029282189127, 11.46765470489704342, 10.00000000000000000 ) ) ;
#9314=VERTEX_POINT ( 'NONE', #18919 ) ;
#9315=EDGE_CURVE ( 'NONE', #19145, #23249, #15068, .T. ) ;
#9316=CARTESIAN_POINT ( 'NONE',  ( 0.7500000000000004441, 33.00000000000000000, 10.75000000000000000 ) ) ;
#9319=PLANE ( 'NONE',  #31147 ) ;
#9323=FACE_OUTER_BOUND ( 'NONE', #3407, .T. ) ;
#9325=CARTESIAN_POINT ( 'NONE',  ( 0.000000000000000000, 22.50000000000000355, 7.000000000000000000 ) ) ;
#9328=AXIS2_PLACEMENT_3D ( 'NONE', #12518, #37700, #31205 ) ;
#9337=ADVANCED_FACE ( 'NONE', ( #3078 ), #2862, .T. ) ;
#9338=DIRECTION ( 'NONE',  ( 0.1045284632676569680, 0.9945218953682729568, -0.000000000000000000 ) ) ;
#9342=CARTESIAN_POINT ( 'NONE',  ( 11.46110508464496824, 32.14680900553369014, 10.68306113187827933 ) ) ;
#9343=ORIENTED_EDGE ( 'NONE', *, *, #12440, .F. ) ;
#9345=CARTESIAN_POINT ( 'NONE',  ( 0.5000000000000000000, 37.18846563620834189, 10.96580507645519909 ) ) ;
#9347=CONICAL_SURFACE ( 'NONE', #14538, 1.000000000000004441, 0.7853981633974522758 ) ;
#9348=CARTESIAN_POINT ( 'NONE',  ( 0.6108529249775871417, 37.48755679569043053, 7.500000000000000888 ) ) ;
#9349=ORIENTED_EDGE ( 'NONE', *, *, #16852, .F. ) ;
#9352=DIRECTION ( 'NONE',  ( 0.000000000000000000, 0.000000000000000000, -1.000000000000000000 ) ) ;
#9353=B_SPLINE_SURFACE_WITH_KNOTS ( 'NONE', 1, 3, ( 
 ( #15037, #3046, #30490, #11795, #6089, #30288, #27430, #33932, #24585, #37175 ),
 ( #5691, #18102, #21727, #24777, #34135, #40012, #24181, #17904, #6286, #18296 ) ),
 .UNSPECIFIED., .F., .F., .F.,
 ( 2, 2 ),
 ( 4, 2, 2, 2, 4 ),
 ( 0.000000000000000000, 1.000000000000000000 ),
 ( -1.096214744126235097, -0.7035156624275106241, -0.3108165807287861515, 0.08188250096993832106, 0.4745815826686627936 ),
 .UNSPECIFIED. ) ;
#9354=EDGE_LOOP ( 'NONE', ( #9915, #39060, #34537 ) ) ;
#9356=CYLINDRICAL_SURFACE ( 'NONE', #30008, 6.000000000000001776 ) ;
#9357=VERTEX_POINT ( 'NONE', #31307 ) ;
#9360=ORIENTED_EDGE ( 'NONE', *, *, #30488, .T. ) ;
#9361=LINE ( 'NONE', #12576, #10307 ) ;
#9364=CARTESIAN_POINT ( 'NONE',  ( 1.204925152852602155, 12.02153850147726999, 11.00000000000000000 ) ) ;
#9365=LINE ( 'NONE', #31100, #33209 ) ;
#9366=ADVANCED_FACE ( 'NONE', ( #19511 ), #27860, .F. ) ;
#9368=CIRCLE ( 'NONE', #6735, 6.000000000000003553 ) ;
#9371=CARTESIAN_POINT ( 'NONE',  ( 3.574287532905564557, 8.089166425130672522, 10.87262190629281022 ) ) ;
#9373=CARTESIAN_POINT ( 'NONE',  ( 12.63210941633768947, 14.41074797273250496, 7.485699520496975623 ) ) ;
#9377=CARTESIAN_POINT ( 'NONE',  ( -12.67493120981686516, 14.45362483784325924, 10.49999999999999822 ) ) ;
#9378=ADVANCED_FACE ( 'NONE', ( #9777 ), #29061, .F. ) ;
#9380=ORIENTED_EDGE ( 'NONE', *, *, #34744, .T. ) ;
#9384=EDGE_CURVE ( 'NONE', #33679, #31336, #17819, .T. ) ;
#9385=CARTESIAN_POINT ( 'NONE',  ( 3.503793317224329851, 8.420815634768676006, 7.499999999999990230 ) ) ;
#9386=ORIENTED_EDGE ( 'NONE', *, *, #13443, .T. ) ;
#9392=CIRCLE ( 'NONE', #32096, 15.00000000000000000 ) ;
#9393=EDGE_LOOP ( 'NONE', ( #7135, #3014, #33637, #34960 ) ) ;
#9394=ADVANCED_FACE ( 'NONE', ( #22960 ), #25602, .T. ) ;
#9397=CARTESIAN_POINT ( 'NONE',  ( -3.503793317224518145, 8.420815634768723967, 7.000000000000000000 ) ) ;
#9398=EDGE_LOOP ( 'NONE', ( #38012, #13522, #30840, #28037 ) ) ;
#9402=ORIENTED_EDGE ( 'NONE', *, *, #3945, .F. ) ;
#9408=ORIENTED_EDGE ( 'NONE', *, *, #34109, .T. ) ;
#9411=CARTESIAN_POINT ( 'NONE',  ( -14.52537758579311067, 26.24401664712872062, 7.365694256298322529 ) ) ;
#9415=CARTESIAN_POINT ( 'NONE',  ( 13.16028273094469014, 27.30176617939681449, 7.500000000000000888 ) ) ;
#9417=AXIS2_PLACEMENT_3D ( 'NONE', #5708, #5311, #18118 ) ;
#9419=VECTOR ( 'NONE', #2744, 1000.000000000000000 ) ;
#9420=DIRECTION ( 'NONE',  ( 1.000000000000000000, 0.000000000000000000, 0.000000000000000000 ) ) ;
#9423=DIRECTION ( 'NONE',  ( -0.2876062384759393020, -0.6459741880212640508, -0.7071067811865402453 ) ) ;
#9427=EDGE_CURVE ( 'NONE', #15350, #19729, #31904, .T. ) ;
#9429=EDGE_LOOP ( 'NONE', ( #37713, #27908, #5387, #15996 ) ) ;
#9432=EDGE_CURVE ( 'NONE', #253, #17719, #24316, .T. ) ;
#9433=DIRECTION ( 'NONE',  ( -0.000000000000000000, -0.000000000000000000, -1.000000000000000000 ) ) ;
#9435=EDGE_LOOP ( 'NONE', ( #19856, #15033, #34938, #24783, #141 ) ) ;
#9437=EDGE_LOOP ( 'NONE', ( #3959, #8838, #21772, #13764 ) ) ;
#9439=CARTESIAN_POINT ( 'NONE',  ( -12.83926296998453154, 26.67172942406192604, 7.000000000000000000 ) ) ;
#9441=CARTESIAN_POINT ( 'NONE',  ( 12.74038105676659249, 14.56698729810780613, 10.59344459855566889 ) ) ;
#9442=AXIS2_PLACEMENT_3D ( 'NONE', #23779, #32937, #20749 ) ;
#9443=ORIENTED_EDGE ( 'NONE', *, *, #34083, .F. ) ;
#9446=DIRECTION ( 'NONE',  ( 0.000000000000000000, 0.000000000000000000, 1.000000000000000000 ) ) ;
#9448=ORIENTED_EDGE ( 'NONE', *, *, #8046, .T. ) ;
#9451=DIRECTION ( 'NONE',  ( -1.000000000000000000, 0.000000000000000000, 0.000000000000000000 ) ) ;
#9454=ORIENTED_EDGE ( 'NONE', *, *, #35662, .T. ) ;
#9457=CIRCLE ( 'NONE', #35401, 0.4999999999999997780 ) ;
#9458=AXIS2_PLACEMENT_3D ( 'NONE', #21135, #11398, #30489 ) ;
#9459=CARTESIAN_POINT ( 'NONE',  ( -5.537830610278340338, 36.16746786612513631, 10.94387467463486452 ) ) ;
#9464=ORIENTED_EDGE ( 'NONE', *, *, #5871, .F. ) ;
#9465=EDGE_CURVE ( 'NONE', #20052, #31246, #11990, .T. ) ;
#9470=DIRECTION ( 'NONE',  ( -1.000000000000000000, 0.000000000000000000, 0.000000000000000000 ) ) ;
#9471=CARTESIAN_POINT ( 'NONE',  ( 1.278175571583998860, 14.08178954835375940, 9.000000000000001776 ) ) ;
#9473=AXIS2_PLACEMENT_3D ( 'NONE', #25448, #7365, #31554 ) ;
#9475=DIRECTION ( 'NONE',  ( -0.2185080122244101586, -0.6724985119639573794, -0.7071067811865475727 ) ) ;
#9478=CARTESIAN_POINT ( 'NONE',  ( -6.789317288263781336, 35.87572455244716707, 7.455686640544902488 ) ) ;
#9479=AXIS2_PLACEMENT_3D ( 'NONE', #1995, #20683, #1787 ) ;
#9480=ORIENTED_EDGE ( 'NONE', *, *, #10443, .T. ) ;
#9484=FACE_OUTER_BOUND ( 'NONE', #11024, .T. ) ;
#9485=AXIS2_PLACEMENT_3D ( 'NONE', #19876, #14378, #4632 ) ;
#9490=ORIENTED_EDGE ( 'NONE', *, *, #29513, .T. ) ;
#9492=B_SPLINE_CURVE_WITH_KNOTS ( 'NONE', 3,
 ( #23395, #11609, #32749, #2068, #8149, #14444 ),
 .UNSPECIFIED., .F., .F.,
 ( 4, 2, 4 ),
 ( 0.000000000000000000, 0.5000000000000000000, 1.000000000000000000 ),
 .UNSPECIFIED. ) ;
#9500=EDGE_CURVE ( 'NONE', #1586, #11592, #16270, .T. ) ;
#9501=ORIENTED_EDGE ( 'NONE', *, *, #37681, .F. ) ;
#9504=EDGE_LOOP ( 'NONE', ( #12246, #23818, #22175 ) ) ;
#9505=DIRECTION ( 'NONE',  ( 0.000000000000000000, 0.000000000000000000, 1.000000000000000000 ) ) ;
#9506=CARTESIAN_POINT ( 'NONE',  ( 10.73859285986296541, 31.49625607628530588, 10.00000000000000000 ) ) ;
#9510=AXIS2_PLACEMENT_3D ( 'NONE', #9439, #30971, #21818 ) ;
#9511=VECTOR ( 'NONE', #32585, 1000.000000000000114 ) ;
#9512=EDGE_CURVE ( 'NONE', #30503, #6957, #32319, .T. ) ;
#9513=ORIENTED_EDGE ( 'NONE', *, *, #28950, .T. ) ;
#9515=EDGE_LOOP ( 'NONE', ( #25770, #8440, #23741, #22359 ) ) ;
#9516=CARTESIAN_POINT ( 'NONE',  ( -14.47283171447380035, 21.48159823030330884, 9.000000000000001776 ) ) ;
#9517=DIRECTION ( 'NONE',  ( 0.000000000000000000, 0.000000000000000000, -1.000000000000000000 ) ) ;
#9519=DIRECTION ( 'NONE',  ( 0.9510565162951543083, 0.3090169943749450088, 0.000000000000000000 ) ) ;
#9520=ORIENTED_EDGE ( 'NONE', *, *, #16972, .F. ) ;
#9521=ADVANCED_FACE ( 'NONE', ( #39402 ), #35767, .T. ) ;
#9523=CARTESIAN_POINT ( 'NONE',  ( 3.295881626406581777, 9.398963235502485247, 9.500000000000000000 ) ) ;
#9524=DIRECTION ( 'NONE',  ( -0.9135454576426059736, -0.4067366430757888285, -0.000000000000000000 ) ) ;
#9526=DIRECTION ( 'NONE',  ( -1.000000000000000000, 0.000000000000000000, 0.000000000000000000 ) ) ;
#9527=CARTESIAN_POINT ( 'NONE',  ( 13.63581098909226874, 27.45627467658428955, 7.000000000000000000 ) ) ;
#9530=ORIENTED_EDGE ( 'NONE', *, *, #20537, .F. ) ;
#9534=LINE ( 'NONE', #15227, #15874 ) ;
#9545=LINE ( 'NONE', #6281, #7934 ) ;
#9546=ADVANCED_FACE ( 'NONE', ( #2045 ), #13250, .T. ) ;
#9547=EDGE_LOOP ( 'NONE', ( #17102, #26780, #22670 ) ) ;
#9550=CARTESIAN_POINT ( 'NONE',  ( 9.997483185316555776, 21.95197631500757041, 10.50000000000000355 ) ) ;
#9552=ORIENTED_EDGE ( 'NONE', *, *, #31848, .T. ) ;
#9558=CARTESIAN_POINT ( 'NONE',  ( 2.421689871081641687, 8.701977744317826335, 7.499999999999991118 ) ) ;
#9559=ORIENTED_EDGE ( 'NONE', *, *, #16715, .T. ) ;
#9561=ORIENTED_EDGE ( 'NONE', *, *, #8273, .T. ) ;
#9563=DIRECTION ( 'NONE',  ( -0.9781476007338069101, -0.2079116908177532919, 0.000000000000000000 ) ) ;
#9564=CARTESIAN_POINT ( 'NONE',  ( -11.54666566735211752, 32.07468077621347646, 7.500000000000004441 ) ) ;
#9572=CARTESIAN_POINT ( 'NONE',  ( 0.5000000000000001110, 37.00000000000000711, 9.000000000000001776 ) ) ;
#9574=FACE_OUTER_BOUND ( 'NONE', #26180, .T. ) ;
#9576=AXIS2_PLACEMENT_3D ( 'NONE', #4367, #7614, #29157 ) ;
#9580=DIRECTION ( 'NONE',  ( -0.9945218953682742891, -0.1045284632676437425, 0.000000000000000000 ) ) ;
#9581=VERTEX_POINT ( 'NONE', #8531 ) ;
#9586=ADVANCED_FACE ( 'NONE', ( #14631 ), #8122, .F. ) ;
#9593=CIRCLE ( 'NONE', #18045, 0.5000000000000004441 ) ;
#9597=CARTESIAN_POINT ( 'NONE',  ( 5.644276917315719899, 36.40655018617690786, 11.00000000000000000 ) ) ;
#9598=EDGE_LOOP ( 'NONE', ( #29349, #20623, #12877, #10726 ) ) ;
#9600=DIRECTION ( 'NONE',  ( 0.000000000000000000, 0.000000000000000000, 1.000000000000000000 ) ) ;
#9601=CARTESIAN_POINT ( 'NONE',  ( -12.05736835487443415, 14.38397459621567442, 11.00000000000000000 ) ) ;
#9603=EDGE_LOOP ( 'NONE', ( #1246, #6791, #17794, #38599, #24819, #21333 ) ) ;
#9605=VERTEX_POINT ( 'NONE', #33332 ) ;
#9610=EDGE_LOOP ( 'NONE', ( #18549, #35645, #34311, #33005, #23421, #29085 ) ) ;
#9615=FACE_OUTER_BOUND ( 'NONE', #4614, .T. ) ;
#9616=EDGE_CURVE ( 'NONE', #5670, #38335, #1616, .T. ) ;
#9617=EDGE_CURVE ( 'NONE', #20501, #38258, #35339, .T. ) ;
#9619=CIRCLE ( 'NONE', #20658, 1.000000000000002665 ) ;
#9620=AXIS2_PLACEMENT_3D ( 'NONE', #37230, #31326, #6335 ) ;
#9625=CARTESIAN_POINT ( 'NONE',  ( 7.111215932167701759, 17.81698729810774751, 7.000000000000000000 ) ) ;
#9626=CARTESIAN_POINT ( 'NONE',  ( 7.611215932167711529, 18.68301270189218855, 9.000000000000001776 ) ) ;
#9628=LINE ( 'NONE', #9223, #870 ) ;
#9630=AXIS2_PLACEMENT_3D ( 'NONE', #21930, #6092, #15441 ) ;
#9634=DIRECTION ( 'NONE',  ( 0.000000000000000000, 0.000000000000000000, -1.000000000000000000 ) ) ;
#9636=ORIENTED_EDGE ( 'NONE', *, *, #14389, .T. ) ;
#9637=CARTESIAN_POINT ( 'NONE',  ( -3.357189294653177836, 32.49896394832315849, 11.00000000000000000 ) ) ;
#9641=DIRECTION ( 'NONE',  ( -0.1045284632676569680, -0.9945218953682730678, 0.000000000000000000 ) ) ;
#9644=CARTESIAN_POINT ( 'NONE',  ( 12.29179778625991304, 14.31343464431668799, 10.49999999999999822 ) ) ;
#9646=ORIENTED_EDGE ( 'NONE', *, *, #28865, .F. ) ;
#9649=DIRECTION ( 'NONE',  ( 0.000000000000000000, 1.000000000000000000, 0.000000000000000000 ) ) ;
#9651=ORIENTED_EDGE ( 'NONE', *, *, #1227, .F. ) ;
#9653=CARTESIAN_POINT ( 'NONE',  ( -0.5000000000000004441, 37.00000000000000711, 9.000000000000001776 ) ) ;
#9656=B_SPLINE_CURVE_WITH_KNOTS ( 'NONE', 3,
 ( #25325, #12734, #15590, #6041, #3392, #6828 ),
 .UNSPECIFIED., .F., .F.,
 ( 4, 2, 4 ),
 ( 0.000000000000000000, 0.5000000000000000000, 1.000000000000000000 ),
 .UNSPECIFIED. ) ;
#9659=AXIS2_PLACEMENT_3D ( 'NONE', #12970, #16026, #31666 ) ;
#9664=VECTOR ( 'NONE', #14258, 1000.000000000000000 ) ;
#9666=ADVANCED_FACE ( 'NONE', ( #15424 ), #23653, .T. ) ;
#9667=DIRECTION ( 'NONE',  ( 1.000000000000000000, 0.000000000000000000, 0.000000000000000000 ) ) ;
#9668=ADVANCED_FACE ( 'NONE', ( #31069 ), #15024, .F. ) ;
#9669=ORIENTED_EDGE ( 'NONE', *, *, #24746, .F. ) ;
#9670=FACE_OUTER_BOUND ( 'NONE', #8000, .T. ) ;
#9671=DIRECTION ( 'NONE',  ( -1.000000000000000000, 0.000000000000000000, 0.000000000000000000 ) ) ;
#9674=CARTESIAN_POINT ( 'NONE',  ( 14.91650131011209268, 21.43496667674292055, 10.76099332938163577 ) ) ;
#9675=CARTESIAN_POINT ( 'NONE',  ( 14.86556419889023672, 20.43481210330075726, 10.59344459855564935 ) ) ;
#9677=DIRECTION ( 'NONE',  ( -0.000000000000000000, -0.000000000000000000, -1.000000000000000000 ) ) ;
#9678=CARTESIAN_POINT ( 'NONE',  ( -7.929471891321301591, 25.60217271033470610, 9.000000000000001776 ) ) ;
#9680=VECTOR ( 'NONE', #14470, 1000.000000000000000 ) ;
#9683=AXIS2_PLACEMENT_3D ( 'NONE', #11336, #7872, #21077 ) ;
#9686=CARTESIAN_POINT ( 'NONE',  ( 5.362728154695970417, 13.41753630677055753, 10.50000000000000000 ) ) ;
#9692=VECTOR ( 'NONE', #30053, 1000.000000000000114 ) ;
#9693=B_SPLINE_SURFACE_WITH_KNOTS ( 'NONE', 1, 3, ( 
 ( #20629, #17184, #23267, #23666, #35661, #7819, #20828, #32823, #20222, #23865 ),
 ( #29559, #1738, #14520, #26913, #4978, #17390, #29764, #5375, #36268, #8431 ) ),
 .UNSPECIFIED., .F., .F., .F.,
 ( 2, 2 ),
 ( 4, 2, 2, 2, 4 ),
 ( 0.000000000000000000, 1.000000000000000000 ),
 ( -1.496612791730154157, -1.103913710031430906, -0.7112146283327074325, -0.3185155466339841257, 0.07418353506473918113 ),
 .UNSPECIFIED. ) ;
#9694=EDGE_LOOP ( 'NONE', ( #25430, #23181, #15380, #11571 ) ) ;
#9695=CARTESIAN_POINT ( 'NONE',  ( -8.118377661053489902, 10.47536095541709322, 9.000000000000001776 ) ) ;
#9701=VERTEX_POINT ( 'NONE', #28011 ) ;
#9704=VERTEX_POINT ( 'NONE', #18480 ) ;
#9708=LINE ( 'NONE', #22088, #33663 ) ;
#9709=CARTESIAN_POINT ( 'NONE',  ( 3.399837471815457590, 8.909889435135580626, 7.499999999999990230 ) ) ;
#9714=EDGE_LOOP ( 'NONE', ( #24557, #30762, #16743, #6004 ) ) ;
#9715=DIRECTION ( 'NONE',  ( 0.6691306063588569053, -0.7431448254773954654, 0.000000000000000000 ) ) ;
#9719=DIRECTION ( 'NONE',  ( 0.4999999999999912292, -0.8660254037844437036, 0.000000000000000000 ) ) ;
#9720=VERTEX_POINT ( 'NONE', #15625 ) ;
#9723=LINE ( 'NONE', #22104, #37095 ) ;
#9726=CARTESIAN_POINT ( 'NONE',  ( -10.44103466624267540, 32.57396620494226624, 11.00000000000000000 ) ) ;
#9732=DIRECTION ( 'NONE',  ( 0.8090169943749504489, 0.5877852522924690293, 0.000000000000000000 ) ) ;
#9740=EDGE_CURVE ( 'NONE', #13272, #39672, #184, .T. ) ;
#9741=CARTESIAN_POINT ( 'NONE',  ( 13.81505241748941515, 27.51451374705149888, 10.96580508970281542 ) ) ;
#9742=CARTESIAN_POINT ( 'NONE',  ( -14.70623423376111738, 19.54590544129804286, 7.000000000000000000 ) ) ;
#9743=EDGE_LOOP ( 'NONE', ( #14601, #38030, #16125 ) ) ;
#9744=AXIS2_PLACEMENT_3D ( 'NONE', #22047, #6403, #9671 ) ;
#9746=CARTESIAN_POINT ( 'NONE',  ( 10.03245514394483706, 31.53326318584457510, 7.000000000000000000 ) ) ;
#9748=VERTEX_POINT ( 'NONE', #27817 ) ;
#9751=CARTESIAN_POINT ( 'NONE',  ( 14.53551886312849994, 26.20443074943802841, 7.338691926023212631 ) ) ;
#9753=EDGE_CURVE ( 'NONE', #39323, #14045, #16515, .T. ) ;
#9763=CARTESIAN_POINT ( 'NONE',  ( 12.30736835487432757, 14.81698729810772441, 9.500000000000000000 ) ) ;
#9765=CYLINDRICAL_SURFACE ( 'NONE', #24614, 0.5000000000000004441 ) ;
#9766=ORIENTED_EDGE ( 'NONE', *, *, #15111, .F. ) ;
#9767=CARTESIAN_POINT ( 'NONE',  ( 3.900351417861458003, 8.105760029628141794, 10.49999999999999822 ) ) ;
#9769=EDGE_CURVE ( 'NONE', #7636, #37730, #9534, .T. ) ;
#9772=AXIS2_PLACEMENT_3D ( 'NONE', #2179, #14563, #26955 ) ;
#9777=FACE_OUTER_BOUND ( 'NONE', #35539, .T. ) ;
#9778=LINE ( 'NONE', #37613, #512 ) ;
#9779=ORIENTED_EDGE ( 'NONE', *, *, #23736, .T. ) ;
#9785=LINE ( 'NONE', #28463, #36074 ) ;
#9786=ORIENTED_EDGE ( 'NONE', *, *, #34397, .F. ) ;
#9789=FACE_OUTER_BOUND ( 'NONE', #14905, .T. ) ;
#9790=EDGE_CURVE ( 'NONE', #8575, #24087, #37160, .T. ) ;
#9794=FACE_OUTER_BOUND ( 'NONE', #33540, .T. ) ;
#9795=ORIENTED_EDGE ( 'NONE', *, *, #35085, .T. ) ;
#9799=AXIS2_PLACEMENT_3D ( 'NONE', #1230, #10170, #29654 ) ;
#9806=ORIENTED_EDGE ( 'NONE', *, *, #11747, .F. ) ;
#9807=B_SPLINE_CURVE_WITH_KNOTS ( 'NONE', 3,
 ( #14079, #13678, #26066, #26477, #38466, #10639, #23022, #38873 ),
 .UNSPECIFIED., .F., .F.,
 ( 4, 2, 2, 4 ),
 ( 0.000000000000000000, 0.0004726692273637142245, 0.0007090038410455722041, 0.0009453384547274302921 ),
 .UNSPECIFIED. ) ;
#9810=VECTOR ( 'NONE', #14666, 1000.000000000000000 ) ;
#9811=PLANE ( 'NONE',  #40158 ) ;
#9812=VECTOR ( 'NONE', #3061, 1000.000000000000114 ) ;
#9813=EDGE_CURVE ( 'NONE', #26679, #33392, #2882, .T. ) ;
#9822=EDGE_LOOP ( 'NONE', ( #20590, #1411, #37169 ) ) ;
#9825=CARTESIAN_POINT ( 'NONE',  ( 10.10646936306337906, 32.94553861768082470, 10.49999999999999822 ) ) ;
#9827=ORIENTED_EDGE ( 'NONE', *, *, #5642, .T. ) ;
#9828=FACE_OUTER_BOUND ( 'NONE', #33710, .T. ) ;
#9829=ORIENTED_EDGE ( 'NONE', *, *, #19717, .T. ) ;
#9834=DIRECTION ( 'NONE',  ( 0.000000000000000000, -0.000000000000000000, -1.000000000000000000 ) ) ;
#9840=ORIENTED_EDGE ( 'NONE', *, *, #33524, .F. ) ;
#9843=FACE_OUTER_BOUND ( 'NONE', #4588, .T. ) ;
#9844=EDGE_CURVE ( 'NONE', #35248, #4321, #14575, .T. ) ;
#9845=CARTESIAN_POINT ( 'NONE',  ( 9.427394655428274817, 11.06314620770945290, 11.00000000000000000 ) ) ;
#9846=DIRECTION ( 'NONE',  ( -0.1045284632676569680, -0.9945218953682729568, 0.000000000000000000 ) ) ;
#9851=ORIENTED_EDGE ( 'NONE', *, *, #26135, .T. ) ;
#9852=AXIS2_PLACEMENT_3D ( 'NONE', #21341, #36777, #8544 ) ;
#9854=CARTESIAN_POINT ( 'NONE',  ( 6.354454053420411697, 35.54304081427980577, 7.500000000000000888 ) ) ;
#9857=EDGE_CURVE ( 'NONE', #14734, #2755, #27613, .T. ) ;
#9859=CARTESIAN_POINT ( 'NONE',  ( -1.000000000000000000, 37.50000000000000711, 10.50000000000000178 ) ) ;
#9863=CARTESIAN_POINT ( 'NONE',  ( 14.36203778474857806, 19.98498072221368815, 10.49999999999999822 ) ) ;
#9865=DIRECTION ( 'NONE',  ( 0.000000000000000000, 0.000000000000000000, 1.000000000000000000 ) ) ;
#9866=FACE_OUTER_BOUND ( 'NONE', #17960, .T. ) ;
#9869=ORIENTED_EDGE ( 'NONE', *, *, #8268, .F. ) ;
#9871=CARTESIAN_POINT ( 'NONE',  ( 2.629601561899429285, 7.723830143584023311, 10.59344459855566889 ) ) ;
#9875=CARTESIAN_POINT ( 'NONE',  ( -5.982165713378357452, 28.55918256678905465, 9.000000000000001776 ) ) ;
#9877=ORIENTED_EDGE ( 'NONE', *, *, #10314, .T. ) ;
#9888=ORIENTED_EDGE ( 'NONE', *, *, #17590, .T. ) ;
#9889=EDGE_CURVE ( 'NONE', #27233, #35146, #21326, .T. ) ;
#9891=CARTESIAN_POINT ( 'NONE',  ( 9.038010526469520300, 11.76154733104316819, 9.500000000000000000 ) ) ;
#9893=ORIENTED_EDGE ( 'NONE', *, *, #23942, .T. ) ;
#9895=ADVANCED_FACE ( 'NONE', ( #16423 ), #3548, .T. ) ;
#9897=VECTOR ( 'NONE', #30571, 1000.000000000000000 ) ;
#9898=VERTEX_POINT ( 'NONE', #10326 ) ;
#9899=CARTESIAN_POINT ( 'NONE',  ( 1.838889047819958655, 31.15129278236397781, 9.000000000000001776 ) ) ;
#9901=B_SPLINE_CURVE_WITH_KNOTS ( 'NONE', 3,
 ( #38445, #32762, #11221, #11025, #23611, #19962, #22795, #22997 ),
 .UNSPECIFIED., .F., .F.,
 ( 4, 2, 2, 4 ),
 ( 0.000000000000000000, 0.0004726692273637109177, 0.0007090038410455688431, 0.0009453384547274268227 ),
 .UNSPECIFIED. ) ;
#9907=CIRCLE ( 'NONE', #1471, 15.00000000000000000 ) ;
#9909=DIRECTION ( 'NONE',  ( -0.3535533905932713994, 0.6123724356958013537, -0.7071067811865427988 ) ) ;
#9910=DIRECTION ( 'NONE',  ( 0.000000000000000000, 0.000000000000000000, 1.000000000000000000 ) ) ;
#9912=ADVANCED_FACE ( 'NONE', ( #15823 ), #12967, .F. ) ;
#9914=DIRECTION ( 'NONE',  ( 0.000000000000000000, 0.000000000000000000, 1.000000000000000000 ) ) ;
#9915=ORIENTED_EDGE ( 'NONE', *, *, #11064, .T. ) ;
#9917=CARTESIAN_POINT ( 'NONE',  ( 8.412270287199559604, 10.07085245822950981, 10.49999999999999822 ) ) ;
#9918=DIRECTION ( 'NONE',  ( 0.2079116908177533474, -0.9781476007338067991, 0.000000000000000000 ) ) ;
#9919=LINE ( 'NONE', #30862, #19533 ) ;
#9923=CARTESIAN_POINT ( 'NONE',  ( 2.143544478356361971, 7.864861742947437229, 10.49999999999999645 ) ) ;
#9926=VECTOR ( 'NONE', #33961, 1000.000000000000227 ) ;
#9929=LINE ( 'NONE', #25557, #15264 ) ;
#9932=DIRECTION ( 'NONE',  ( 0.000000000000000000, 0.000000000000000000, -1.000000000000000000 ) ) ;
#9933=MECHANICAL_DESIGN_GEOMETRIC_PRESENTATION_REPRESENTATION('',(#222),#22915);
#9937=EDGE_CURVE ( 'NONE', #26679, #21646, #988, .T. ) ;
#9939=CARTESIAN_POINT ( 'NONE',  ( 9.331903152615748098, 11.35703883385568780, 11.00000000000000000 ) ) ;
#9940=CARTESIAN_POINT ( 'NONE',  ( -10.49474413300070097, 21.89971208337388120, 10.50000000000000000 ) ) ;
#9943=CARTESIAN_POINT ( 'NONE',  ( 6.354454053420409920, 35.54304081427980577, 9.500000000000000000 ) ) ;
#9944=VERTEX_POINT ( 'NONE', #7066 ) ;
#9951=CIRCLE ( 'NONE', #24849, 0.5000000000000004441 ) ;
#9957=FACE_OUTER_BOUND ( 'NONE', #16339, .T. ) ;
#9962=ORIENTED_EDGE ( 'NONE', *, *, #27023, .F. ) ;
#9963=DIRECTION ( 'NONE',  ( 0.5000000000000038858, 0.8660254037844363761, 0.000000000000000000 ) ) ;
#9965=CARTESIAN_POINT ( 'NONE',  ( 12.74038105676653920, 14.56698729810772619, 10.50000000000000000 ) ) ;
#9966=EDGE_CURVE ( 'NONE', #5508, #35565, #16022, .T. ) ;
#9981=ORIENTED_EDGE ( 'NONE', *, *, #26713, .T. ) ;
#9982=EDGE_LOOP ( 'NONE', ( #21450, #20856, #27677 ) ) ;
#9986=CONICAL_SURFACE ( 'NONE', #19097, 1.000000000000006883, 0.7853981633974547183 ) ;
#9989=VERTEX_POINT ( 'NONE', #19071 ) ;
#9992=CARTESIAN_POINT ( 'NONE',  ( 6.572794801194151049, 16.58182897866491956, 9.000000000000001776 ) ) ;
#9994=ORIENTED_EDGE ( 'NONE', *, *, #23785, .F. ) ;
#9996=ORIENTED_EDGE ( 'NONE', *, *, #22037, .T. ) ;
#9999=DIRECTION ( 'NONE',  ( -0.000000000000000000, -0.000000000000000000, -1.000000000000000000 ) ) ;
#10003=LINE ( 'NONE', #35188, #21495 ) ;
#10005=AXIS2_PLACEMENT_3D ( 'NONE', #26151, #29405, #35507 ) ;
#10006=CARTESIAN_POINT ( 'NONE',  ( -12.74038105676665289, 14.56698729810790027, 7.000000000000000000 ) ) ;
#10007=EDGE_CURVE ( 'NONE', #36443, #11532, #31662, .T. ) ;
#10008=DIRECTION ( 'NONE',  ( 1.000000000000000000, 0.000000000000000000, -0.000000000000000000 ) ) ;
#10009=B_SPLINE_SURFACE_WITH_KNOTS ( 'NONE', 1, 3, ( 
 ( #18686, #31077, #3244, #15635, #19273, #34720, #31672, #34325, #18884, #31274 ),
 ( #22124, #34524, #31472, #20648, #39321, #2360, #13579, #36082, #23127, #33049 ) ),
 .UNSPECIFIED., .F., .F., .F.,
 ( 2, 2 ),
 ( 4, 2, 2, 2, 4 ),
 ( 0.000000000000000000, 1.000000000000000000 ),
 ( 1.265795420569473695, 1.658494502268196502, 2.051193583966919309, 2.443892665665642117, 2.836591747364364924 ),
 .UNSPECIFIED. ) ;
#10010=VECTOR ( 'NONE', #24965, 1000.000000000000000 ) ;
#10015=EDGE_CURVE ( 'NONE', #7168, #27126, #38154, .T. ) ;
#10019=EDGE_LOOP ( 'NONE', ( #35480, #20043, #37666, #26433 ) ) ;
#10020=CIRCLE ( 'NONE', #28205, 0.5000000000000013323 ) ;
#10025=ORIENTED_EDGE ( 'NONE', *, *, #30939, .F. ) ;
#10030=FACE_OUTER_BOUND ( 'NONE', #35411, .T. ) ;
#10036=DIRECTION ( 'NONE',  ( 0.6123724356958029080, 0.3535533905932708998, -0.7071067811865417996 ) ) ;
#10038=VERTEX_POINT ( 'NONE', #22707 ) ;
#10040=CARTESIAN_POINT ( 'NONE',  ( -12.37435565298220119, 15.93301270189233598, 10.00000000000000000 ) ) ;
#10041=EDGE_CURVE ( 'NONE', #11410, #2015, #12769, .T. ) ;
#10043=ADVANCED_FACE ( 'NONE', ( #29013 ), #3627, .F. ) ;
#10044=CARTESIAN_POINT ( 'NONE',  ( -10.79197459925262947, 32.88995393993013749, 10.68306085400104699 ) ) ;
#10045=ORIENTED_EDGE ( 'NONE', *, *, #17021, .T. ) ;
#10047=VECTOR ( 'NONE', #13209, 1000.000000000000227 ) ;
#10050=VERTEX_POINT ( 'NONE', #781 ) ;
#10055=DIRECTION ( 'NONE',  ( 0.6691306063588671194, 0.7431448254773863615, -0.000000000000000000 ) ) ;
#10056=EDGE_CURVE ( 'NONE', #18776, #9701, #13163, .T. ) ;
#10061=ORIENTED_EDGE ( 'NONE', *, *, #4044, .T. ) ;
#10063=CARTESIAN_POINT ( 'NONE',  ( -8.927394655428429360, 11.06314620770957191, 9.500000000000000000 ) ) ;
#10065=CARTESIAN_POINT ( 'NONE',  ( 7.824485034907089798, 10.87986945260445992, 9.500000000000000000 ) ) ;
#10066=DIRECTION ( 'NONE',  ( 0.000000000000000000, 0.000000000000000000, 1.000000000000000000 ) ) ;
#10067=CYLINDRICAL_SURFACE ( 'NONE', #7395, 0.4999999999999983902 ) ;
#10068=AXIS2_PLACEMENT_3D ( 'NONE', #11737, #27174, #15179 ) ;
#10070=DIRECTION ( 'NONE',  ( -0.9510565162951503115, 0.3090169943749573878, -0.000000000000000000 ) ) ;
#10071=ORIENTED_EDGE ( 'NONE', *, *, #4143, .T. ) ;
#10073=CARTESIAN_POINT ( 'NONE',  ( 2.291516524179206815, 7.763791616332271772, 10.49999999999999822 ) ) ;
#10078=VERTEX_POINT ( 'NONE', #1188 ) ;
#10081=CIRCLE ( 'NONE', #28234, 0.5000000000000004441 ) ;
#10082=CARTESIAN_POINT ( 'NONE',  ( 14.44923221060104090, 26.57085556310762087, 10.49999999999999822 ) ) ;
#10085=AXIS2_PLACEMENT_3D ( 'NONE', #25300, #324, #9470 ) ;
#10086=CIRCLE ( 'NONE', #25014, 5.999999999999994671 ) ;
#10090=VERTEX_POINT ( 'NONE', #6862 ) ;
#10094=EDGE_LOOP ( 'NONE', ( #207, #38168, #1233 ) ) ;
#10096=EDGE_CURVE ( 'NONE', #23174, #20519, #6468, .T. ) ;
#10098=ORIENTED_EDGE ( 'NONE', *, *, #13544, .T. ) ;
#10104=VERTEX_POINT ( 'NONE', #25356 ) ;
#10105=DIRECTION ( 'NONE',  ( -0.7071067811865500152, 1.645406930227287500E-16, 0.7071067811865451302 ) ) ;
#10108=EDGE_CURVE ( 'NONE', #7803, #172, #15905, .T. ) ;
#10109=VECTOR ( 'NONE', #30714, 1000.000000000000227 ) ;
#10110=AXIS2_PLACEMENT_3D ( 'NONE', #11539, #23726, #8080 ) ;
#10111=DIRECTION ( 'NONE',  ( -1.000000000000000000, 0.000000000000000000, 0.000000000000000000 ) ) ;
#10113=EDGE_CURVE ( 'NONE', #3294, #32472, #9929, .T. ) ;
#10115=PLANE ( 'NONE',  #32125 ) ;
#10117=PLANE ( 'NONE',  #18862 ) ;
#10118=CARTESIAN_POINT ( 'NONE',  ( 3.992867117591230919, 8.524771480177550487, 7.499999999999990230 ) ) ;
#10119=CARTESIAN_POINT ( 'NONE',  ( -14.52509594610762456, 21.97885917798744870, 10.49999999999999467 ) ) ;
#10120=CARTESIAN_POINT ( 'NONE',  ( -13.37378135583787220, 20.59160479820268108, 7.000000000000000000 ) ) ;
#10122=CARTESIAN_POINT ( 'NONE',  ( -3.000488737322915878, 30.46850471150003159, 7.000000000000000000 ) ) ;
#10123=ORIENTED_EDGE ( 'NONE', *, *, #17055, .F. ) ;
#10124=ADVANCED_FACE ( 'NONE', ( #4022 ), #585, .T. ) ;
#10126=CARTESIAN_POINT ( 'NONE',  ( -5.767236651883564491, 13.71142893291686349, 11.00000000000000000 ) ) ;
#10132=CARTESIAN_POINT ( 'NONE',  ( -10.20374679324127776, 33.03312760923218150, 10.49999999999999822 ) ) ;
#10137=CARTESIAN_POINT ( 'NONE',  ( 7.852310722358922135, 10.04909572729066269, 10.49999999999999822 ) ) ;
#10138=CARTESIAN_POINT ( 'NONE',  ( 11.22168704032814013, 31.70696390855182756, 10.83333333333333393 ) ) ;
#10140=ORIENTED_EDGE ( 'NONE', *, *, #6400, .T. ) ;
#10144=EDGE_CURVE ( 'NONE', #14996, #15350, #28860, .T. ) ;
#10145=AXIS2_PLACEMENT_3D ( 'NONE', #22864, #3980, #19832 ) ;
#10146=CARTESIAN_POINT ( 'NONE',  ( -3.503793317224518145, 8.420815634768723967, 7.000000000000000000 ) ) ;
#10149=CYLINDRICAL_SURFACE ( 'NONE', #34919, 6.000000000000001776 ) ;
#10150=AXIS2_PLACEMENT_3D ( 'NONE', #36675, #8845, #9238 ) ;
#10151=CARTESIAN_POINT ( 'NONE',  ( -12.80736835487442349, 15.68301270189233954, 9.000000000000001776 ) ) ;
#10152=VERTEX_POINT ( 'NONE', #38963 ) ;
#10157=ORIENTED_EDGE ( 'NONE', *, *, #4307, .T. ) ;
#10158=PRODUCT_CONTEXT ( 'NONE', #26987, 'mechanical' ) ;
#10160=LINE ( 'NONE', #7097, #11892 ) ;
#10161=CARTESIAN_POINT ( 'NONE',  ( -4.360894802593465513, 8.147407145008980223, 7.102474990965859547 ) ) ;
#10162=EDGE_CURVE ( 'NONE', #7910, #13732, #37938, .T. ) ;
#10164=FACE_OUTER_BOUND ( 'NONE', #38501, .T. ) ;
#10165=ORIENTED_EDGE ( 'NONE', *, *, #32101, .T. ) ;
#10169=CARTESIAN_POINT ( 'NONE',  ( 12.37161151015161842, 14.01709413980860219, 7.202682876670052359 ) ) ;
#10170=DIRECTION ( 'NONE',  ( 0.000000000000000000, 0.000000000000000000, -1.000000000000000000 ) ) ;
#10174=AXIS2_PLACEMENT_3D ( 'NONE', #34811, #6964, #28513 ) ;
#10177=CARTESIAN_POINT ( 'NONE',  ( -5.440908595777636414, 35.94977745735568675, 7.000000000000000000 ) ) ;
#10179=ORIENTED_EDGE ( 'NONE', *, *, #12037, .F. ) ;
#10183=DIRECTION ( 'NONE',  ( 0.000000000000000000, 0.000000000000000000, 1.000000000000000000 ) ) ;
#10188=CARTESIAN_POINT ( 'NONE',  ( 14.44622163125243830, 19.97613264340516537, 10.49999999999999822 ) ) ;
#10190=CARTESIAN_POINT ( 'NONE',  ( -13.41480434723648685, 15.78756373729235740, 7.392564007638123158 ) ) ;
#10194=DIRECTION ( 'NONE',  ( -0.000000000000000000, -0.000000000000000000, -1.000000000000000000 ) ) ;
#10195=EDGE_LOOP ( 'NONE', ( #34104, #39769, #1296, #19566 ) ) ;
#10197=DIRECTION ( 'NONE',  ( 1.000000000000000000, 0.000000000000000000, 0.000000000000000000 ) ) ;
#10203=ORIENTED_EDGE ( 'NONE', *, *, #5548, .F. ) ;
#10207=CIRCLE ( 'NONE', #1131, 6.000000000000005329 ) ;
#10216=AXIS2_PLACEMENT_3D ( 'NONE', #31923, #35384, #4091 ) ;
#10223=EDGE_LOOP ( 'NONE', ( #11765, #10470, #25039 ) ) ;
#10226=VERTEX_POINT ( 'NONE', #38558 ) ;
#10228=CARTESIAN_POINT ( 'NONE',  ( 0.4999999999999990563, 31.00000000000000355, 9.000000000000001776 ) ) ;
#10230=LINE ( 'NONE', #6571, #18598 ) ;
#10231=TOROIDAL_SURFACE ( 'NONE', #32962, 1.000000000000000000, 0.5000000000000000000 ) ;
#10235=DIRECTION ( 'NONE',  ( -0.9510565162951543083, -0.3090169943749450088, 0.000000000000000000 ) ) ;
#10237=EDGE_LOOP ( 'NONE', ( #1097, #34185, #31821, #6536 ) ) ;
#10239=ADVANCED_FACE ( 'NONE', ( #7679 ), #26289, .T. ) ;
#10240=CARTESIAN_POINT ( 'NONE',  ( 3.610593701936713806, 31.83882289796390097, 10.49999999999999645 ) ) ;
#10247=VERTEX_POINT ( 'NONE', #30022 ) ;
#10248=ADVANCED_FACE ( 'NONE', ( #32267 ), #39361, .F. ) ;
#10249=AXIS2_PLACEMENT_3D ( 'NONE', #7314, #35768, #32528 ) ;
#10251=DIRECTION ( 'NONE',  ( -0.9135454576426059736, -0.4067366430757888285, 0.000000000000000000 ) ) ;
#10252=TOROIDAL_SURFACE ( 'NONE', #30400, 1.000000000000000000, 0.5000000000000000000 ) ;
#10253=CARTESIAN_POINT ( 'NONE',  ( -14.26584774442725845, 27.13525491562436542, 7.000000000000000000 ) ) ;
#10254=VECTOR ( 'NONE', #29747, 999.9999999999998863 ) ;
#10256=CARTESIAN_POINT ( 'NONE',  ( -11.36213480545077736, 32.05769576588223657, 10.87262190629438408 ) ) ;
#10258=DIRECTION ( 'NONE',  ( 0.9510565162951543083, 0.3090169943749450088, 0.000000000000000000 ) ) ;
#10259=VERTEX_POINT ( 'NONE', #29416 ) ;
#10262=ADVANCED_FACE ( 'NONE', ( #13771 ), #7471, .T. ) ;
#10263=CARTESIAN_POINT ( 'NONE',  ( 3.666817917346630207, 8.455467583238284845, 10.83333333333332860 ) ) ;
#10265=DIRECTION ( 'NONE',  ( -1.000000000000000000, 0.000000000000000000, 0.000000000000000000 ) ) ;
#10266=LINE ( 'NONE', #13509, #22900 ) ;
#10268=CARTESIAN_POINT ( 'NONE',  ( -1.828660225306043108, 9.087095699275881344, 9.500000000000000000 ) ) ;
#10272=DIRECTION ( 'NONE',  ( 0.000000000000000000, -0.000000000000000000, -1.000000000000000000 ) ) ;
#10274=CARTESIAN_POINT ( 'NONE',  ( 7.824485034907088021, 10.87986945260446170, 7.499999999999999112 ) ) ;
#10276=ORIENTED_EDGE ( 'NONE', *, *, #4738, .F. ) ;
#10278=EDGE_LOOP ( 'NONE', ( #26952, #32956, #21131, #9286 ) ) ;
#10283=VECTOR ( 'NONE', #19661, 1000.000000000000114 ) ;
#10290=CARTESIAN_POINT ( 'NONE',  ( 2.518583951651052644, 7.712953814960687104, 7.000000000000000000 ) ) ;
#10293=ORIENTED_EDGE ( 'NONE', *, *, #712, .T. ) ;
#10296=VECTOR ( 'NONE', #27345, 1000.000000000000114 ) ;
#10300=CARTESIAN_POINT ( 'NONE',  ( -13.30736791469135483, 15.68301270237671474, 10.49999999999999822 ) ) ;
#10303=ORIENTED_EDGE ( 'NONE', *, *, #34779, .F. ) ;
#10304=EDGE_LOOP ( 'NONE', ( #12126, #9349, #3081, #28928 ) ) ;
#10305=DIRECTION ( 'NONE',  ( -0.1045284632676569680, -0.9945218953682730678, 0.000000000000000000 ) ) ;
#10307=VECTOR ( 'NONE', #6666, 999.9999999999998863 ) ;
#10308=AXIS2_PLACEMENT_3D ( 'NONE', #14774, #21459, #2184 ) ;
#10312=DIRECTION ( 'NONE',  ( -0.2876062384759508483, 0.6459741880212531706, -0.7071067811865455743 ) ) ;
#10314=EDGE_CURVE ( 'NONE', #29868, #39481, #13956, .T. ) ;
#10315=VECTOR ( 'NONE', #15057, 1000.000000000000114 ) ;
#10316=CARTESIAN_POINT ( 'NONE',  ( -11.11016527260153808, 31.83082137946488643, 7.000000000000000000 ) ) ;
#10321=VERTEX_POINT ( 'NONE', #32882 ) ;
#10323=DIRECTION ( 'NONE',  ( -0.9781476007338041345, 0.2079116908177664202, 0.000000000000000000 ) ) ;
#10326=CARTESIAN_POINT ( 'NONE',  ( 2.317734025672765430, 9.191051544684729180, 10.00000000000000000 ) ) ;
#10327=B_SPLINE_CURVE_WITH_KNOTS ( 'NONE', 3,
 ( #7666, #22696, #7863, #20069, #14163, #13962 ),
 .UNSPECIFIED., .F., .F.,
 ( 4, 2, 4 ),
 ( 0.000000000000000000, 0.5000000000000000000, 1.000000000000000000 ),
 .UNSPECIFIED. ) ;
#10330=CARTESIAN_POINT ( 'NONE',  ( -12.37435565298220119, 15.93301270189233598, 7.499999999999993783 ) ) ;
#10337=VERTEX_POINT ( 'NONE', #35723 ) ;
#10339=ORIENTED_EDGE ( 'NONE', *, *, #25010, .F. ) ;
#10340=EDGE_CURVE ( 'NONE', #4096, #36923, #17445, .T. ) ;
#10342=CARTESIAN_POINT ( 'NONE',  ( 14.47283171447378969, 21.48159823030311344, 10.99999999999999289 ) ) ;
#10343=ORIENTED_EDGE ( 'NONE', *, *, #7448, .T. ) ;
#10345=EDGE_CURVE ( 'NONE', #34172, #18383, #2279, .T. ) ;
#10346=CARTESIAN_POINT ( 'NONE',  ( 9.160254037844365982, 18.36602540378440196, 10.49999999999999822 ) ) ;
#10348=CARTESIAN_POINT ( 'NONE',  ( -8.633502029282189127, 11.46765470489704164, 9.500000000000000000 ) ) ;
#10350=B_SPLINE_SURFACE_WITH_KNOTS ( 'NONE', 1, 3, ( 
 ( #13119, #10082, #25715, #26324, #25508, #34869, #7019, #10687, #25914, #20035 ),
 ( #7423, #29369, #16788, #1341, #38109, #1546, #22663, #35066, #38718, #16585 ) ),
 .UNSPECIFIED., .F., .F., .F.,
 ( 2, 2 ),
 ( 4, 2, 2, 2, 4 ),
 ( 0.000000000000000000, 1.000000000000000000 ),
 ( 1.344962617103288904, 1.737661698802012822, 2.130360780500736961, 2.523059862199461101, 2.915758943898185240 ),
 .UNSPECIFIED. ) ;
#10353=CARTESIAN_POINT ( 'NONE',  ( -2.256323172317921788, 14.28970123917155277, 7.000000000000000000 ) ) ;
#10356=EDGE_CURVE ( 'NONE', #25471, #20190, #15238, .T. ) ;
#10359=DIRECTION ( 'NONE',  ( -0.000000000000000000, -0.000000000000000000, -1.000000000000000000 ) ) ;
#10360=PLANE ( 'NONE',  #36442 ) ;
#10363=ORIENTED_EDGE ( 'NONE', *, *, #37200, .F. ) ;
#10364=CARTESIAN_POINT ( 'NONE',  ( -2.256323172317922232, 14.28970123917155277, 7.000000000000000000 ) ) ;
#10369=EDGE_CURVE ( 'NONE', #37600, #10337, #5439, .T. ) ;
#10375=CARTESIAN_POINT ( 'NONE',  ( 10.44103466624280507, 32.57396620494213124, 7.000000000000000000 ) ) ;
#10378=LINE ( 'NONE', #23374, #5062 ) ;
#10379=ORIENTED_EDGE ( 'NONE', *, *, #13164, .T. ) ;
#10383=LINE ( 'NONE', #31314, #7518 ) ;
#10392=CARTESIAN_POINT ( 'NONE',  ( 11.81630298851978900, 31.79381426990546089, 10.49999999999999822 ) ) ;
#10393=ORIENTED_EDGE ( 'NONE', *, *, #29147, .T. ) ;
#10396=CARTESIAN_POINT ( 'NONE',  ( 2.672146553953313131, 12.33340603770390764, 10.50000000000000000 ) ) ;
#10398=VERTEX_POINT ( 'NONE', #28668 ) ;
#10400=B_SPLINE_CURVE_WITH_KNOTS ( 'NONE', 3,
 ( #29950, #13910, #32610, #36260, #10666, #8422 ),
 .UNSPECIFIED., .F., .F.,
 ( 4, 2, 4 ),
 ( 0.000000000000000000, 0.5000000000000000000, 1.000000000000000000 ),
 .UNSPECIFIED. ) ;
#10401=DIRECTION ( 'NONE',  ( -1.000000000000000000, 0.000000000000000000, 0.000000000000000000 ) ) ;
#10402=ORIENTED_EDGE ( 'NONE', *, *, #27524, .F. ) ;
#10404=ADVANCED_FACE ( 'NONE', ( #29071 ), #13024, .F. ) ;
#10409=CARTESIAN_POINT ( 'NONE',  ( -2.036571916123810055, 8.108948098542073879, 7.000000000000000000 ) ) ;
#10411=CARTESIAN_POINT ( 'NONE',  ( 1.000000000000000000, 37.00000000000000711, 11.00000000000000000 ) ) ;
#10412=CARTESIAN_POINT ( 'NONE',  ( 0.000000000000000000, 22.50000000000000355, 7.000000000000000000 ) ) ;
#10419=CARTESIAN_POINT ( 'NONE',  ( -4.524139159579186220, 31.43208625488817276, 10.50000000000000000 ) ) ;
#10420=VERTEX_POINT ( 'NONE', #31522 ) ;
#10429=DIRECTION ( 'NONE',  ( 0.4999999999999920064, -0.8660254037844432595, 0.000000000000000000 ) ) ;
#10430=VECTOR ( 'NONE', #21556, 999.9999999999998863 ) ;
#10431=ORIENTED_EDGE ( 'NONE', *, *, #28150, .T. ) ;
#10433=DIRECTION ( 'NONE',  ( 1.000000000000000000, 0.000000000000000000, 0.000000000000000000 ) ) ;
#10435=DIRECTION ( 'NONE',  ( -0.000000000000000000, -0.000000000000000000, -1.000000000000000000 ) ) ;
#10436=ORIENTED_EDGE ( 'NONE', *, *, #306, .T. ) ;
#10439=CARTESIAN_POINT ( 'NONE',  ( -21.55328011382844977, 16.02264588471131646, 11.00000000000000000 ) ) ;
#10443=EDGE_CURVE ( 'NONE', #14016, #34496, #22767, .T. ) ;
#10444=CARTESIAN_POINT ( 'NONE',  ( 0.5000000000000001110, 37.00000000000000711, 7.000000000000000000 ) ) ;
#10445=LINE ( 'NONE', #13896, #2433 ) ;
#10446=ORIENTED_EDGE ( 'NONE', *, *, #23335, .F. ) ;
#10449=VECTOR ( 'NONE', #21158, 1000.000000000000000 ) ;
#10456=AXIS2_PLACEMENT_3D ( 'NONE', #9122, #2826, #12565 ) ;
#10457=DIRECTION ( 'NONE',  ( -0.6123724356957971349, 0.3535533905932787824, -0.7071067811865427988 ) ) ;
#10459=FACE_OUTER_BOUND ( 'NONE', #23869, .T. ) ;
#10461=ADVANCED_FACE ( 'NONE', ( #19525 ), #29277, .F. ) ;
#10463=CARTESIAN_POINT ( 'NONE',  ( -6.832768599200551130, 35.70122713809554682, 10.49999999999999822 ) ) ;
#10464=DIRECTION ( 'NONE',  ( 0.3090169943749573322, 0.9510565162951504226, 0.000000000000000000 ) ) ;
#10466=CARTESIAN_POINT ( 'NONE',  ( 14.86556419889027048, 20.43481210330100595, 10.63089969389956835 ) ) ;
#10467=CARTESIAN_POINT ( 'NONE',  ( 9.343266739736582949, 17.68301270189217433, 11.00000000000000000 ) ) ;
#10470=ORIENTED_EDGE ( 'NONE', *, *, #3640, .T. ) ;
#10471=AXIS2_PLACEMENT_3D ( 'NONE', #380, #31647, #24751 ) ;
#10474=VECTOR ( 'NONE', #5265, 1000.000000000000114 ) ;
#10477=DIRECTION ( 'NONE',  ( 0.6445931928399328825, 0.000000000000000000, -0.7645257456387070105 ) ) ;
#10479=EDGE_LOOP ( 'NONE', ( #21474, #33482, #19231 ) ) ;
#10483=DIRECTION ( 'NONE',  ( 0.3090169943749450643, -0.9510565162951544194, 0.000000000000000000 ) ) ;
#10491=DIRECTION ( 'NONE',  ( 1.000000000000000000, 0.000000000000000000, 0.000000000000000000 ) ) ;
#10493=CARTESIAN_POINT ( 'NONE',  ( 1.590043107810628076, 12.61456814725305442, 10.50000000000000000 ) ) ;
#10496=B_SPLINE_CURVE_WITH_KNOTS ( 'NONE', 3,
 ( #11803, #15446, #18110, #24989 ),
 .UNSPECIFIED., .F., .F.,
 ( 4, 4 ),
 ( 0.6000000000734145855, 1.000000000000000000 ),
 .UNSPECIFIED. ) ;
#10498=CARTESIAN_POINT ( 'NONE',  ( -11.44473057578096942, 31.45924896672619298, 9.500000000000000000 ) ) ;
#10499=EDGE_LOOP ( 'NONE', ( #1166, #20251, #26643, #11937 ) ) ;
#10502=EDGE_CURVE ( 'NONE', #23547, #25420, #12255, .T. ) ;
#10505=AXIS2_PLACEMENT_3D ( 'NONE', #12563, #3417, #15813 ) ;
#10506=ORIENTED_EDGE ( 'NONE', *, *, #4712, .F. ) ;
#10507=CARTESIAN_POINT ( 'NONE',  ( -6.811226782241547539, 35.33967249274200384, 10.50000000000000355 ) ) ;
#10509=CARTESIAN_POINT ( 'NONE',  ( 3.503793317224327186, 8.420815634768674229, 7.000000000000000000 ) ) ;
#10512=LINE ( 'NONE', #39143, #17211 ) ;
#10513=ADVANCED_FACE ( 'NONE', ( #9789 ), #16080, .T. ) ;
#10514=DIRECTION ( 'NONE',  ( -0.6691306063588570163, 0.7431448254773953543, -0.000000000000000000 ) ) ;
#10515=DIRECTION ( 'NONE',  ( 0.000000000000000000, 0.000000000000000000, 1.000000000000000000 ) ) ;
#10516=DIRECTION ( 'NONE',  ( 0.2079116908177657541, 0.9781476007338044676, -1.803346454958047642E-16 ) ) ;
#10519=CARTESIAN_POINT ( 'NONE',  ( 14.44277748876681855, 26.55045409923015853, 7.500000000000000888 ) ) ;
#10520=ORIENTED_EDGE ( 'NONE', *, *, #20565, .F. ) ;
#10523=CARTESIAN_POINT ( 'NONE',  ( 12.67417846324118358, 14.47720745114811436, 7.499999999999997335 ) ) ;
#10525=CARTESIAN_POINT ( 'NONE',  ( -13.57128027507772039, 27.95460132400015496, 10.49999999999999822 ) ) ;
#10527=EDGE_CURVE ( 'NONE', #16505, #24016, #4289, .T. ) ;
#10528=DIRECTION ( 'NONE',  ( 0.000000000000000000, 0.000000000000000000, -1.000000000000000000 ) ) ;
#10533=CIRCLE ( 'NONE', #11178, 0.5000000000000000000 ) ;
#10536=B_SPLINE_CURVE_WITH_KNOTS ( 'NONE', 3,
 ( #16257, #34743, #22338, #15455, #6894, #15657 ),
 .UNSPECIFIED., .F., .F.,
 ( 4, 2, 4 ),
 ( 0.000000000000000000, 0.5000000000000000000, 1.000000000000000000 ),
 .UNSPECIFIED. ) ;
#10538=DIRECTION ( 'NONE',  ( 1.000000000000000000, 0.000000000000000000, 0.000000000000000000 ) ) ;
#10540=EDGE_LOOP ( 'NONE', ( #36271, #20656, #14297, #2080, #35946 ) ) ;
#10544=CARTESIAN_POINT ( 'NONE',  ( 4.794796183863160977, 36.71301971979253409, 7.000000000000000000 ) ) ;
#10545=ORIENTED_EDGE ( 'NONE', *, *, #28354, .F. ) ;
#10547=DIRECTION ( 'NONE',  ( -0.000000000000000000, -0.000000000000000000, -1.000000000000000000 ) ) ;
#10549=VECTOR ( 'NONE', #15248, 1000.000000000000000 ) ;
#10556=CIRCLE ( 'NONE', #7317, 15.00000000000000000 ) ;
#10560=B_SPLINE_CURVE_WITH_KNOTS ( 'NONE', 3,
 ( #8721, #11967, #33910, #5662 ),
 .UNSPECIFIED., .F., .F.,
 ( 4, 4 ),
 ( 0.000000000000000000, 1.000000000000000000 ),
 .UNSPECIFIED. ) ;
#10562=CARTESIAN_POINT ( 'NONE',  ( -12.62435565298219764, 16.36602540378455828, 10.50000000000000000 ) ) ;
#10564=CARTESIAN_POINT ( 'NONE',  ( -11.48173768534023154, 32.16538668264431777, 10.49999999999999822 ) ) ;
#10565=ORIENTED_EDGE ( 'NONE', *, *, #19717, .F. ) ;
#10566=CARTESIAN_POINT ( 'NONE',  ( 3.118675362266300599, 7.827785988992891575, 7.000000000000000000 ) ) ;
#10567=LINE ( 'NONE', #35354, #25399 ) ;
#10568=CYLINDRICAL_SURFACE ( 'NONE', #9799, 0.5000000000000004441 ) ;
#10569=EDGE_CURVE ( 'NONE', #39330, #9244, #35779, .T. ) ;
#10571=AXIS2_PLACEMENT_3D ( 'NONE', #5174, #2132, #2335 ) ;
#10573=ORIENTED_EDGE ( 'NONE', *, *, #36674, .F. ) ;
#10574=FACE_OUTER_BOUND ( 'NONE', #35788, .T. ) ;
#10575=CARTESIAN_POINT ( 'NONE',  ( -0.6308996938995719006, 37.50000000000000711, 10.49999999999999822 ) ) ;
#10576=AXIS2_PLACEMENT_3D ( 'NONE', #37197, #21747, #19108 ) ;
#10578=DIRECTION ( 'NONE',  ( -0.8660254037844362651, 0.5000000000000043299, 0.000000000000000000 ) ) ;
#10579=DIRECTION ( 'NONE',  ( 0.6691306063588561281, -0.7431448254773961315, 0.000000000000000000 ) ) ;
#10580=ORIENTED_EDGE ( 'NONE', *, *, #19102, .T. ) ;
#10582=CIRCLE ( 'NONE', #37205, 6.000000000000010658 ) ;
#10586=EDGE_LOOP ( 'NONE', ( #24496, #30985, #22011, #37133 ) ) ;
#10587=EDGE_LOOP ( 'NONE', ( #22604, #20788, #20401, #38216 ) ) ;
#10590=VECTOR ( 'NONE', #16775, 1000.000000000000000 ) ;
#10593=AXIS2_PLACEMENT_3D ( 'NONE', #34254, #15162, #15560 ) ;
#10594=DIRECTION ( 'NONE',  ( -0.1470157664652027019, -0.6916548014802211819, -0.7071067811865510144 ) ) ;
#10595=ORIENTED_EDGE ( 'NONE', *, *, #19818, .T. ) ;
#10598=CARTESIAN_POINT ( 'NONE',  ( 3.597409820281487480, 14.42008525284347087, 7.000000000000000000 ) ) ;
#10599=ORIENTED_EDGE ( 'NONE', *, *, #2466, .T. ) ;
#10603=EDGE_CURVE ( 'NONE', #20519, #25405, #5094, .T. ) ;
#10611=FACE_OUTER_BOUND ( 'NONE', #9598, .T. ) ;
#10613=AXIS2_PLACEMENT_3D ( 'NONE', #12160, #23955, #30254 ) ;
#10614=PLANE ( 'NONE',  #18107 ) ;
#10615=DIRECTION ( 'NONE',  ( -0.000000000000000000, -0.000000000000000000, -1.000000000000000000 ) ) ;
#10619=EDGE_CURVE ( 'NONE', #26362, #28707, #19819, .T. ) ;
#10625=VECTOR ( 'NONE', #16219, 999.9999999999998863 ) ;
#10626=ORIENTED_EDGE ( 'NONE', *, *, #22993, .F. ) ;
#10628=EDGE_CURVE ( 'NONE', #10152, #21190, #5487, .T. ) ;
#10630=CARTESIAN_POINT ( 'NONE',  ( -13.24038105676664578, 15.43301270189234309, 10.50000000000000000 ) ) ;
#10632=ORIENTED_EDGE ( 'NONE', *, *, #17791, .T. ) ;
#10634=FACE_OUTER_BOUND ( 'NONE', #30682, .T. ) ;
#10635=VERTEX_POINT ( 'NONE', #4892 ) ;
#10637=DIRECTION ( 'NONE',  ( -0.000000000000000000, -0.000000000000000000, -1.000000000000000000 ) ) ;
#10639=CARTESIAN_POINT ( 'NONE',  ( 13.35472669706387272, 15.66947210016787118, 7.455686640544899824 ) ) ;
#10640=VECTOR ( 'NONE', #25094, 1000.000000000000114 ) ;
#10641=ORIENTED_EDGE ( 'NONE', *, *, #8926, .T. ) ;
#10644=CARTESIAN_POINT ( 'NONE',  ( -12.37435565298220119, 15.93301270189233598, 7.499999999999993783 ) ) ;
#10646=VERTEX_POINT ( 'NONE', #14033 ) ;
#10648=DIRECTION ( 'NONE',  ( -0.3090169943749448977, 0.9510565162951543083, 0.000000000000000000 ) ) ;
#10649=DIRECTION ( 'NONE',  ( 0.7032331762534119735, 0.07391278520356013571, -0.7071067811865404673 ) ) ;
#10650=VERTEX_POINT ( 'NONE', #17302 ) ;
#10651=ADVANCED_FACE ( 'NONE', ( #30079 ), #2252, .F. ) ;
#10653=ADVANCED_FACE ( 'NONE', ( #7736 ), #39413, .T. ) ;
#10655=VECTOR ( 'NONE', #11818, 1000.000000000000114 ) ;
#10657=EDGE_LOOP ( 'NONE', ( #28277, #9112, #16189, #23388, #22742, #10061, #27003 ) ) ;
#10660=VECTOR ( 'NONE', #29310, 1000.000000000000114 ) ;
#10661=DIRECTION ( 'NONE',  ( -0.000000000000000000, -0.000000000000000000, -1.000000000000000000 ) ) ;
#10662=CARTESIAN_POINT ( 'NONE',  ( -5.440908595777636414, 35.94977745735568675, 7.500000000000000888 ) ) ;
#10663=ADVANCED_FACE ( 'NONE', ( #11193 ), #8345, .F. ) ;
#10665=CARTESIAN_POINT ( 'NONE',  ( -11.50946345163895934, 31.52577281809603704, 10.49999999999999822 ) ) ;
#10666=CARTESIAN_POINT ( 'NONE',  ( 6.557822374958314882, 35.99981354310111215, 10.63089969389957368 ) ) ;
#10667=ADVANCED_FACE ( 'NONE', ( #35980 ), #23704, .T. ) ;
#10669=EDGE_LOOP ( 'NONE', ( #26340, #22035, #17526 ) ) ;
#10670=DIRECTION ( 'NONE',  ( 0.8660254037844364872, -0.5000000000000038858, 0.000000000000000000 ) ) ;
#10673=CARTESIAN_POINT ( 'NONE',  ( 14.81197284684443360, 20.44044478137463727, 10.76099332938163577 ) ) ;
#10674=PLANE ( 'NONE',  #12533 ) ;
#10681=CARTESIAN_POINT ( 'NONE',  ( -2.036571916123810055, 8.108948098542073879, 7.499999999999997335 ) ) ;
#10683=ORIENTED_EDGE ( 'NONE', *, *, #18215, .F. ) ;
#10685=ORIENTED_EDGE ( 'NONE', *, *, #37560, .T. ) ;
#10687=CARTESIAN_POINT ( 'NONE',  ( 14.18553059334559308, 26.06413323176228047, 10.49999999999999822 ) ) ;
#10694=ORIENTED_EDGE ( 'NONE', *, *, #20086, .F. ) ;
#10697=LINE ( 'NONE', #10493, #5643 ) ;
#10698=DIRECTION ( 'NONE',  ( -0.9781476007338042455, 0.2079116908177663370, 0.000000000000000000 ) ) ;
#10699=CIRCLE ( 'NONE', #11999, 6.000000000000003553 ) ;
#10700=ORIENTED_EDGE ( 'NONE', *, *, #7030, .F. ) ;
#10706=EDGE_CURVE ( 'NONE', #16758, #12080, #26424, .T. ) ;
#10710=ORIENTED_EDGE ( 'NONE', *, *, #30647, .T. ) ;
#10711=DIRECTION ( 'NONE',  ( 0.8660254037844364872, -0.5000000000000038858, 0.000000000000000000 ) ) ;
#10714=DIRECTION ( 'NONE',  ( -0.6691306063588561281, 0.7431448254773961315, 0.000000000000000000 ) ) ;
#10715=ORIENTED_EDGE ( 'NONE', *, *, #24933, .F. ) ;
#10719=CIRCLE ( 'NONE', #5520, 6.000000000000005329 ) ;
#10725=AXIS2_PLACEMENT_3D ( 'NONE', #9523, #16410, #34696 ) ;
#10726=ORIENTED_EDGE ( 'NONE', *, *, #8628, .T. ) ;
#10728=VECTOR ( 'NONE', #30080, 1000.000000000000000 ) ;
#10729=DIRECTION ( 'NONE',  ( 0.8660254037844432595, 0.4999999999999921729, 0.000000000000000000 ) ) ;
#10735=FACE_OUTER_BOUND ( 'NONE', #92, .T. ) ;
#10741=LINE ( 'NONE', #21431, #4048 ) ;
#10742=ORIENTED_EDGE ( 'NONE', *, *, #11766, .F. ) ;
#10744=EDGE_LOOP ( 'NONE', ( #12159, #15730, #9806, #38573 ) ) ;
#10746=CARTESIAN_POINT ( 'NONE',  ( -9.427394962683591118, 11.06314620782489833, 10.49999999999999822 ) ) ;
#10747=EDGE_LOOP ( 'NONE', ( #51, #28130, #31233 ) ) ;
#10749=ADVANCED_FACE ( 'NONE', ( #29473 ), #32539, .F. ) ;
#10752=AXIS2_PLACEMENT_3D ( 'NONE', #7973, #17343, #39058 ) ;
#10754=ORIENTED_EDGE ( 'NONE', *, *, #32131, .F. ) ;
#10756=VECTOR ( 'NONE', #35247, 1000.000000000000000 ) ;
#10758=EDGE_CURVE ( 'NONE', #24136, #11294, #30285, .T. ) ;
#10761=EDGE_CURVE ( 'NONE', #18018, #38835, #36042, .T. ) ;
#10762=CARTESIAN_POINT ( 'NONE',  ( -6.651296319737220131, 27.81603774131167839, 9.000000000000001776 ) ) ;
#10763=DIRECTION ( 'NONE',  ( -0.9945218953682745111, -0.1045284632676436454, 0.000000000000000000 ) ) ;
#10765=CARTESIAN_POINT ( 'NONE',  ( -10.36702044712415116, 31.16169077310601665, 9.500000000000000000 ) ) ;
#10767=DIRECTION ( 'NONE',  ( 0.000000000000000000, 0.000000000000000000, 1.000000000000000000 ) ) ;
#10769=CARTESIAN_POINT ( 'NONE',  ( -13.95683075005229767, 28.08631143191951196, 10.50000000000000533 ) ) ;
#10774=CYLINDRICAL_SURFACE ( 'NONE', #28104, 0.5000000000000004441 ) ;
#10776=EDGE_CURVE ( 'NONE', #27469, #27237, #26827, .T. ) ;
#10777=EDGE_CURVE ( 'NONE', #38307, #34486, #1002, .T. ) ;
#10781=LINE ( 'NONE', #4072, #32974 ) ;
#10783=AXIS2_PLACEMENT_3D ( 'NONE', #28603, #19256, #13157 ) ;
#10785=VECTOR ( 'NONE', #6429, 1000.000000000000000 ) ;
#10789=CARTESIAN_POINT ( 'NONE',  ( -9.819582157326459892, 24.63911342745442568, 10.50000000000000533 ) ) ;
#10790=ORIENTED_EDGE ( 'NONE', *, *, #8628, .F. ) ;
#10793=CARTESIAN_POINT ( 'NONE',  ( -5.440908595777636414, 35.94977745735568675, 7.500000000000000888 ) ) ;
#10794=DIRECTION ( 'NONE',  ( 0.5877852522924792433, 0.8090169943749431214, 0.000000000000000000 ) ) ;
#10797=VERTEX_POINT ( 'NONE', #36573 ) ;
#10800=DIRECTION ( 'NONE',  ( -0.9781476007338072431, -0.2079116908177519041, 0.000000000000000000 ) ) ;
#10801=LINE ( 'NONE', #26231, #480 ) ;
#10805=EDGE_CURVE ( 'NONE', #35366, #21446, #32146, .T. ) ;
#10806=DIRECTION ( 'NONE',  ( 0.8660254037844363761, -0.5000000000000038858, 0.000000000000000000 ) ) ;
#10809=DIRECTION ( 'NONE',  ( -0.5000000000000038858, -0.8660254037844363761, 0.000000000000000000 ) ) ;
#10811=ORIENTED_EDGE ( 'NONE', *, *, #4069, .T. ) ;
#10814=DIRECTION ( 'NONE',  ( 1.000000000000000000, 0.000000000000000000, 0.000000000000000000 ) ) ;
#10816=AXIS2_PLACEMENT_3D ( 'NONE', #18585, #28115, #37066 ) ;
#10817=CARTESIAN_POINT ( 'NONE',  ( -13.49038105676664223, 15.86602540378456361, 11.00000000000000000 ) ) ;
#10819=DIRECTION ( 'NONE',  ( -1.000000000000000000, 0.000000000000000000, 0.000000000000000000 ) ) ;
#10826=DIRECTION ( 'NONE',  ( 1.000000000000000000, 0.000000000000000000, 0.000000000000000000 ) ) ;
#10830=ORIENTED_EDGE ( 'NONE', *, *, #1026, .F. ) ;
#10835=ORIENTED_EDGE ( 'NONE', *, *, #18486, .F. ) ;
#10839=DIRECTION ( 'NONE',  ( -1.000000000000000000, 0.000000000000000000, 0.000000000000000000 ) ) ;
#10841=CARTESIAN_POINT ( 'NONE',  ( -14.31603901957233660, 19.98981538725089990, 7.000000000000000000 ) ) ;
#10842=CIRCLE ( 'NONE', #13409, 0.5000000000000004441 ) ;
#10844=ORIENTED_EDGE ( 'NONE', *, *, #11505, .T. ) ;
#10853=ORIENTED_EDGE ( 'NONE', *, *, #30990, .F. ) ;
#10855=EDGE_CURVE ( 'NONE', #26924, #22721, #30179, .T. ) ;
#10857=AXIS2_PLACEMENT_3D ( 'NONE', #16568, #16975, #19205 ) ;
#10860=ORIENTED_EDGE ( 'NONE', *, *, #37827, .F. ) ;
#10864=CARTESIAN_POINT ( 'NONE',  ( 14.36830325120613239, 20.48707633493483371, 7.500000000000010658 ) ) ;
#10865=EDGE_CURVE ( 'NONE', #32296, #22181, #27717, .T. ) ;
#10867=AXIS2_PLACEMENT_3D ( 'NONE', #28128, #31378, #505 ) ;
#10870=FACE_OUTER_BOUND ( 'NONE', #29739, .T. ) ;
#10871=CARTESIAN_POINT ( 'NONE',  ( 12.92073081513896859, 15.61756285494237773, 10.99999999999999822 ) ) ;
#10875=CARTESIAN_POINT ( 'NONE',  ( 7.267999511063016449, 35.13630417120400296, 7.000000000000000000 ) ) ;
#10877=EDGE_CURVE ( 'NONE', #17593, #9209, #18887, .T. ) ;
#10878=AXIS2_PLACEMENT_3D ( 'NONE', #15155, #15555, #3164 ) ;
#10880=CARTESIAN_POINT ( 'NONE',  ( -8.472151273871419974, 28.78272654129072095, 10.50000000000000000 ) ) ;
#10885=CARTESIAN_POINT ( 'NONE',  ( 3.914034194965611668, 30.06176806842419680, 7.000000000000000000 ) ) ;
#10890=CARTESIAN_POINT ( 'NONE',  ( -11.11016527260153097, 31.83082137946489354, 11.00000000000000000 ) ) ;
#10894=ORIENTED_EDGE ( 'NONE', *, *, #8626, .T. ) ;
#10896=CARTESIAN_POINT ( 'NONE',  ( 3.607749162633204332, 7.931741834401772273, 10.63089969389957545 ) ) ;
#10902=ORIENTED_EDGE ( 'NONE', *, *, #4052, .F. ) ;
#10907=VERTEX_POINT ( 'NONE', #5688 ) ;
#10909=ADVANCED_FACE ( 'NONE', ( #31080 ), #18762, .T. ) ;
#10911=VECTOR ( 'NONE', #5596, 1000.000000000000227 ) ;
#10913=ORIENTED_EDGE ( 'NONE', *, *, #10706, .F. ) ;
#10914=EDGE_CURVE ( 'NONE', #14680, #14045, #23084, .T. ) ;
#10916=DIRECTION ( 'NONE',  ( -0.2079116908177663370, -0.9781476007338042455, 0.000000000000000000 ) ) ;
#10918=( NAMED_UNIT ( * ) PLANE_ANGLE_UNIT ( ) SI_UNIT ( $, .RADIAN. ) );
#10925=LINE ( 'NONE', #14364, #34416 ) ;
#10929=FACE_OUTER_BOUND ( 'NONE', #16627, .T. ) ;
#10935=DIRECTION ( 'NONE',  ( 0.000000000000000000, 0.000000000000000000, -1.000000000000000000 ) ) ;
#10936=AXIS2_PLACEMENT_3D ( 'NONE', #8600, #8405, #20802 ) ;
#10937=ORIENTED_EDGE ( 'NONE', *, *, #38336, .T. ) ;
#10939=LINE ( 'NONE', #14173, #5792 ) ;
#10951=DIRECTION ( 'NONE',  ( -0.9781476007338043566, 0.2079116908177657264, 0.000000000000000000 ) ) ;
#10955=LINE ( 'NONE', #14397, #5323 ) ;
#10956=ORIENTED_EDGE ( 'NONE', *, *, #14562, .T. ) ;
#10957=DIRECTION ( 'NONE',  ( -1.000000000000000000, 0.000000000000000000, 0.000000000000000000 ) ) ;
#10958=CARTESIAN_POINT ( 'NONE',  ( 8.954580980757247843, 11.02572744104254987, 11.00000000000000000 ) ) ;
#10959=ORIENTED_EDGE ( 'NONE', *, *, #36602, .T. ) ;
#10966=DIRECTION ( 'NONE',  ( -0.8660254037844425934, -0.4999999999999933942, -6.938893903907226800E-15 ) ) ;
#10967=EDGE_LOOP ( 'NONE', ( #28242, #37480, #11060, #12628 ) ) ;
#10970=CARTESIAN_POINT ( 'NONE',  ( 3.161220354320215975, 12.43736188311278212, 10.50000000000000000 ) ) ;
#10976=DIRECTION ( 'NONE',  ( 1.000000000000000000, 0.000000000000000000, 0.000000000000000000 ) ) ;
#10979=EDGE_LOOP ( 'NONE', ( #33742, #9786, #19776, #14110, #9005 ) ) ;
#10986=AXIS2_PLACEMENT_3D ( 'NONE', #931, #35811, #32570 ) ;
#10989=VECTOR ( 'NONE', #24310, 1000.000000000000000 ) ;
#10992=ADVANCED_FACE ( 'NONE', ( #35278 ), #4192, .T. ) ;
#10993=DIRECTION ( 'NONE',  ( -0.9945218953682745111, -0.1045284632676437703, 0.000000000000000000 ) ) ;
#10994=EDGE_CURVE ( 'NONE', #25787, #32523, #16570, .T. ) ;
#10995=ORIENTED_EDGE ( 'NONE', *, *, #7096, .F. ) ;
#10996=VERTEX_POINT ( 'NONE', #10290 ) ;
#10997=CIRCLE ( 'NONE', #7734, 0.4999999999999995559 ) ;
#11002=PLANE ( 'NONE',  #1416 ) ;
#11006=CARTESIAN_POINT ( 'NONE',  ( -3.610593701936590350, 31.83882289796395426, 10.50000000000000533 ) ) ;
#11008=VERTEX_POINT ( 'NONE', #32232 ) ;
#11010=CARTESIAN_POINT ( 'NONE',  ( 4.727507481117209309, 31.88885898370940453, 10.50000000000000000 ) ) ;
#11011=ORIENTED_EDGE ( 'NONE', *, *, #7121, .T. ) ;
#11014=EDGE_CURVE ( 'NONE', #7168, #22045, #10697, .T. ) ;
#11021=VECTOR ( 'NONE', #37889, 1000.000000000000114 ) ;
#11023=DIRECTION ( 'NONE',  ( 0.8660254037844377084, -0.5000000000000015543, -3.469446951953621683E-15 ) ) ;
#11024=EDGE_LOOP ( 'NONE', ( #15050, #25980, #31375, #10641 ) ) ;
#11025=CARTESIAN_POINT ( 'NONE',  ( -8.015823967414606344, 9.821249526829326726, 7.339470489435493405 ) ) ;
#11026=CIRCLE ( 'NONE', #23346, 0.5000000000000001110 ) ;
#11028=LINE ( 'NONE', #35805, #28160 ) ;
#11032=CARTESIAN_POINT ( 'NONE',  ( -12.49038105676665644, 14.13397459621567798, 11.00000000000000000 ) ) ;
#11035=ORIENTED_EDGE ( 'NONE', *, *, #10007, .T. ) ;
#11037=ORIENTED_EDGE ( 'NONE', *, *, #18989, .F. ) ;
#11043=ORIENTED_EDGE ( 'NONE', *, *, #21293, .T. ) ;
#11047=DIRECTION ( 'NONE',  ( 1.000000000000000000, 0.000000000000000000, 0.000000000000000000 ) ) ;
#11049=CARTESIAN_POINT ( 'NONE',  ( 8.118377661053324701, 10.47536095541698486, 9.000000000000001776 ) ) ;
#11050=VERTEX_POINT ( 'NONE', #1556 ) ;
#11053=CARTESIAN_POINT ( 'NONE',  ( 5.473344025737210572, 14.11593743010426394, 10.49999999999999822 ) ) ;
#11055=EDGE_LOOP ( 'NONE', ( #12796, #22524, #17992, #6716, #27587 ) ) ;
#11060=ORIENTED_EDGE ( 'NONE', *, *, #3147, .F. ) ;
#11064=EDGE_CURVE ( 'NONE', #39958, #20580, #38729, .T. ) ;
#11071=CARTESIAN_POINT ( 'NONE',  ( -13.46929972531958697, 26.35070966310183138, 7.499999999999994671 ) ) ;
#11073=DIRECTION ( 'NONE',  ( 0.000000000000000000, 0.000000000000000000, -1.000000000000000000 ) ) ;
#11074=CARTESIAN_POINT ( 'NONE',  ( -9.151574469205524309, 1.945227203041487218, 7.000000000000000000 ) ) ;
#11080=AXIS2_PLACEMENT_3D ( 'NONE', #34956, #14013, #13407 ) ;
#11082=LINE ( 'NONE', #33430, #15149 ) ;
#11085=ORIENTED_EDGE ( 'NONE', *, *, #20515, .T. ) ;
#11091=ORIENTED_EDGE ( 'NONE', *, *, #25743, .T. ) ;
#11092=CARTESIAN_POINT ( 'NONE',  ( -14.89501059309200137, 21.76138985984223595, 10.49999999999999822 ) ) ;
#11095=CARTESIAN_POINT ( 'NONE',  ( 8.238488885696289898, 24.65111619403943877, 9.000000000000001776 ) ) ;
#11101=ORIENTED_EDGE ( 'NONE', *, *, #33904, .T. ) ;
#11104=CARTESIAN_POINT ( 'NONE',  ( 13.63581098909226519, 27.45627467658428600, 7.000000000000000000 ) ) ;
#11106=DIRECTION ( 'NONE',  ( -0.9135454576426005335, 0.4067366430758009299, 0.000000000000000000 ) ) ;
#11112=VECTOR ( 'NONE', #36358, 1000.000000000000000 ) ;
#11119=CARTESIAN_POINT ( 'NONE',  ( 6.557822374958623968, 35.99981354310097004, 10.59344459855570619 ) ) ;
#11120=CYLINDRICAL_SURFACE ( 'NONE', #19030, 6.000000000000005329 ) ;
#11122=FACE_OUTER_BOUND ( 'NONE', #39072, .T. ) ;
#11123=CARTESIAN_POINT ( 'NONE',  ( -13.24038105676664046, 15.43301270189234486, 10.63089969389957545 ) ) ;
#11124=CARTESIAN_POINT ( 'NONE',  ( 14.36830325120613239, 20.48707633493483371, 7.000000000000000000 ) ) ;
#11126=EDGE_CURVE ( 'NONE', #35341, #6246, #30942, .T. ) ;
#11129=FACE_OUTER_BOUND ( 'NONE', #30436, .T. ) ;
#11132=DIRECTION ( 'NONE',  ( -0.000000000000000000, -0.000000000000000000, 1.000000000000000000 ) ) ;
#11135=AXIS2_PLACEMENT_3D ( 'NONE', #34528, #22722, #18889 ) ;
#11137=CARTESIAN_POINT ( 'NONE',  ( -14.06009009443818591, 27.59413131461144530, 10.76099332938163400 ) ) ;
#11139=CARTESIAN_POINT ( 'NONE',  ( -14.97283170755581061, 21.46414480565966798, 10.49999999999999822 ) ) ;
#11140=DIRECTION ( 'NONE',  ( -0.4067366430757888285, 0.9135454576426059736, 0.000000000000000000 ) ) ;
#11146=EDGE_LOOP ( 'NONE', ( #4276, #8949, #39370, #33080, #35088, #39282, #34136 ) ) ;
#11148=ORIENTED_EDGE ( 'NONE', *, *, #31759, .F. ) ;
#11150=CARTESIAN_POINT ( 'NONE',  ( 14.52509594610761745, 21.97885917798724265, 10.49999999999999822 ) ) ;
#11151=EDGE_LOOP ( 'NONE', ( #38782, #22273, #19195 ) ) ;
#11152=DIRECTION ( 'NONE',  ( -0.4067366430757884399, 0.9135454576426061957, 1.734723475976807410E-14 ) ) ;
#11153=CARTESIAN_POINT ( 'NONE',  ( 9.126688212160850355, 10.78884215935634749, 10.87262190629280667 ) ) ;
#11160=ORIENTED_EDGE ( 'NONE', *, *, #18532, .F. ) ;
#11161=VECTOR ( 'NONE', #18605, 1000.000000000000000 ) ;
#11163=VERTEX_POINT ( 'NONE', #30596 ) ;
#11164=LINE ( 'NONE', #14410, #33957 ) ;
#11167=CARTESIAN_POINT ( 'NONE',  ( 0.000000000000000000, 22.50000000000000355, 7.000000000000000000 ) ) ;
#11170=LINE ( 'NONE', #4670, #15859 ) ;
#11171=CARTESIAN_POINT ( 'NONE',  ( -1.000000000000000000, 37.00000000000000711, 10.49999999999999822 ) ) ;
#11173=EDGE_CURVE ( 'NONE', #32427, #40197, #10842, .T. ) ;
#11176=VERTEX_POINT ( 'NONE', #17614 ) ;
#11178=AXIS2_PLACEMENT_3D ( 'NONE', #17335, #29710, #32975 ) ;
#11179=CARTESIAN_POINT ( 'NONE',  ( -10.33795143809923367, 20.40792924032147226, 10.50000000000000000 ) ) ;
#11180=EDGE_CURVE ( 'NONE', #34496, #20580, #8225, .T. ) ;
#11183=LINE ( 'NONE', #23165, #26457 ) ;
#11187=AXIS2_PLACEMENT_3D ( 'NONE', #28679, #7546, #38230 ) ;
#11188=CARTESIAN_POINT ( 'NONE',  ( -15.00000000000000000, 22.50000000000000355, 7.000000000000000000 ) ) ;
#11189=ORIENTED_EDGE ( 'NONE', *, *, #19932, .F. ) ;
#11190=B_SPLINE_CURVE_WITH_KNOTS ( 'NONE', 3,
 ( #6462, #31652, #6656, #13360, #22496, #35102 ),
 .UNSPECIFIED., .F., .F.,
 ( 4, 2, 4 ),
 ( 0.000000000000000000, 0.4999999999999988898, 1.000000000000000000 ),
 .UNSPECIFIED. ) ;
#11191=ORIENTED_EDGE ( 'NONE', *, *, #14228, .T. ) ;
#11193=FACE_OUTER_BOUND ( 'NONE', #14604, .T. ) ;
#11195=VECTOR ( 'NONE', #6381, 1000.000000000000114 ) ;
#11200=CARTESIAN_POINT ( 'NONE',  ( 11.30412111481574655, 32.00546000420950321, 10.94611345180491035 ) ) ;
#11201=CARTESIAN_POINT ( 'NONE',  ( 9.892954722048896699, 20.95745441963929423, 10.50000000000000533 ) ) ;
#11202=CARTESIAN_POINT ( 'NONE',  ( -2.623829155769458410, 7.750987179268020277, 10.68306085400110739 ) ) ;
#11207=ORIENTED_EDGE ( 'NONE', *, *, #7603, .T. ) ;
#11210=ORIENTED_EDGE ( 'NONE', *, *, #1106, .T. ) ;
#11212=ADVANCED_FACE ( 'NONE', ( #2162 ), #39725, .T. ) ;
#11217=LINE ( 'NONE', #33563, #10315 ) ;
#11218=ORIENTED_EDGE ( 'NONE', *, *, #36845, .F. ) ;
#11219=DIRECTION ( 'NONE',  ( 0.5254827454987502922, -0.4731467892558335331, -0.7071067811865415775 ) ) ;
#11220=AXIS2_PLACEMENT_3D ( 'NONE', #12990, #611, #6886 ) ;
#11221=CARTESIAN_POINT ( 'NONE',  ( -7.852079885517520452, 9.718707764022953555, 7.203056206335834766 ) ) ;
#11223=DIRECTION ( 'NONE',  ( 0.000000000000000000, 0.000000000000000000, -1.000000000000000000 ) ) ;
#11227=CARTESIAN_POINT ( 'NONE',  ( -13.24038105676666710, 15.43301270189238394, 10.59344438985530878 ) ) ;
#11228=CARTESIAN_POINT ( 'NONE',  ( -9.356056665764024061, 26.06569820189715259, 10.49999999999999112 ) ) ;
#11232=ORIENTED_EDGE ( 'NONE', *, *, #38535, .F. ) ;
#11235=EDGE_CURVE ( 'NONE', #5911, #4096, #5001, .T. ) ;
#11238=ORIENTED_EDGE ( 'NONE', *, *, #19203, .T. ) ;
#11240=ORIENTED_EDGE ( 'NONE', *, *, #27021, .T. ) ;
#11245=CIRCLE ( 'NONE', #22236, 0.5000000000000004441 ) ;
#11250=VERTEX_POINT ( 'NONE', #39328 ) ;
#11252=CARTESIAN_POINT ( 'NONE',  ( -7.713869163866016621, 10.18146832927085121, 10.49999999999999822 ) ) ;
#11255=ORIENTED_EDGE ( 'NONE', *, *, #19815, .T. ) ;
#11258=AXIS2_PLACEMENT_3D ( 'NONE', #6893, #16050, #24996 ) ;
#11260=EDGE_CURVE ( 'NONE', #5091, #23135, #17412, .T. ) ;
#11264=AXIS2_PLACEMENT_3D ( 'NONE', #11478, #20426, #14320 ) ;
#11265=FACE_OUTER_BOUND ( 'NONE', #5379, .T. ) ;
#11269=EDGE_CURVE ( 'NONE', #39078, #34288, #32895, .T. ) ;
#11271=AXIS2_PLACEMENT_3D ( 'NONE', #20073, #13761, #1992 ) ;
#11272=DIRECTION ( 'NONE',  ( -0.7032331762534076436, 0.07391278520357413839, -0.7071067811865433539 ) ) ;
#11273=CARTESIAN_POINT ( 'NONE',  ( -10.49474413300070097, 21.89971208337388120, 10.00000000000000000 ) ) ;
#11274=DIRECTION ( 'NONE',  ( 0.5773502691896257311, -0.5773502691896217343, 0.5773502691896298389 ) ) ;
#11275=ORIENTED_EDGE ( 'NONE', *, *, #4816, .F. ) ;
#11277=DIRECTION ( 'NONE',  ( 0.000000000000000000, 0.000000000000000000, 1.000000000000000000 ) ) ;
#11280=FACE_OUTER_BOUND ( 'NONE', #5385, .T. ) ;
#11282=B_SPLINE_CURVE_WITH_KNOTS ( 'NONE', 3,
 ( #35360, #1432, #17691, #7920, #23765, #8120 ),
 .UNSPECIFIED., .F., .F.,
 ( 4, 2, 4 ),
 ( 0.000000000000000000, 0.5000000000000000000, 1.000000000000000000 ),
 .UNSPECIFIED. ) ;
#11284=DIRECTION ( 'NONE',  ( -0.000000000000000000, -0.000000000000000000, -1.000000000000000000 ) ) ;
#11285=EDGE_LOOP ( 'NONE', ( #14139, #39230, #3374 ) ) ;
#11286=VECTOR ( 'NONE', #34098, 1000.000000000000000 ) ;
#11288=ADVANCED_FACE ( 'NONE', ( #31573 ), #27930, .T. ) ;
#11294=VERTEX_POINT ( 'NONE', #25469 ) ;
#11295=LINE ( 'NONE', #20437, #26106 ) ;
#11296=ORIENTED_EDGE ( 'NONE', *, *, #24342, .F. ) ;
#11298=CARTESIAN_POINT ( 'NONE',  ( 11.44134295108989186, 15.31698729810772797, 10.00000000000000000 ) ) ;
#11302=VECTOR ( 'NONE', #20775, 1000.000000000000000 ) ;
#11307=DIRECTION ( 'NONE',  ( -0.2079116908177664480, -0.9781476007338042455, 0.000000000000000000 ) ) ;
#11308=DIRECTION ( 'NONE',  ( 0.000000000000000000, 0.000000000000000000, -1.000000000000000000 ) ) ;
#11309=CARTESIAN_POINT ( 'NONE',  ( -14.84160187385925589, 20.32586711127000711, 7.500000000000004441 ) ) ;
#11313=FACE_OUTER_BOUND ( 'NONE', #36772, .T. ) ;
#11317=DIRECTION ( 'NONE',  ( -0.8090169943749504489, -0.5877852522924689183, 0.000000000000000000 ) ) ;
#11320=VERTEX_POINT ( 'NONE', #3151 ) ;
#11322=CARTESIAN_POINT ( 'NONE',  ( 6.546529844545025512, 35.97445010452246805, 10.68306085400100791 ) ) ;
#11323=DIRECTION ( 'NONE',  ( 0.8660254037844431485, 0.4999999999999921174, 0.000000000000000000 ) ) ;
#11327=FACE_OUTER_BOUND ( 'NONE', #35999, .T. ) ;
#11328=DIRECTION ( 'NONE',  ( 1.000000000000000000, 0.000000000000000000, 0.000000000000000000 ) ) ;
#11329=CARTESIAN_POINT ( 'NONE',  ( 10.06946225350410984, 32.23940090176269990, 7.499999999999996447 ) ) ;
#11331=AXIS2_PLACEMENT_3D ( 'NONE', #2441, #21716, #24572 ) ;
#11333=CARTESIAN_POINT ( 'NONE',  ( -12.99377146717201192, 26.19620116591435277, 10.50000000000000000 ) ) ;
#11334=ORIENTED_EDGE ( 'NONE', *, *, #16593, .T. ) ;
#11336=CARTESIAN_POINT ( 'NONE',  ( -3.784955426773653375, 9.502919080911414795, 9.500000000000000000 ) ) ;
#11337=CARTESIAN_POINT ( 'NONE',  ( -1.000000000000000444, 37.04625217320466390, 10.49999999999999822 ) ) ;
#11339=EDGE_CURVE ( 'NONE', #24976, #13129, #6339, .T. ) ;
#11343=CARTESIAN_POINT ( 'NONE',  ( -0.5000000000000004441, 32.50000000000000000, 10.50000000000000000 ) ) ;
#11344=EDGE_CURVE ( 'NONE', #31717, #2452, #18988, .T. ) ;
#11345=AXIS2_PLACEMENT_3D ( 'NONE', #38080, #10055, #7399 ) ;
#11350=CYLINDRICAL_SURFACE ( 'NONE', #21879, 0.4999999999999998890 ) ;
#11351=ORIENTED_EDGE ( 'NONE', *, *, #7561, .T. ) ;
#11353=ORIENTED_EDGE ( 'NONE', *, *, #22386, .F. ) ;
#11354=CARTESIAN_POINT ( 'NONE',  ( 5.023113021171168313, 36.63452954033265030, 7.203056206335840095 ) ) ;
#11355=ORIENTED_EDGE ( 'NONE', *, *, #33008, .T. ) ;
#11357=CARTESIAN_POINT ( 'NONE',  ( 1.278175571583998194, 14.08178954835375940, 9.000000000000001776 ) ) ;
#11360=EDGE_CURVE ( 'NONE', #25659, #25600, #30099, .T. ) ;
#11361=ORIENTED_EDGE ( 'NONE', *, *, #17569, .T. ) ;
#11363=AXIS2_PLACEMENT_3D ( 'NONE', #1593, #7875, #17244 ) ;
#11364=EDGE_CURVE ( 'NONE', #20973, #16864, #106, .T. ) ;
#11366=CARTESIAN_POINT ( 'NONE',  ( 10.62305557349671403, 33.09035064698313278, 7.455686640544900712 ) ) ;
#11367=ORIENTED_EDGE ( 'NONE', *, *, #21444, .F. ) ;
#11369=DIRECTION ( 'NONE',  ( 0.000000000000000000, 0.000000000000000000, -1.000000000000000000 ) ) ;
#11370=AXIS2_PLACEMENT_3D ( 'NONE', #9071, #8267, #6011 ) ;
#11371=ADVANCED_FACE ( 'NONE', ( #19180 ), #16141, .T. ) ;
#11377=CARTESIAN_POINT ( 'NONE',  ( 10.16122020288883299, 33.53402030034401804, 7.000000000000000000 ) ) ;
#11381=DIRECTION ( 'NONE',  ( -0.8090169943749503378, -0.5877852522924691403, 0.000000000000000000 ) ) ;
#11385=EDGE_CURVE ( 'NONE', #17600, #35419, #18398, .T. ) ;
#11387=DIRECTION ( 'NONE',  ( 0.000000000000000000, 0.000000000000000000, 1.000000000000000000 ) ) ;
#11388=ADVANCED_FACE ( 'NONE', ( #21831 ), #12489, .T. ) ;
#11396=VECTOR ( 'NONE', #38912, 1000.000000000000000 ) ;
#11398=DIRECTION ( 'NONE',  ( 0.000000000000000000, 0.000000000000000000, 1.000000000000000000 ) ) ;
#11400=CARTESIAN_POINT ( 'NONE',  ( 0.5000000000000002220, 36.00000000000000711, 10.50000000000000000 ) ) ;
#11401=VERTEX_POINT ( 'NONE', #34235 ) ;
#11404=LINE ( 'NONE', #35585, #3809 ) ;
#11406=VERTEX_POINT ( 'NONE', #6386 ) ;
#11408=CARTESIAN_POINT ( 'NONE',  ( -5.459721035624959029, 35.99203088905950665, 10.99999999999999289 ) ) ;
#11409=ADVANCED_FACE ( 'NONE', ( #31181 ), #23157, .T. ) ;
#11410=VERTEX_POINT ( 'NONE', #15739 ) ;
#11414=ORIENTED_EDGE ( 'NONE', *, *, #3666, .F. ) ;
#11428=AXIS2_PLACEMENT_3D ( 'NONE', #13367, #19663, #32057 ) ;
#11431=CARTESIAN_POINT ( 'NONE',  ( -11.81630298851966288, 31.79381426990562787, 11.00000000000000000 ) ) ;
#11432=CARTESIAN_POINT ( 'NONE',  ( 2.525645716490519277, 8.212903943950919938, 11.00000000000000355 ) ) ;
#11433=ORIENTED_EDGE ( 'NONE', *, *, #28134, .T. ) ;
#11438=CARTESIAN_POINT ( 'NONE',  ( -14.18553059334566591, 26.06413323176255759, 10.49999999999999822 ) ) ;
#11440=VERTEX_POINT ( 'NONE', #7185 ) ;
#11442=VERTEX_POINT ( 'NONE', #3941 ) ;
#11446=CYLINDRICAL_SURFACE ( 'NONE', #2382, 0.4999999999999986122 ) ;
#11450=DIRECTION ( 'NONE',  ( -0.2079116908177663092, -0.9781476007338041345, 0.000000000000000000 ) ) ;
#11451=ORIENTED_EDGE ( 'NONE', *, *, #33431, .T. ) ;
#11454=LINE ( 'NONE', #27090, #12170 ) ;
#11456=ORIENTED_EDGE ( 'NONE', *, *, #12061, .T. ) ;
#11462=ORIENTED_EDGE ( 'NONE', *, *, #14579, .F. ) ;
#11464=DIRECTION ( 'NONE',  ( 1.000000000000000000, 0.000000000000000000, 0.000000000000000000 ) ) ;
#11465=DIRECTION ( 'NONE',  ( 0.7071067811865451302, 8.659560562354889717E-17, 0.7071067811865500152 ) ) ;
#11466=DIRECTION ( 'NONE',  ( -1.000000000000000000, 0.000000000000000000, 0.000000000000000000 ) ) ;
#11468=DIRECTION ( 'NONE',  ( -0.000000000000000000, -0.000000000000000000, -1.000000000000000000 ) ) ;
#11471=LINE ( 'NONE', #24257, #29547 ) ;
#11472=VERTEX_POINT ( 'NONE', #19380 ) ;
#11474=CARTESIAN_POINT ( 'NONE',  ( -10.47804177580193041, 33.28010392086039815, 10.49999999999999822 ) ) ;
#11478=CARTESIAN_POINT ( 'NONE',  ( -12.16658951415318768, 37.80625835076882879, 10.00000000000000000 ) ) ;
#11482=VERTEX_POINT ( 'NONE', #16545 ) ;
#11484=AXIS2_PLACEMENT_3D ( 'NONE', #37663, #10637, #7579 ) ;
#11486=EDGE_CURVE ( 'NONE', #2306, #13272, #1506, .T. ) ;
#11487=CARTESIAN_POINT ( 'NONE',  ( -7.659620408498105881, 26.92228390473685096, 9.000000000000001776 ) ) ;
#11489=EDGE_LOOP ( 'NONE', ( #9232, #19628, #4016, #39870 ) ) ;
#11491=EDGE_LOOP ( 'NONE', ( #27926, #8904, #39932, #33752, #32648, #17052, #19773 ) ) ;
#11493=DIRECTION ( 'NONE',  ( -0.000000000000000000, -0.000000000000000000, -1.000000000000000000 ) ) ;
#11495=CARTESIAN_POINT ( 'NONE',  ( 3.914034194965609892, 30.06176806842420035, 9.000000000000001776 ) ) ;
#11500=EDGE_CURVE ( 'NONE', #11836, #14093, #25673, .T. ) ;
#11505=EDGE_CURVE ( 'NONE', #38413, #8399, #10445, .T. ) ;
#11506=DIRECTION ( 'NONE',  ( 1.000000000000000000, 0.000000000000000000, 0.000000000000000000 ) ) ;
#11507=VERTEX_POINT ( 'NONE', #38070 ) ;
#11516=ORIENTED_EDGE ( 'NONE', *, *, #37483, .T. ) ;
#11522=CARTESIAN_POINT ( 'NONE',  ( -13.63581098909220479, 27.45627467658446008, 11.00000000000000000 ) ) ;
#11525=DIRECTION ( 'NONE',  ( -0.9510565162951507556, 0.3090169943749560000, 0.000000000000000000 ) ) ;
#11526=CARTESIAN_POINT ( 'NONE',  ( 10.73859285986296541, 31.49625607628530588, 9.500000000000000000 ) ) ;
#11532=VERTEX_POINT ( 'NONE', #35226 ) ;
#11534=CARTESIAN_POINT ( 'NONE',  ( -8.118377661053488126, 10.47536095541708967, 7.000000000000000000 ) ) ;
#11535=CARTESIAN_POINT ( 'NONE',  ( -13.63581098909220479, 27.45627467658446008, 10.99999999999999289 ) ) ;
#11539=CARTESIAN_POINT ( 'NONE',  ( 12.30736835487432757, 14.81698729810772441, 7.000000000000000000 ) ) ;
#11541=DIRECTION ( 'NONE',  ( 0.2079116908177656708, 0.9781476007338043566, -0.000000000000000000 ) ) ;
#11542=AXIS2_PLACEMENT_3D ( 'NONE', #3450, #21932, #15646 ) ;
#11543=CIRCLE ( 'NONE', #39429, 0.5000000000000004441 ) ;
#11548=DIRECTION ( 'NONE',  ( 0.000000000000000000, 0.000000000000000000, 1.000000000000000000 ) ) ;
#11551=AXIS2_PLACEMENT_3D ( 'NONE', #28840, #1018, #36542 ) ;
#11553=VECTOR ( 'NONE', #2954, 1000.000000000000114 ) ;
#11555=VERTEX_POINT ( 'NONE', #7386 ) ;
#11557=CARTESIAN_POINT ( 'NONE',  ( 9.415016184005738253, 11.18446770392332468, 10.49999999999999822 ) ) ;
#11558=EDGE_LOOP ( 'NONE', ( #16770, #4256, #11688, #12078 ) ) ;
#11563=CARTESIAN_POINT ( 'NONE',  ( -13.46929972531958875, 26.35070966310182783, 9.500000000000000000 ) ) ;
#11564=VERTEX_POINT ( 'NONE', #7796 ) ;
#11565=EDGE_CURVE ( 'NONE', #29202, #35666, #5667, .T. ) ;
#11566=CARTESIAN_POINT ( 'NONE',  ( 2.036571916123614656, 8.108948098542045457, 9.500000000000000000 ) ) ;
#11568=CIRCLE ( 'NONE', #27800, 0.4999999999999995559 ) ;
#11569=AXIS2_PLACEMENT_3D ( 'NONE', #28280, #37027, #18155 ) ;
#11570=PLANE ( 'NONE',  #8442 ) ;
#11571=ORIENTED_EDGE ( 'NONE', *, *, #7684, .F. ) ;
#11573=CARTESIAN_POINT ( 'NONE',  ( -1.838889047819898037, 31.15129278236396360, 9.000000000000001776 ) ) ;
#11576=CIRCLE ( 'NONE', #32347, 0.4999999999999999445 ) ;
#11578=ORIENTED_EDGE ( 'NONE', *, *, #4408, .T. ) ;
#11583=CARTESIAN_POINT ( 'NONE',  ( 6.576253646258392926, 14.29921418520925869, 10.50000000000000000 ) ) ;
#11584=CARTESIAN_POINT ( 'NONE',  ( 9.665073660139013256, 25.11464168560187460, 10.00000000000000000 ) ) ;
#11591=DIRECTION ( 'NONE',  ( 1.000000000000000000, 0.000000000000000000, 0.000000000000000000 ) ) ;
#11592=VERTEX_POINT ( 'NONE', #20605 ) ;
#11593=ORIENTED_EDGE ( 'NONE', *, *, #4387, .T. ) ;
#11596=CARTESIAN_POINT ( 'NONE',  ( 12.19971670159632637, 4.637739668175409058, 7.000000000000000000 ) ) ;
#11597=CARTESIAN_POINT ( 'NONE',  ( -12.48446084878477436, 14.34248059624584926, 10.49999999999999822 ) ) ;
#11599=AXIS2_PLACEMENT_3D ( 'NONE', #13973, #38151, #13767 ) ;
#11601=CARTESIAN_POINT ( 'NONE',  ( -11.80736835487443592, 13.95096189432345213, 7.000000000000000000 ) ) ;
#11602=ORIENTED_EDGE ( 'NONE', *, *, #15225, .T. ) ;
#11604=DIRECTION ( 'NONE',  ( 1.000000000000000000, 0.000000000000000000, 0.000000000000000000 ) ) ;
#11605=CARTESIAN_POINT ( 'NONE',  ( -2.606860170653613640, 7.830819977571337631, 10.82238861112329609 ) ) ;
#11609=CARTESIAN_POINT ( 'NONE',  ( -14.07088901726633345, 27.73527618063616984, 10.49999999999999645 ) ) ;
#11610=ORIENTED_EDGE ( 'NONE', *, *, #12965, .T. ) ;
#11615=CARTESIAN_POINT ( 'NONE',  ( 7.766013557953383106, 28.81973365084986938, 10.50000000000000178 ) ) ;
#11617=DIRECTION ( 'NONE',  ( -0.000000000000000000, -0.000000000000000000, -1.000000000000000000 ) ) ;
#11622=FACE_OUTER_BOUND ( 'NONE', #31609, .T. ) ;
#11623=CARTESIAN_POINT ( 'NONE',  ( 2.256323172317815207, 14.28970123917151192, 7.000000000000000000 ) ) ;
#11624=AXIS2_PLACEMENT_3D ( 'NONE', #31805, #25310, #7771 ) ;
#11626=CIRCLE ( 'NONE', #18127, 0.5000000000000004441 ) ;
#11627=DIRECTION ( 'NONE',  ( -0.2079116908177664480, -0.9781476007338042455, 0.000000000000000000 ) ) ;
#11631=TOROIDAL_SURFACE ( 'NONE', #19389, 1.000000000000000000, 0.5000000000000000000 ) ;
#11632=LINE ( 'NONE', #17738, #15717 ) ;
#11633=LINE ( 'NONE', #2090, #9680 ) ;
#11634=ORIENTED_EDGE ( 'NONE', *, *, #28957, .F. ) ;
#11635=ADVANCED_FACE ( 'NONE', ( #26887 ), #39675, .T. ) ;
#11637=ORIENTED_EDGE ( 'NONE', *, *, #11385, .T. ) ;
#11640=EDGE_CURVE ( 'NONE', #13994, #490, #11454, .T. ) ;
#11643=EDGE_LOOP ( 'NONE', ( #38325, #24303, #20934, #32421 ) ) ;
#11645=ORIENTED_EDGE ( 'NONE', *, *, #10761, .F. ) ;
#11647=CARTESIAN_POINT ( 'NONE',  ( -11.11016527260153630, 31.83082137946488643, 7.000000000000000000 ) ) ;
#11649=CARTESIAN_POINT ( 'NONE',  ( -4.524139159579195102, 31.43208625488816566, 10.50000000000000888 ) ) ;
#11650=ORIENTED_EDGE ( 'NONE', *, *, #36068, .T. ) ;
#11657=DIRECTION ( 'NONE',  ( 1.000000000000000000, 0.000000000000000000, 0.000000000000000000 ) ) ;
#11661=VERTEX_POINT ( 'NONE', #39480 ) ;
#11665=ORIENTED_EDGE ( 'NONE', *, *, #35362, .T. ) ;
#11667=DIRECTION ( 'NONE',  ( -1.000000000000000000, -1.224646799147351235E-16, 0.000000000000000000 ) ) ;
#11672=CARTESIAN_POINT ( 'NONE',  ( 10.29511041547406691, 24.79362192464177639, 11.00000000000000000 ) ) ;
#11675=CARTESIAN_POINT ( 'NONE',  ( 14.09933648065468503, 26.02968990214155198, 10.50000000000000533 ) ) ;
#11685=EDGE_CURVE ( 'NONE', #29068, #4691, #32919, .T. ) ;
#11686=CARTESIAN_POINT ( 'NONE',  ( -8.910254037844424602, 17.93301270189230578, 10.50000000000000178 ) ) ;
#11688=ORIENTED_EDGE ( 'NONE', *, *, #13748, .F. ) ;
#11689=DIRECTION ( 'NONE',  ( -1.000000000000000000, 0.000000000000000000, 0.000000000000000000 ) ) ;
#11690=VECTOR ( 'NONE', #20469, 999.9999999999998863 ) ;
#11691=EDGE_LOOP ( 'NONE', ( #35881, #28676, #14436 ) ) ;
#11693=CARTESIAN_POINT ( 'NONE',  ( 14.97277451176449325, 21.48159783397873923, 10.49999999999999822 ) ) ;
#11700=ORIENTED_EDGE ( 'NONE', *, *, #2346, .F. ) ;
#11703=DIRECTION ( 'NONE',  ( 0.000000000000000000, 0.000000000000000000, 1.000000000000000000 ) ) ;
#11704=CARTESIAN_POINT ( 'NONE',  ( 0.000000000000000000, 22.50000000000000355, 0.000000000000000000 ) ) ;
#11705=ORIENTED_EDGE ( 'NONE', *, *, #30256, .F. ) ;
#11708=VECTOR ( 'NONE', #11369, 1000.000000000000000 ) ;
#11709=CARTESIAN_POINT ( 'NONE',  ( -9.734896950324548826, 32.61097331450152836, 10.50000000000000000 ) ) ;
#11711=DIRECTION ( 'NONE',  ( -0.000000000000000000, -0.000000000000000000, -1.000000000000000000 ) ) ;
#11712=CARTESIAN_POINT ( 'NONE',  ( -7.111215932167764819, 17.81698729810783988, 9.000000000000001776 ) ) ;
#11713=ADVANCED_FACE ( 'NONE', ( #6728 ), #1119, .T. ) ;
#11714=VERTEX_POINT ( 'NONE', #12244 ) ;
#11715=EDGE_CURVE ( 'NONE', #32514, #15350, #21389, .T. ) ;
#11717=CARTESIAN_POINT ( 'NONE',  ( 14.97435279638159322, 21.61966441463743749, 7.485646746502383486 ) ) ;
#11718=CARTESIAN_POINT ( 'NONE',  ( 6.856875760695868571, 35.58019112794455907, 10.49999999999999822 ) ) ;
#11719=FACE_OUTER_BOUND ( 'NONE', #7259, .T. ) ;
#11721=FACE_OUTER_BOUND ( 'NONE', #16930, .T. ) ;
#11723=EDGE_CURVE ( 'NONE', #22206, #10321, #29690, .T. ) ;
#11727=CARTESIAN_POINT ( 'NONE',  ( -5.440908595777636414, 35.94977745735568675, 11.00000000000000000 ) ) ;
#11729=CARTESIAN_POINT ( 'NONE',  ( -10.39021566973305788, 20.90519018800561213, 10.00000000000000000 ) ) ;
#11730=ORIENTED_EDGE ( 'NONE', *, *, #6012, .T. ) ;
#11731=AXIS2_PLACEMENT_3D ( 'NONE', #31343, #31940, #21796 ) ;
#11734=CARTESIAN_POINT ( 'NONE',  ( -13.86243997625759583, 27.52991089825177795, 10.94387467463492136 ) ) ;
#11737=CARTESIAN_POINT ( 'NONE',  ( -3.503793317224518145, 8.420815634768723967, 7.000000000000000000 ) ) ;
#11739=ORIENTED_EDGE ( 'NONE', *, *, #6521, .F. ) ;
#11747=EDGE_CURVE ( 'NONE', #16315, #22657, #34384, .T. ) ;
#11748=AXIS2_PLACEMENT_3D ( 'NONE', #32311, #7717, #35759 ) ;
#11750=ORIENTED_EDGE ( 'NONE', *, *, #8221, .T. ) ;
#11752=ORIENTED_EDGE ( 'NONE', *, *, #21935, .T. ) ;
#11753=CARTESIAN_POINT ( 'NONE',  ( -12.80736835487442349, 15.68301270189233954, 7.000000000000000000 ) ) ;
#11757=EDGE_CURVE ( 'NONE', #19499, #20763, #29017, .T. ) ;
#11758=VERTEX_POINT ( 'NONE', #37630 ) ;
#11760=CARTESIAN_POINT ( 'NONE',  ( 10.33787318040696057, 33.36945112946456504, 7.203056206335834766 ) ) ;
#11761=EDGE_LOOP ( 'NONE', ( #39866, #37156, #6134, #34582 ) ) ;
#11762=DIRECTION ( 'NONE',  ( -0.8090169943749423442, 0.5877852522924800205, 0.000000000000000000 ) ) ;
#11763=DIRECTION ( 'NONE',  ( -0.7071067811865526798, 0.000000000000000000, -0.7071067811865424657 ) ) ;
#11765=ORIENTED_EDGE ( 'NONE', *, *, #33709, .F. ) ;
#11766=EDGE_CURVE ( 'NONE', #6428, #19542, #18746, .T. ) ;
#11770=EDGE_CURVE ( 'NONE', #7975, #2021, #31530, .T. ) ;
#11771=CARTESIAN_POINT ( 'NONE',  ( 1.000000000000000000, 37.00000000000000711, 7.500000000000000888 ) ) ;
#11775=ORIENTED_EDGE ( 'NONE', *, *, #20332, .F. ) ;
#11777=FACE_OUTER_BOUND ( 'NONE', #1465, .T. ) ;
#11778=CARTESIAN_POINT ( 'NONE',  ( -14.72984284853662729, 19.66343513167324630, 7.102637441331452806 ) ) ;
#11786=AXIS2_PLACEMENT_3D ( 'NONE', #30461, #36751, #15009 ) ;
#11788=DIRECTION ( 'NONE',  ( -0.3090169943749450643, 0.9510565162951543083, 0.000000000000000000 ) ) ;
#11790=ORIENTED_EDGE ( 'NONE', *, *, #7907, .T. ) ;
#11793=DIRECTION ( 'NONE',  ( -0.8660254037844432595, -0.4999999999999920064, 0.000000000000000000 ) ) ;
#11794=DIRECTION ( 'NONE',  ( -0.9510565162951503115, 0.3090169943749573322, 0.000000000000000000 ) ) ;
#11795=CARTESIAN_POINT ( 'NONE',  ( -9.417813166173889527, 10.93662330136618444, 10.49999999999999822 ) ) ;
#11798=DIRECTION ( 'NONE',  ( 1.000000000000000000, 3.469446951953568829E-15, 0.000000000000000000 ) ) ;
#11800=CARTESIAN_POINT ( 'NONE',  ( -3.813962023474481544, 32.29559562678526419, 10.50000000000000000 ) ) ;
#11801=VERTEX_POINT ( 'NONE', #27484 ) ;
#11803=CARTESIAN_POINT ( 'NONE',  ( -9.427394962683591118, 11.06314620782489833, 10.49999999999999822 ) ) ;
#11804=ORIENTED_EDGE ( 'NONE', *, *, #16513, .F. ) ;
#11807=ORIENTED_EDGE ( 'NONE', *, *, #39545, .T. ) ;
#11810=CARTESIAN_POINT ( 'NONE',  ( 13.36830325120611995, 20.48707633493483371, 7.000000000000000000 ) ) ;
#11811=EDGE_CURVE ( 'NONE', #32024, #30975, #15496, .T. ) ;
#11815=DIRECTION ( 'NONE',  ( 0.000000000000000000, 0.000000000000000000, 1.000000000000000000 ) ) ;
#11816=DIRECTION ( 'NONE',  ( 0.000000000000000000, 0.000000000000000000, 1.000000000000000000 ) ) ;
#11818=DIRECTION ( 'NONE',  ( -0.2185080122244276168, -0.6724985119639504960, 0.7071067811865486830 ) ) ;
#11820=VECTOR ( 'NONE', #26742, 1000.000000000000000 ) ;
#11823=CARTESIAN_POINT ( 'NONE',  ( -12.84742388243067168, 15.65988663227498456, 11.00000000000000000 ) ) ;
#11825=ORIENTED_EDGE ( 'NONE', *, *, #36882, .T. ) ;
#11827=ORIENTED_EDGE ( 'NONE', *, *, #8152, .T. ) ;
#11829=CIRCLE ( 'NONE', #13765, 6.000000000000003553 ) ;
#11836=VERTEX_POINT ( 'NONE', #30936 ) ;
#11841=ADVANCED_FACE ( 'NONE', ( #24436 ), #17352, .T. ) ;
#11842=EDGE_LOOP ( 'NONE', ( #9186, #27641, #5574, #35284, #12978 ) ) ;
#11846=CARTESIAN_POINT ( 'NONE',  ( 0.000000000000000000, 22.50000000000000355, 7.000000000000000000 ) ) ;
#11847=ORIENTED_EDGE ( 'NONE', *, *, #34431, .F. ) ;
#11851=ORIENTED_EDGE ( 'NONE', *, *, #31236, .T. ) ;
#11856=ORIENTED_EDGE ( 'NONE', *, *, #3347, .T. ) ;
#11857=AXIS2_PLACEMENT_3D ( 'NONE', #20759, #35790, #13843 ) ;
#11859=DIRECTION ( 'NONE',  ( 0.05233595624294447302, 0.9986295347545738332, 0.000000000000000000 ) ) ;
#11861=DIRECTION ( 'NONE',  ( -0.8660254037844433705, -0.4999999999999918399, -0.000000000000000000 ) ) ;
#11862=VECTOR ( 'NONE', #11450, 1000.000000000000114 ) ;
#11865=CYLINDRICAL_SURFACE ( 'NONE', #35069, 0.5000000000000015543 ) ;
#11866=EDGE_CURVE ( 'NONE', #6906, #31457, #37231, .T. ) ;
#11867=CARTESIAN_POINT ( 'NONE',  ( -11.68377382812826681, 31.90739031292463679, 7.426391444473273928 ) ) ;
#11871=DIRECTION ( 'NONE',  ( 0.2079116908177533751, -0.9781476007338067991, 0.000000000000000000 ) ) ;
#11874=PLANE ( 'NONE',  #7948 ) ;
#11877=ORIENTED_EDGE ( 'NONE', *, *, #37483, .F. ) ;
#11884=DIRECTION ( 'NONE',  ( -1.000000000000000000, 0.000000000000000000, 0.000000000000000000 ) ) ;
#11885=VERTEX_POINT ( 'NONE', #5945 ) ;
#11888=EDGE_CURVE ( 'NONE', #34284, #19377, #30333, .T. ) ;
#11890=CARTESIAN_POINT ( 'NONE',  ( 8.927394655428267711, 11.06314620770944757, 11.00000000000000000 ) ) ;
#11892=VECTOR ( 'NONE', #31691, 1000.000000000000114 ) ;
#11895=DIRECTION ( 'NONE',  ( -0.000000000000000000, -0.000000000000000000, -1.000000000000000000 ) ) ;
#11899=FACE_OUTER_BOUND ( 'NONE', #31193, .T. ) ;
#11902=EDGE_LOOP ( 'NONE', ( #3787, #3404, #32805, #24027 ) ) ;
#11906=CARTESIAN_POINT ( 'NONE',  ( -5.034171952701847808, 35.03623199971306690, 7.000000000000000000 ) ) ;
#11908=CARTESIAN_POINT ( 'NONE',  ( -10.79456899466765840, 1.678572790138225468, 10.00000000000000000 ) ) ;
#11911=CARTESIAN_POINT ( 'NONE',  ( 9.911438049897887126, 11.24107483890952075, 7.000000000000000000 ) ) ;
#11912=EDGE_CURVE ( 'NONE', #1084, #2141, #37425, .T. ) ;
#11913=( GEOMETRIC_REPRESENTATION_CONTEXT ( 3 ) GLOBAL_UNCERTAINTY_ASSIGNED_CONTEXT ( ( #16904 ) ) GLOBAL_UNIT_ASSIGNED_CONTEXT ( ( #13606, #19500, #32516 ) ) REPRESENTATION_CONTEXT ( 'NONE', 'WORKASPACE' ) );
#11914=ORIENTED_EDGE ( 'NONE', *, *, #33173, .T. ) ;
#11916=DIRECTION ( 'NONE',  ( -0.000000000000000000, -0.000000000000000000, -1.000000000000000000 ) ) ;
#11917=LINE ( 'NONE', #21259, #18405 ) ;
#11919=CARTESIAN_POINT ( 'NONE',  ( 8.910254037844364206, 17.93301270189218499, 10.50000000000000000 ) ) ;
#11920=CARTESIAN_POINT ( 'NONE',  ( 2.568190708544436429, 12.82247983807081226, 10.50000000000000000 ) ) ;
#11921=B_SPLINE_CURVE_WITH_KNOTS ( 'NONE', 3,
 ( #31199, #22439, #6214, #6796 ),
 .UNSPECIFIED., .F., .F.,
 ( 4, 4 ),
 ( 0.000000000000000000, 1.000000000000000000 ),
 .UNSPECIFIED. ) ;
#11922=CARTESIAN_POINT ( 'NONE',  ( -10.72918489117944674, 32.98258515686310943, 7.500000000000004441 ) ) ;
#11924=DIRECTION ( 'NONE',  ( -1.000000000000000000, 0.000000000000000000, 0.000000000000000000 ) ) ;
#11925=DIRECTION ( 'NONE',  ( 0.000000000000000000, 0.000000000000000000, 1.000000000000000000 ) ) ;
#11927=CARTESIAN_POINT ( 'NONE',  ( 9.911438049897887126, 11.24107483890952075, 7.000000000000000000 ) ) ;
#11928=EDGE_LOOP ( 'NONE', ( #31123, #8584, #25941 ) ) ;
#11930=CARTESIAN_POINT ( 'NONE',  ( -5.187504188494229673, 36.60991850771488032, 10.49999999999999822 ) ) ;
#11932=CARTESIAN_POINT ( 'NONE',  ( -13.95827473762437165, 27.56104949980369412, 10.87262190629278535 ) ) ;
#11937=ORIENTED_EDGE ( 'NONE', *, *, #16154, .T. ) ;
#11945=CARTESIAN_POINT ( 'NONE',  ( 8.816778784387034662, 10.36474508437574471, 7.000000000000000000 ) ) ;
#11946=EDGE_CURVE ( 'NONE', #20669, #15620, #26712, .T. ) ;
#11950=VECTOR ( 'NONE', #16813, 1000.000000000000000 ) ;
#11953=DIRECTION ( 'NONE',  ( 1.000000000000000000, 0.000000000000000000, 0.000000000000000000 ) ) ;
#11954=FACE_OUTER_BOUND ( 'NONE', #35016, .T. ) ;
#11957=CIRCLE ( 'NONE', #17165, 0.4999999999999999445 ) ;
#11958=ORIENTED_EDGE ( 'NONE', *, *, #34357, .F. ) ;
#11959=DIRECTION ( 'NONE',  ( 0.000000000000000000, 0.000000000000000000, 1.000000000000000000 ) ) ;
#11960=VERTEX_POINT ( 'NONE', #28675 ) ;
#11961=CARTESIAN_POINT ( 'NONE',  ( 8.927394655428276593, 11.06314620770945290, 7.000000000000000000 ) ) ;
#11963=CIRCLE ( 'NONE', #22334, 1.000000000000002665 ) ;
#11967=CARTESIAN_POINT ( 'NONE',  ( -3.829842517469123298, 8.490119531707978950, 10.66666666666666785 ) ) ;
#11968=FACE_OUTER_BOUND ( 'NONE', #16392, .T. ) ;
#11974=ORIENTED_EDGE ( 'NONE', *, *, #27882, .F. ) ;
#11976=CARTESIAN_POINT ( 'NONE',  ( 14.31603901957230462, 19.98981538725069740, 7.500000000000010658 ) ) ;
#11979=CARTESIAN_POINT ( 'NONE',  ( 3.784955426773477072, 9.502919080911359728, 9.500000000000000000 ) ) ;
#11983=EDGE_CURVE ( 'NONE', #26378, #26489, #16703, .T. ) ;
#11984=CARTESIAN_POINT ( 'NONE',  ( -0.4999999999999998890, 37.00000000000000711, 11.00000000000000000 ) ) ;
#11986=ORIENTED_EDGE ( 'NONE', *, *, #35923, .T. ) ;
#11988=CARTESIAN_POINT ( 'NONE',  ( -14.44622163125246850, 19.97613264340537143, 10.49999999999999645 ) ) ;
#11990=CIRCLE ( 'NONE', #25583, 6.000000000000008882 ) ;
#11991=DIRECTION ( 'NONE',  ( -0.1045284632676437703, 0.9945218953682745111, 0.000000000000000000 ) ) ;
#11992=ORIENTED_EDGE ( 'NONE', *, *, #30112, .T. ) ;
#11994=EDGE_CURVE ( 'NONE', #9244, #24567, #28476, .T. ) ;
#11995=FACE_OUTER_BOUND ( 'NONE', #32202, .T. ) ;
#11996=DIRECTION ( 'NONE',  ( -0.000000000000000000, -0.000000000000000000, 1.000000000000000000 ) ) ;
#11997=EDGE_CURVE ( 'NONE', #22687, #7930, #38627, .T. ) ;
#11998=ORIENTED_EDGE ( 'NONE', *, *, #22309, .F. ) ;
#11999=AXIS2_PLACEMENT_3D ( 'NONE', #12125, #15370, #30014 ) ;
#12001=DIRECTION ( 'NONE',  ( -1.000000000000000000, 0.000000000000000000, 0.000000000000000000 ) ) ;
#12005=ORIENTED_EDGE ( 'NONE', *, *, #24548, .T. ) ;
#12008=LINE ( 'NONE', #36593, #4621 ) ;
#12010=DIRECTION ( 'NONE',  ( 1.000000000000000000, 0.000000000000000000, 0.000000000000000000 ) ) ;
#12011=VERTEX_POINT ( 'NONE', #19532 ) ;
#12013=ADVANCED_FACE ( 'NONE', ( #13433 ), #23193, .T. ) ;
#12015=EDGE_CURVE ( 'NONE', #4321, #14003, #10801, .T. ) ;
#12016=VECTOR ( 'NONE', #38355, 999.9999999999998863 ) ;
#12018=LINE ( 'NONE', #24206, #20408 ) ;
#12019=CARTESIAN_POINT ( 'NONE',  ( -3.713592597587352717, 7.966960743906856379, 7.499999999999997335 ) ) ;
#12021=AXIS2_PLACEMENT_3D ( 'NONE', #39900, #30577, #27709 ) ;
#12023=FACE_OUTER_BOUND ( 'NONE', #10094, .T. ) ;
#12024=ORIENTED_EDGE ( 'NONE', *, *, #36372, .F. ) ;
#12025=ORIENTED_EDGE ( 'NONE', *, *, #24746, .T. ) ;
#12026=AXIS2_PLACEMENT_3D ( 'NONE', #36849, #21209, #33619 ) ;
#12028=CIRCLE ( 'NONE', #6822, 0.5000000000000002220 ) ;
#12031=CARTESIAN_POINT ( 'NONE',  ( -3.781037291632698416, 7.996959361763665619, 10.49999999999999822 ) ) ;
#12035=CARTESIAN_POINT ( 'NONE',  ( -6.557822374958138134, 35.99981354310120452, 10.49999999999999822 ) ) ;
#12037=EDGE_CURVE ( 'NONE', #13902, #35341, #18044, .T. ) ;
#12043=ORIENTED_EDGE ( 'NONE', *, *, #3219, .T. ) ;
#12045=CARTESIAN_POINT ( 'NONE',  ( -12.80736835487442349, 15.68301270189233954, 7.000000000000000000 ) ) ;
#12047=ORIENTED_EDGE ( 'NONE', *, *, #7492, .T. ) ;
#12052=ORIENTED_EDGE ( 'NONE', *, *, #2319, .T. ) ;
#12056=DIRECTION ( 'NONE',  ( -0.000000000000000000, -0.000000000000000000, 1.000000000000000000 ) ) ;
#12058=CIRCLE ( 'NONE', #34763, 0.9999999999999998890 ) ;
#12061=EDGE_CURVE ( 'NONE', #18383, #16182, #32547, .T. ) ;
#12066=FACE_OUTER_BOUND ( 'NONE', #26831, .T. ) ;
#12067=DIRECTION ( 'NONE',  ( -0.000000000000000000, -0.000000000000000000, -1.000000000000000000 ) ) ;
#12070=DIRECTION ( 'NONE',  ( 0.000000000000000000, -0.6216356077939705349, -0.7833065626704661666 ) ) ;
#12076=CARTESIAN_POINT ( 'NONE',  ( 12.74038105676654453, 14.56698729810772264, 10.49999999999999822 ) ) ;
#12078=ORIENTED_EDGE ( 'NONE', *, *, #12965, .F. ) ;
#12080=VERTEX_POINT ( 'NONE', #34985 ) ;
#12081=AXIS2_PLACEMENT_3D ( 'NONE', #16277, #31518, #6520 ) ;
#12083=DIRECTION ( 'NONE',  ( -0.000000000000000000, -0.000000000000000000, -1.000000000000000000 ) ) ;
#12087=AXIS2_PLACEMENT_3D ( 'NONE', #11095, #2354, #1752 ) ;
#12090=CARTESIAN_POINT ( 'NONE',  ( -14.92615392307458144, 21.72537115092790216, 10.49999999999999822 ) ) ;
#12092=VERTEX_POINT ( 'NONE', #10598 ) ;
#12093=ADVANCED_FACE ( 'NONE', ( #16091 ), #26026, .T. ) ;
#12095=AXIS2_PLACEMENT_3D ( 'NONE', #19411, #22652, #34267 ) ;
#12097=EDGE_CURVE ( 'NONE', #3986, #38536, #22372, .T. ) ;
#12098=DIRECTION ( 'NONE',  ( 0.000000000000000000, 0.000000000000000000, 1.000000000000000000 ) ) ;
#12099=CARTESIAN_POINT ( 'NONE',  ( -13.94482798346716201, 26.50521816028930999, 7.000000000000000000 ) ) ;
#12100=ORIENTED_EDGE ( 'NONE', *, *, #33127, .T. ) ;
#12104=DIRECTION ( 'NONE',  ( 1.000000000000000000, 0.000000000000000000, 0.000000000000000000 ) ) ;
#12106=CARTESIAN_POINT ( 'NONE',  ( -14.47283171447380035, 21.48159823030330884, 7.000000000000000000 ) ) ;
#12107=DIRECTION ( 'NONE',  ( 0.000000000000000000, 0.000000000000000000, 1.000000000000000000 ) ) ;
#12110=CARTESIAN_POINT ( 'NONE',  ( -5.490944681523147075, 34.83286367817517259, 7.000000000000000000 ) ) ;
#12112=EDGE_CURVE ( 'NONE', #33136, #17440, #13459, .T. ) ;
#12113=AXIS2_PLACEMENT_3D ( 'NONE', #36881, #8855, #32849 ) ;
#12114=AXIS2_PLACEMENT_3D ( 'NONE', #23019, #4538, #34614 ) ;
#12116=LINE ( 'NONE', #18617, #28771 ) ;
#12119=LINE ( 'NONE', #27555, #8485 ) ;
#12120=CARTESIAN_POINT ( 'NONE',  ( 5.362728154695969529, 13.41753630677055753, 11.00000000000000000 ) ) ;
#12121=CARTESIAN_POINT ( 'NONE',  ( -14.47283171447380390, 21.48159823030330884, 7.000000000000000000 ) ) ;
#12122=DIRECTION ( 'NONE',  ( -0.000000000000000000, -0.000000000000000000, -1.000000000000000000 ) ) ;
#12123=CARTESIAN_POINT ( 'NONE',  ( 14.09933648065468503, 26.02968990214155198, 10.50000000000000533 ) ) ;
#12125=CARTESIAN_POINT ( 'NONE',  ( -10.44103466624267185, 32.57396620494226624, 7.000000000000000000 ) ) ;
#12126=ORIENTED_EDGE ( 'NONE', *, *, #31722, .T. ) ;
#12128=DIRECTION ( 'NONE',  ( 0.9135454576426059736, 0.4067366430757888285, 0.000000000000000000 ) ) ;
#12135=CARTESIAN_POINT ( 'NONE',  ( -4.003793318659595535, 8.455722206104626437, 10.49999999999999822 ) ) ;
#12137=EDGE_CURVE ( 'NONE', #34496, #34284, #1455, .T. ) ;
#12142=ADVANCED_FACE ( 'NONE', ( #2461 ), #23988, .T. ) ;
#12146=ORIENTED_EDGE ( 'NONE', *, *, #25395, .F. ) ;
#12153=LINE ( 'NONE', #24543, #27144 ) ;
#12156=VECTOR ( 'NONE', #14968, 1000.000000000000000 ) ;
#12157=ORIENTED_EDGE ( 'NONE', *, *, #20055, .T. ) ;
#12159=ORIENTED_EDGE ( 'NONE', *, *, #11715, .T. ) ;
#12160=CARTESIAN_POINT ( 'NONE',  ( -9.625795778762141097, 10.95253033666833709, 11.00000000000000000 ) ) ;
#12161=DIRECTION ( 'NONE',  ( -0.7431448254773862505, 0.6691306063588670083, 0.000000000000000000 ) ) ;
#12166=DIRECTION ( 'NONE',  ( 0.9510565162951543083, 0.3090169943749450088, 0.000000000000000000 ) ) ;
#12167=CARTESIAN_POINT ( 'NONE',  ( -3.399837471815634338, 8.909889435135630364, 7.499999999999997335 ) ) ;
#12170=VECTOR ( 'NONE', #14902, 1000.000000000000000 ) ;
#12178=CIRCLE ( 'NONE', #18653, 6.000000000000014211 ) ;
#12180=VECTOR ( 'NONE', #31182, 1000.000000000000000 ) ;
#12184=CARTESIAN_POINT ( 'NONE',  ( 11.48173768534048556, 32.16538668264401934, 10.59344438985533721 ) ) ;
#12188=CARTESIAN_POINT ( 'NONE',  ( 0.6830608540009363017, 37.47223625998419294, 10.49999999999999822 ) ) ;
#12189=CARTESIAN_POINT ( 'NONE',  ( 10.81260707898150386, 32.90853150812155548, 7.000000000000000000 ) ) ;
#12190=CARTESIAN_POINT ( 'NONE',  ( 0.000000000000000000, 22.50000000000000355, 7.000000000000000000 ) ) ;
#12196=EDGE_LOOP ( 'NONE', ( #35266, #20507, #1502 ) ) ;
#12198=DIRECTION ( 'NONE',  ( 1.000000000000000000, 0.000000000000000000, 0.000000000000000000 ) ) ;
#12203=ORIENTED_EDGE ( 'NONE', *, *, #13731, .T. ) ;
#12205=AXIS2_PLACEMENT_3D ( 'NONE', #34295, #21302, #21891 ) ;
#12207=FACE_OUTER_BOUND ( 'NONE', #1507, .T. ) ;
#12209=CIRCLE ( 'NONE', #15457, 0.5000000000000004441 ) ;
#12211=ORIENTED_EDGE ( 'NONE', *, *, #24147, .T. ) ;
#12212=CARTESIAN_POINT ( 'NONE',  ( 3.699151772511975800, 7.951170058885261405, 10.49999999999999822 ) ) ;
#12213=EDGE_CURVE ( 'NONE', #35769, #22927, #6327, .T. ) ;
#12214=CARTESIAN_POINT ( 'NONE',  ( 10.24611365915863281, 21.92584419919065652, 10.75000000000001421 ) ) ;
#12216=CARTESIAN_POINT ( 'NONE',  ( 12.05736835487432579, 14.38397459621550567, 9.500000000000000000 ) ) ;
#12218=EDGE_CURVE ( 'NONE', #31473, #35530, #32953, .T. ) ;
#12219=CARTESIAN_POINT ( 'NONE',  ( -8.137585970691990411, 29.15429895402942861, 11.00000000000000000 ) ) ;
#12230=CARTESIAN_POINT ( 'NONE',  ( -3.523049899833476051, 8.330220536420963384, 10.99387789255783154 ) ) ;
#12231=VERTEX_POINT ( 'NONE', #17908 ) ;
#12235=FACE_OUTER_BOUND ( 'NONE', #18852, .T. ) ;
#12240=CARTESIAN_POINT ( 'NONE',  ( 13.86512115012093638, 28.22494587244850450, 7.203056206335839207 ) ) ;
#12241=EDGE_LOOP ( 'NONE', ( #454, #15891, #25024, #31618 ) ) ;
#12243=CARTESIAN_POINT ( 'NONE',  ( -3.992867117591420545, 8.524771480177605554, 11.00000000000000000 ) ) ;
#12244=CARTESIAN_POINT ( 'NONE',  ( -6.576253646258507501, 14.29921418520934395, 11.00000000000000000 ) ) ;
#12245=ADVANCED_FACE ( 'NONE', ( #14244 ), #12924, .T. ) ;
#12246=ORIENTED_EDGE ( 'NONE', *, *, #33997, .F. ) ;
#12252=ORIENTED_EDGE ( 'NONE', *, *, #24311, .F. ) ;
#12255=B_SPLINE_CURVE_WITH_KNOTS ( 'NONE', 3,
 ( #34569, #31916, #37622, #22170, #25414, #13631 ),
 .UNSPECIFIED., .F., .F.,
 ( 4, 2, 4 ),
 ( 0.000000000000000000, 0.5000000000000000000, 1.000000000000000000 ),
 .UNSPECIFIED. ) ;
#12257=VECTOR ( 'NONE', #1263, 1000.000000000000114 ) ;
#12261=CIRCLE ( 'NONE', #31089, 0.9999999999999998890 ) ;
#12263=ADVANCED_FACE ( 'NONE', ( #26432 ), #36194, .T. ) ;
#12266=ORIENTED_EDGE ( 'NONE', *, *, #37201, .F. ) ;
#12269=EDGE_CURVE ( 'NONE', #18776, #13281, #38829, .T. ) ;
#12270=CARTESIAN_POINT ( 'NONE',  ( -14.47283171447380390, 21.48159823030330529, 11.00000000000000000 ) ) ;
#12274=ORIENTED_EDGE ( 'NONE', *, *, #1118, .F. ) ;
#12279=EDGE_LOOP ( 'NONE', ( #5864, #34736, #32578 ) ) ;
#12281=ORIENTED_EDGE ( 'NONE', *, *, #437, .T. ) ;
#12285=CARTESIAN_POINT ( 'NONE',  ( 0.5000000000000000000, 37.50000000000000711, 7.000000000000000000 ) ) ;
#12286=AXIS2_PLACEMENT_3D ( 'NONE', #34850, #12706, #722 ) ;
#12289=CARTESIAN_POINT ( 'NONE',  ( 12.30736835487432579, 14.81698729810772619, 7.000000000000000000 ) ) ;
#12295=CARTESIAN_POINT ( 'NONE',  ( 6.973232007841551727, 35.78074362234890060, 7.338691926023217071 ) ) ;
#12298=AXIS2_PLACEMENT_3D ( 'NONE', #34949, #38390, #7505 ) ;
#12306=FACE_OUTER_BOUND ( 'NONE', #13674, .T. ) ;
#12307=EDGE_LOOP ( 'NONE', ( #22061, #38989, #28944 ) ) ;
#12310=VECTOR ( 'NONE', #20824, 1000.000000000000000 ) ;
#12315=PLANE ( 'NONE',  #5235 ) ;
#12317=AXIS2_PLACEMENT_3D ( 'NONE', #971, #19862, #25342 ) ;
#12319=EDGE_CURVE ( 'NONE', #12345, #13029, #3749, .T. ) ;
#12320=CARTESIAN_POINT ( 'NONE',  ( 11.73118655278371492, 31.84795188348743622, 7.381627713044569106 ) ) ;
#12323=VERTEX_POINT ( 'NONE', #30495 ) ;
#12325=DIRECTION ( 'NONE',  ( 0.000000000000000000, -0.5821182788257888152, 0.8131041196900314905 ) ) ;
#12326=CARTESIAN_POINT ( 'NONE',  ( 7.309360666678370144, 9.887575703124513282, 7.000000000000000000 ) ) ;
#12339=CARTESIAN_POINT ( 'NONE',  ( 13.48130249190479191, 27.93180293473185927, 7.500000000000000888 ) ) ;
#12345=VERTEX_POINT ( 'NONE', #24985 ) ;
#12346=CARTESIAN_POINT ( 'NONE',  ( -9.997483185316564658, 21.95197631500770541, 10.00000000000000000 ) ) ;
#12348=CIRCLE ( 'NONE', #9772, 0.5000000000000004441 ) ;
#12354=DIRECTION ( 'NONE',  ( -1.000000000000000000, -1.224646799147353947E-16, 0.000000000000000000 ) ) ;
#12355=CARTESIAN_POINT ( 'NONE',  ( 0.000000000000000000, 22.50000000000000355, 7.000000000000000000 ) ) ;
#12356=EDGE_CURVE ( 'NONE', #18033, #8130, #2855, .T. ) ;
#12359=EDGE_LOOP ( 'NONE', ( #33653, #27825, #13788 ) ) ;
#12360=EDGE_CURVE ( 'NONE', #11661, #33995, #3254, .T. ) ;
#12362=AXIS2_PLACEMENT_3D ( 'NONE', #22493, #32256, #7252 ) ;
#12363=LINE ( 'NONE', #9120, #4223 ) ;
#12364=CARTESIAN_POINT ( 'NONE',  ( 3.610593701936716027, 31.83882289796390097, 10.00000000000000000 ) ) ;
#12365=CARTESIAN_POINT ( 'NONE',  ( 3.295881626406578224, 9.398963235502483471, 9.500000000000000000 ) ) ;
#12370=ADVANCED_FACE ( 'NONE', ( #34337 ), #12393, .F. ) ;
#12374=CARTESIAN_POINT ( 'NONE',  ( -13.47830981910552772, 21.58612669357095015, 10.50000000000000000 ) ) ;
#12377=CARTESIAN_POINT ( 'NONE',  ( -8.401171878996500197, 21.11424711454089476, 7.000000000000000000 ) ) ;
#12381=FACE_OUTER_BOUND ( 'NONE', #4446, .T. ) ;
#12382=ORIENTED_EDGE ( 'NONE', *, *, #1071, .F. ) ;
#12384=EDGE_CURVE ( 'NONE', #39240, #18776, #6488, .T. ) ;
#12385=CARTESIAN_POINT ( 'NONE',  ( 0.5000000000000000000, 37.23829181893393070, 10.94387467462633623 ) ) ;
#12386=DIRECTION ( 'NONE',  ( -0.3090169943749414005, 0.9510565162951555296, 0.000000000000000000 ) ) ;
#12389=CARTESIAN_POINT ( 'NONE',  ( 12.99377146717205989, 26.19620116591418935, 9.500000000000000000 ) ) ;
#12390=ORIENTED_EDGE ( 'NONE', *, *, #20360, .T. ) ;
#12393=PLANE ( 'NONE',  #16726 ) ;
#12396=CARTESIAN_POINT ( 'NONE',  ( -14.09933648065464062, 26.02968990214173317, 9.500000000000000000 ) ) ;
#12397=ORIENTED_EDGE ( 'NONE', *, *, #32488, .F. ) ;
#12399=ORIENTED_EDGE ( 'NONE', *, *, #21193, .T. ) ;
#12404=EDGE_CURVE ( 'NONE', #27087, #21540, #26462, .T. ) ;
#12407=ORIENTED_EDGE ( 'NONE', *, *, #25769, .F. ) ;
#12409=CARTESIAN_POINT ( 'NONE',  ( 3.513409677696501365, 8.375574215747722207, 11.00000000000000355 ) ) ;
#12411=FACE_OUTER_BOUND ( 'NONE', #26031, .T. ) ;
#12415=LINE ( 'NONE', #15465, #13999 ) ;
#12420=CARTESIAN_POINT ( 'NONE',  ( 1.281526940109136037, 37.44563527730423402, 7.102474990965860435 ) ) ;
#12421=ORIENTED_EDGE ( 'NONE', *, *, #35953, .T. ) ;
#12425=AXIS2_PLACEMENT_3D ( 'NONE', #21530, #24384, #33545 ) ;
#12427=VERTEX_POINT ( 'NONE', #27434 ) ;
#12432=VERTEX_POINT ( 'NONE', #37181 ) ;
#12435=CARTESIAN_POINT ( 'NONE',  ( 0.5000000000000000000, 37.50000000000000711, 10.49999999999999822 ) ) ;
#12436=ORIENTED_EDGE ( 'NONE', *, *, #23555, .T. ) ;
#12438=DIRECTION ( 'NONE',  ( 1.000000000000000000, 0.000000000000000000, 0.000000000000000000 ) ) ;
#12439=CARTESIAN_POINT ( 'NONE',  ( -9.927394655428436465, 11.06314620770957013, 7.000000000000000000 ) ) ;
#12440=EDGE_CURVE ( 'NONE', #40188, #14680, #24388, .T. ) ;
#12445=B_SPLINE_CURVE_WITH_KNOTS ( 'NONE', 3,
 ( #27953, #18422, #40143, #12320, #127, #24706, #37106, #18623 ),
 .UNSPECIFIED., .F., .F.,
 ( 4, 2, 2, 4 ),
 ( 0.000000000000000000, 0.0002364868538934288911, 0.0004729737077868577822, 0.0009459474155737128539 ),
 .UNSPECIFIED. ) ;
#12446=CIRCLE ( 'NONE', #39037, 0.4999999999999998335 ) ;
#12450=ORIENTED_EDGE ( 'NONE', *, *, #35490, .F. ) ;
#12452=PLANE ( 'NONE',  #36915 ) ;
#12456=DIRECTION ( 'NONE',  ( 1.000000000000000000, 0.000000000000000000, 0.000000000000000000 ) ) ;
#12457=AXIS2_PLACEMENT_3D ( 'NONE', #16746, #6773, #22621 ) ;
#12463=CARTESIAN_POINT ( 'NONE',  ( -0.4999999999999998890, 37.00000000000000711, 7.000000000000000000 ) ) ;
#12467=ORIENTED_EDGE ( 'NONE', *, *, #22968, .T. ) ;
#12469=AXIS2_PLACEMENT_3D ( 'NONE', #7358, #876, #38045 ) ;
#12471=DIRECTION ( 'NONE',  ( 0.000000000000000000, 0.000000000000000000, 1.000000000000000000 ) ) ;
#12477=DIRECTION ( 'NONE',  ( -0.000000000000000000, -0.000000000000000000, -1.000000000000000000 ) ) ;
#12479=CARTESIAN_POINT ( 'NONE',  ( 5.237540274239914417, 35.49300472853430222, 7.500000000000000000 ) ) ;
#12483=DIRECTION ( 'NONE',  ( -0.000000000000000000, -0.000000000000000000, -1.000000000000000000 ) ) ;
#12485=ORIENTED_EDGE ( 'NONE', *, *, #11811, .F. ) ;
#12487=ADVANCED_FACE ( 'NONE', ( #6093 ), #37489, .T. ) ;
#12488=DIRECTION ( 'NONE',  ( 0.5877852522924691403, -0.8090169943749503378, -1.734723475976808672E-15 ) ) ;
#12489=CYLINDRICAL_SURFACE ( 'NONE', #18647, 0.5000000000000004441 ) ;
#12496=CARTESIAN_POINT ( 'NONE',  ( -5.578816091646024766, 36.25952276447313949, 10.87262190629284930 ) ) ;
#12497=ADVANCED_FACE ( 'NONE', ( #36984 ), #9150, .F. ) ;
#12499=EDGE_LOOP ( 'NONE', ( #30321, #26637, #13819, #18495 ) ) ;
#12500=EDGE_CURVE ( 'NONE', #24748, #28626, #19091, .T. ) ;
#12502=FACE_OUTER_BOUND ( 'NONE', #33390, .T. ) ;
#12503=VERTEX_POINT ( 'NONE', #16858 ) ;
#12505=B_SPLINE_CURVE_WITH_KNOTS ( 'NONE', 3,
 ( #5746, #3293, #12240, #21775, #37024, #2701, #2510, #24432 ),
 .UNSPECIFIED., .F., .F.,
 ( 4, 2, 2, 4 ),
 ( 0.000000000000000000, 0.0004726692273637226271, 0.0007090038410455847808, 0.0009453384547274468804 ),
 .UNSPECIFIED. ) ;
#12512=CARTESIAN_POINT ( 'NONE',  ( 14.50704651774852927, 20.00412295564763099, 10.49999999999999822 ) ) ;
#12513=CIRCLE ( 'NONE', #10576, 0.5000000000000004441 ) ;
#12515=FACE_OUTER_BOUND ( 'NONE', #19125, .T. ) ;
#12516=CARTESIAN_POINT ( 'NONE',  ( 2.672146553953306025, 12.33340603770390764, 10.00000000000000000 ) ) ;
#12517=CARTESIAN_POINT ( 'NONE',  ( -14.36830325120615903, 20.48707633493503621, 7.000000000000000000 ) ) ;
#12518=CARTESIAN_POINT ( 'NONE',  ( -14.36830325120615548, 20.48707633493503621, 7.000000000000000000 ) ) ;
#12520=CARTESIAN_POINT ( 'NONE',  ( -8.927394655428429360, 11.06314620770957013, 11.00000000000000000 ) ) ;
#12521=VERTEX_POINT ( 'NONE', #10348 ) ;
#12522=AXIS2_PLACEMENT_3D ( 'NONE', #9397, #30735, #15685 ) ;
#12524=LINE ( 'NONE', #31211, #1242 ) ;
#12530=ORIENTED_EDGE ( 'NONE', *, *, #16852, .T. ) ;
#12533=AXIS2_PLACEMENT_3D ( 'NONE', #20020, #3964, #37699 ) ;
#12541=ORIENTED_EDGE ( 'NONE', *, *, #7809, .F. ) ;
#12543=EDGE_CURVE ( 'NONE', #31959, #30328, #25577, .T. ) ;
#12544=VECTOR ( 'NONE', #35559, 1000.000000000000000 ) ;
#12547=DIRECTION ( 'NONE',  ( 0.4067366430757888840, -0.9135454576426058626, -0.000000000000000000 ) ) ;
#12552=CONICAL_SURFACE ( 'NONE', #8644, 1.000000000000004441, 0.7853981633974524978 ) ;
#12553=ORIENTED_EDGE ( 'NONE', *, *, #29898, .F. ) ;
#12554=FACE_OUTER_BOUND ( 'NONE', #27485, .T. ) ;
#12555=ORIENTED_EDGE ( 'NONE', *, *, #2053, .T. ) ;
#12556=PLANE ( 'NONE',  #26850 ) ;
#12560=CIRCLE ( 'NONE', #5436, 15.00000000000000000 ) ;
#12563=CARTESIAN_POINT ( 'NONE',  ( -7.935100905948476502, 11.57827057593827469, 7.000000000000000000 ) ) ;
#12564=EDGE_CURVE ( 'NONE', #22450, #37934, #28402, .T. ) ;
#12565=DIRECTION ( 'NONE',  ( 0.4999999999999919509, -0.8660254037844432595, 0.000000000000000000 ) ) ;
#12566=DIRECTION ( 'NONE',  ( 0.000000000000000000, 0.000000000000000000, -1.000000000000000000 ) ) ;
#12576=CARTESIAN_POINT ( 'NONE',  ( 11.19134295108988830, 14.88397459621551100, 10.00000000000000000 ) ) ;
#12578=AXIS2_PLACEMENT_3D ( 'NONE', #25339, #28390, #21699 ) ;
#12586=CARTESIAN_POINT ( 'NONE',  ( 0.5000000000000000000, 37.50000000000000711, 10.49999999999999822 ) ) ;
#12588=CARTESIAN_POINT ( 'NONE',  ( -11.11016527260153630, 31.83082137946488643, 9.500000000000000000 ) ) ;
#12589=VECTOR ( 'NONE', #37750, 1000.000000000000114 ) ;
#12590=CARTESIAN_POINT ( 'NONE',  ( 14.84898236231943258, 21.81673761604075779, 10.49999999999999822 ) ) ;
#12591=VERTEX_POINT ( 'NONE', #13791 ) ;
#12593=EDGE_CURVE ( 'NONE', #36614, #39958, #35132, .T. ) ;
#12596=VERTEX_POINT ( 'NONE', #38578 ) ;
#12598=FACE_OUTER_BOUND ( 'NONE', #33783, .T. ) ;
#12602=ADVANCED_FACE ( 'NONE', ( #38377 ), #22133, .T. ) ;
#12609=DIRECTION ( 'NONE',  ( -0.5000000000000038858, -0.8660254037844364872, 0.000000000000000000 ) ) ;
#12610=ORIENTED_EDGE ( 'NONE', *, *, #28726, .T. ) ;
#12611=DIRECTION ( 'NONE',  ( -1.000000000000000000, 0.000000000000000000, 0.000000000000000000 ) ) ;
#12614=EDGE_CURVE ( 'NONE', #38107, #13490, #38175, .T. ) ;
#12615=ADVANCED_FACE ( 'NONE', ( #13588 ), #4248, .F. ) ;
#12616=CARTESIAN_POINT ( 'NONE',  ( -12.80736835487442349, 15.68301270189233954, 9.000000000000001776 ) ) ;
#12617=ADVANCED_FACE ( 'NONE', ( #606 ), #6683, .F. ) ;
#12621=CARTESIAN_POINT ( 'NONE',  ( -9.840690490415104463, 20.46019347195529647, 10.49999999999999467 ) ) ;
#12623=ORIENTED_EDGE ( 'NONE', *, *, #32604, .T. ) ;
#12628=ORIENTED_EDGE ( 'NONE', *, *, #29498, .T. ) ;
#12629=VERTEX_POINT ( 'NONE', #7084 ) ;
#12631=CIRCLE ( 'NONE', #38587, 5.999999999999996447 ) ;
#12633=EDGE_CURVE ( 'NONE', #36832, #19894, #31880, .T. ) ;
#12635=CIRCLE ( 'NONE', #2894, 0.5000000000000004441 ) ;
#12636=ORIENTED_EDGE ( 'NONE', *, *, #36600, .T. ) ;
#12640=ORIENTED_EDGE ( 'NONE', *, *, #34551, .T. ) ;
#12642=ADVANCED_FACE ( 'NONE', ( #25781 ), #7284, .F. ) ;
#12643=CARTESIAN_POINT ( 'NONE',  ( -6.354454053420244719, 35.54304081427989814, 9.500000000000000000 ) ) ;
#12644=CARTESIAN_POINT ( 'NONE',  ( 12.37435565298211415, 15.93301270189216545, 7.000000000000000000 ) ) ;
#12645=ORIENTED_EDGE ( 'NONE', *, *, #33487, .F. ) ;
#12647=EDGE_LOOP ( 'NONE', ( #31709, #32580, #438, #297, #27832, #29479, #14578 ) ) ;
#12653=CARTESIAN_POINT ( 'NONE',  ( -14.44277748876678302, 26.55045409923029354, 7.000000000000000000 ) ) ;
#12656=CARTESIAN_POINT ( 'NONE',  ( -13.48130249190472796, 27.93180293473203690, 7.499999999999993783 ) ) ;
#12657=FACE_OUTER_BOUND ( 'NONE', #29124, .T. ) ;
#12662=CARTESIAN_POINT ( 'NONE',  ( 4.524139159579314118, 31.43208625488810171, 10.49999999999999822 ) ) ;
#12663=CARTESIAN_POINT ( 'NONE',  ( 3.784364466546041417, 47.62563423532509432, 7.500000000000005329 ) ) ;
#12673=DIRECTION ( 'NONE',  ( 0.9135454576426059736, 0.4067366430757888285, 0.000000000000000000 ) ) ;
#12674=ORIENTED_EDGE ( 'NONE', *, *, #19251, .T. ) ;
#12676=DIRECTION ( 'NONE',  ( -0.000000000000000000, -0.000000000000000000, -1.000000000000000000 ) ) ;
#12679=EDGE_LOOP ( 'NONE', ( #11739, #5119, #1016, #32761, #30456 ) ) ;
#12682=FACE_OUTER_BOUND ( 'NONE', #4252, .T. ) ;
#12686=CARTESIAN_POINT ( 'NONE',  ( 0.5000000000000000000, 37.00000000000000711, 7.000000000000000000 ) ) ;
#12687=CARTESIAN_POINT ( 'NONE',  ( 6.789742187716170108, 35.87551282667536157, 7.455539900862802938 ) ) ;
#12688=CARTESIAN_POINT ( 'NONE',  ( -10.81260707898136708, 32.90853150812171179, 10.49999999999999822 ) ) ;
#12690=VERTEX_POINT ( 'NONE', #39379 ) ;
#12693=VECTOR ( 'NONE', #22127, 1000.000000000000114 ) ;
#12695=ORIENTED_EDGE ( 'NONE', *, *, #26182, .T. ) ;
#12697=FACE_OUTER_BOUND ( 'NONE', #19330, .T. ) ;
#12699=DIRECTION ( 'NONE',  ( 0.2185080122244111578, -0.6724985119639586006, -0.7071067811865462405 ) ) ;
#12700=LINE ( 'NONE', #2578, #7145 ) ;
#12704=EDGE_CURVE ( 'NONE', #36810, #39240, #3894, .T. ) ;
#12705=CARTESIAN_POINT ( 'NONE',  ( -8.412270287199726582, 10.07085245822961994, 11.00000000000000000 ) ) ;
#12706=DIRECTION ( 'NONE',  ( 0.9945218953682729568, -0.1045284632676570929, -0.000000000000000000 ) ) ;
#12707=VECTOR ( 'NONE', #33740, 1000.000000000000000 ) ;
#12709=DIRECTION ( 'NONE',  ( -0.9510565162951504226, 0.3090169943749573322, 0.000000000000000000 ) ) ;
#12710=DIRECTION ( 'NONE',  ( -0.8090169943749426773, 0.5877852522924796874, 0.000000000000000000 ) ) ;
#12712=CARTESIAN_POINT ( 'NONE',  ( 13.05736835487433289, 16.11602540378438420, 10.50000000000000178 ) ) ;
#12714=ORIENTED_EDGE ( 'NONE', *, *, #13395, .F. ) ;
#12716=DIRECTION ( 'NONE',  ( 0.000000000000000000, -0.000000000000000000, -1.000000000000000000 ) ) ;
#12718=EDGE_CURVE ( 'NONE', #26207, #14734, #20299, .T. ) ;
#12719=DIRECTION ( 'NONE',  ( 0.000000000000000000, 0.000000000000000000, -1.000000000000000000 ) ) ;
#12720=CIRCLE ( 'NONE', #33512, 0.9999999999999996669 ) ;
#12722=ADVANCED_FACE ( 'NONE', ( #5254 ), #6747, .T. ) ;
#12726=ORIENTED_EDGE ( 'NONE', *, *, #8815, .T. ) ;
#12727=CARTESIAN_POINT ( 'NONE',  ( -6.282361020112269934, 14.70372268239681368, 10.00000000000000000 ) ) ;
#12734=CARTESIAN_POINT ( 'NONE',  ( 11.56932667689157057, 32.06810925246610822, 10.49999999999999645 ) ) ;
#12739=LINE ( 'NONE', #21689, #3072 ) ;
#12741=CARTESIAN_POINT ( 'NONE',  ( -14.36830325120616081, 20.48707633493503977, 11.00000000000000000 ) ) ;
#12748=ORIENTED_EDGE ( 'NONE', *, *, #20565, .T. ) ;
#12749=DIRECTION ( 'NONE',  ( 0.9781476007338042455, -0.2079116908177664480, 0.000000000000000000 ) ) ;
#12750=VERTEX_POINT ( 'NONE', #11357 ) ;
#12751=CARTESIAN_POINT ( 'NONE',  ( 4.591666147298500533, 15.32946292166668556, 9.000000000000001776 ) ) ;
#12755=ORIENTED_EDGE ( 'NONE', *, *, #3069, .F. ) ;
#12757=CARTESIAN_POINT ( 'NONE',  ( -9.427394962683591118, 11.06314620782489833, 10.49999999999999822 ) ) ;
#12759=CARTESIAN_POINT ( 'NONE',  ( -7.848705329595171420, 10.27943253798625989, 10.66666666666666607 ) ) ;
#12762=ADVANCED_FACE ( 'NONE', ( #32901 ), #35938, .T. ) ;
#12763=FACE_OUTER_BOUND ( 'NONE', #5461, .T. ) ;
#12765=ORIENTED_EDGE ( 'NONE', *, *, #8884, .F. ) ;
#12767=DIRECTION ( 'NONE',  ( 1.000000000000000000, 0.000000000000000000, 0.000000000000000000 ) ) ;
#12769=LINE ( 'NONE', #3828, #6802 ) ;
#12772=CARTESIAN_POINT ( 'NONE',  ( -10.33648234394568632, 33.08013173297169374, 10.49999999999999467 ) ) ;
#12773=AXIS2_PLACEMENT_3D ( 'NONE', #18600, #28525, #30983 ) ;
#12774=CONICAL_SURFACE ( 'NONE', #11484, 1.000000000000002665, 0.7853981633974530530 ) ;
#12779=CARTESIAN_POINT ( 'NONE',  ( 13.48130249190479191, 27.93180293473185927, 10.49999999999999822 ) ) ;
#12784=LINE ( 'NONE', #9746, #36694 ) ;
#12785=AXIS2_PLACEMENT_3D ( 'NONE', #12121, #9677, #15365 ) ;
#12787=ORIENTED_EDGE ( 'NONE', *, *, #12213, .F. ) ;
#12790=EDGE_CURVE ( 'NONE', #36749, #38004, #35536, .T. ) ;
#12791=CARTESIAN_POINT ( 'NONE',  ( -12.83926296998452798, 26.67172942406192604, 7.000000000000000000 ) ) ;
#12793=ORIENTED_EDGE ( 'NONE', *, *, #10502, .F. ) ;
#12795=DIRECTION ( 'NONE',  ( -0.4731467892558211541, -0.5254827454987550661, -0.7071067811865462405 ) ) ;
#12796=ORIENTED_EDGE ( 'NONE', *, *, #22264, .F. ) ;
#12798=EDGE_LOOP ( 'NONE', ( #20149, #6523, #166, #15895, #27431 ) ) ;
#12800=DIRECTION ( 'NONE',  ( -1.000000000000000000, 0.000000000000000000, 0.000000000000000000 ) ) ;
#12801=CARTESIAN_POINT ( 'NONE',  ( -7.713869163866016621, 10.18146832927085121, 10.50000000000000711 ) ) ;
#12804=DIRECTION ( 'NONE',  ( 0.000000000000000000, 0.000000000000000000, -1.000000000000000000 ) ) ;
#12806=PLANE ( 'NONE',  #14458 ) ;
#12809=VECTOR ( 'NONE', #18805, 1000.000000000000000 ) ;
#12810=CARTESIAN_POINT ( 'NONE',  ( 13.13581098909226696, 27.45627467658428955, 7.500000000000000888 ) ) ;
#12811=EDGE_CURVE ( 'NONE', #32326, #163, #5054, .T. ) ;
#12817=CARTESIAN_POINT ( 'NONE',  ( 4.096822963000107620, 8.035697679810645866, 11.00000000000000000 ) ) ;
#12818=DIRECTION ( 'NONE',  ( -0.000000000000000000, -0.000000000000000000, -1.000000000000000000 ) ) ;
#12819=VERTEX_POINT ( 'NONE', #2807 ) ;
#12824=EDGE_LOOP ( 'NONE', ( #29813, #1627, #7520, #26874 ) ) ;
#12835=CARTESIAN_POINT ( 'NONE',  ( -13.59328760765163224, 16.15712598384885013, 7.083533146543740777 ) ) ;
#12838=DIRECTION ( 'NONE',  ( -0.4067366430757888840, 0.9135454576426058626, 0.000000000000000000 ) ) ;
#12839=DIRECTION ( 'NONE',  ( 1.000000000000000000, 0.000000000000000000, 0.000000000000000000 ) ) ;
#12840=AXIS2_PLACEMENT_3D ( 'NONE', #27495, #39880, #6349 ) ;
#12842=ADVANCED_FACE ( 'NONE', ( #11954 ), #5854, .T. ) ;
#12844=EDGE_LOOP ( 'NONE', ( #32160, #28141, #10123, #35913 ) ) ;
#12845=ADVANCED_FACE ( 'NONE', ( #21884 ), #24344, .F. ) ;
#12852=CARTESIAN_POINT ( 'NONE',  ( -13.49038105676664223, 15.86602540378456361, 10.49999999999999822 ) ) ;
#12853=CARTESIAN_POINT ( 'NONE',  ( -7.713869163866016621, 10.18146832927085121, 11.00000000000000000 ) ) ;
#12854=EDGE_CURVE ( 'NONE', #29281, #29040, #19350, .T. ) ;
#12855=AXIS2_PLACEMENT_3D ( 'NONE', #34183, #9600, #36828 ) ;
#12857=EDGE_CURVE ( 'NONE', #10635, #19442, #33703, .T. ) ;
#12861=CONICAL_SURFACE ( 'NONE', #3791, 0.4999999999999897304, 0.7853981633974508325 ) ;
#12862=LINE ( 'NONE', #37650, #6003 ) ;
#12868=CARTESIAN_POINT ( 'NONE',  ( 10.17939521785132051, 33.00296324411745275, 10.49999999999999822 ) ) ;
#12870=ORIENTED_EDGE ( 'NONE', *, *, #15601, .T. ) ;
#12871=FACE_OUTER_BOUND ( 'NONE', #36277, .T. ) ;
#12874=DIRECTION ( 'NONE',  ( -1.000000000000000000, 0.000000000000000000, 0.000000000000000000 ) ) ;
#12877=ORIENTED_EDGE ( 'NONE', *, *, #28544, .F. ) ;
#12880=DIRECTION ( 'NONE',  ( 0.1045284632676570929, 0.9945218953682730678, 0.000000000000000000 ) ) ;
#12882=EDGE_LOOP ( 'NONE', ( #28157, #39625, #5932 ) ) ;
#12884=CARTESIAN_POINT ( 'NONE',  ( -0.5000000000000004441, 36.50000000000000711, 7.500000000000000888 ) ) ;
#12885=CARTESIAN_POINT ( 'NONE',  ( 14.57486473880226185, 26.18419839932902349, 10.50000000000000533 ) ) ;
#12886=DIRECTION ( 'NONE',  ( 0.9945218953682729568, -0.1045284632676569680, 0.000000000000000000 ) ) ;
#12887=ORIENTED_EDGE ( 'NONE', *, *, #2842, .T. ) ;
#12890=ADVANCED_FACE ( 'NONE', ( #5648 ), #3210, .T. ) ;
#12896=CONICAL_SURFACE ( 'NONE', #2528, 1.000000000000007772, 0.7853981633974554954 ) ;
#12899=ORIENTED_EDGE ( 'NONE', *, *, #34199, .T. ) ;
#12900=CARTESIAN_POINT ( 'NONE',  ( -9.697889840765284930, 31.90483559858340357, 10.50000000000000000 ) ) ;
#12902=CARTESIAN_POINT ( 'NONE',  ( -5.947717410344459665, 34.62949535663729250, 9.500000000000000000 ) ) ;
#12904=EDGE_CURVE ( 'NONE', #4586, #5579, #11568, .T. ) ;
#12905=CARTESIAN_POINT ( 'NONE',  ( 9.997483185316561105, 21.95197631500756685, 10.00000000000000000 ) ) ;
#12906=CARTESIAN_POINT ( 'NONE',  ( 14.70550430380716023, 20.45163507617042242, 10.87262190629277647 ) ) ;
#12907=DIRECTION ( 'NONE',  ( -0.000000000000000000, -0.000000000000000000, -1.000000000000000000 ) ) ;
#12908=FACE_OUTER_BOUND ( 'NONE', #24879, .T. ) ;
#12909=CARTESIAN_POINT ( 'NONE',  ( 13.37378135583784911, 20.59160479820249634, 7.000000000000000000 ) ) ;
#12910=CARTESIAN_POINT ( 'NONE',  ( -0.5000000000000004441, 36.50000000000000711, 7.500000000000000888 ) ) ;
#12911=CIRCLE ( 'NONE', #35640, 1.000000000000002665 ) ;
#12913=CARTESIAN_POINT ( 'NONE',  ( 13.30736835483207692, 15.77027916469364577, 10.49999999999999822 ) ) ;
#12914=AXIS2_PLACEMENT_3D ( 'NONE', #39547, #14967, #36506 ) ;
#12915=EDGE_LOOP ( 'NONE', ( #3053, #4455, #21058, #19989 ) ) ;
#12917=CARTESIAN_POINT ( 'NONE',  ( 2.629601561899396422, 7.723830143584014429, 10.50000000000000533 ) ) ;
#12918=CARTESIAN_POINT ( 'NONE',  ( 12.74038105676654453, 14.56698729810772264, 11.00000000000000000 ) ) ;
#12920=CARTESIAN_POINT ( 'NONE',  ( 14.33346043011691329, 20.15556903647874165, 10.66666666666666963 ) ) ;
#12924=B_SPLINE_SURFACE_WITH_KNOTS ( 'NONE', 1, 3, ( 
 ( #39422, #39623, #11202, #11605, #21142, #20944, #24185, #2065, #26634, #36581 ),
 ( #23593, #4702, #33148, #33351, #4903, #20351, #1866, #5301, #17107, #35989 ) ),
 .UNSPECIFIED., .F., .F., .F.,
 ( 2, 2 ),
 ( 4, 2, 2, 2, 4 ),
 ( 0.000000000000000000, 1.000000000000000000 ),
 ( 4.563205465131944472, 4.955904546830669943, 5.348603628529396303, 5.741302710228122663, 6.134001791926849023 ),
 .UNSPECIFIED. ) ;
#12925=ORIENTED_EDGE ( 'NONE', *, *, #31386, .T. ) ;
#12934=FACE_OUTER_BOUND ( 'NONE', #39529, .T. ) ;
#12936=ORIENTED_EDGE ( 'NONE', *, *, #15353, .F. ) ;
#12946=CIRCLE ( 'NONE', #23341, 6.000000000000015987 ) ;
#12950=AXIS2_PLACEMENT_3D ( 'NONE', #28392, #3019, #31249 ) ;
#12952=CYLINDRICAL_SURFACE ( 'NONE', #39685, 0.5000000000000000000 ) ;
#12953=DIRECTION ( 'NONE',  ( 0.3090169943749450643, -0.9510565162951544194, 0.000000000000000000 ) ) ;
#12954=VERTEX_POINT ( 'NONE', #24939 ) ;
#12959=CARTESIAN_POINT ( 'NONE',  ( 10.54700836463452518, 22.39697303105787540, 10.50000000000000533 ) ) ;
#12960=CARTESIAN_POINT ( 'NONE',  ( 11.54666566735224364, 32.07468077621332725, 7.499999999999997335 ) ) ;
#12962=EDGE_LOOP ( 'NONE', ( #7412, #10545, #18337, #21991 ) ) ;
#12965=EDGE_CURVE ( 'NONE', #11714, #21064, #27589, .T. ) ;
#12967=PLANE ( 'NONE',  #39244 ) ;
#12970=CARTESIAN_POINT ( 'NONE',  ( 10.36702044712426840, 31.16169077310587809, 9.500000000000000000 ) ) ;
#12971=VECTOR ( 'NONE', #1636, 1000.000000000000114 ) ;
#12976=CARTESIAN_POINT ( 'NONE',  ( 13.95827473762443027, 27.56104949980340280, 10.87262190629280845 ) ) ;
#12977=DIRECTION ( 'NONE',  ( -0.9781476007338072431, -0.2079116908177516265, 0.000000000000000000 ) ) ;
#12978=ORIENTED_EDGE ( 'NONE', *, *, #36204, .F. ) ;
#12979=VECTOR ( 'NONE', #22638, 1000.000000000000000 ) ;
#12981=CARTESIAN_POINT ( 'NONE',  ( -7.790810073469786268, 10.07556825234761533, 10.49999999999999645 ) ) ;
#12982=CARTESIAN_POINT ( 'NONE',  ( 10.47804177580207607, 33.28010392086025604, 7.000000000000000000 ) ) ;
#12986=EDGE_CURVE ( 'NONE', #16736, #1570, #18703, .T. ) ;
#12987=DIRECTION ( 'NONE',  ( -1.000000000000000000, 0.000000000000000000, 0.000000000000000000 ) ) ;
#12990=CARTESIAN_POINT ( 'NONE',  ( 9.151574469205250750, 1.945227203041362207, 7.000000000000000000 ) ) ;
#12991=ORIENTED_EDGE ( 'NONE', *, *, #30031, .F. ) ;
#12993=CIRCLE ( 'NONE', #34493, 0.5000000000000004441 ) ;
#12994=EDGE_CURVE ( 'NONE', #5398, #11410, #12153, .T. ) ;
#12995=ORIENTED_EDGE ( 'NONE', *, *, #23533, .T. ) ;
#12998=CARTESIAN_POINT ( 'NONE',  ( -4.591666147298613332, 15.32946292166675306, 9.000000000000001776 ) ) ;
#13001=FACE_OUTER_BOUND ( 'NONE', #2102, .T. ) ;
#13006=TOROIDAL_SURFACE ( 'NONE', #38975, 1.000000000000000000, 0.5000000000000000000 ) ;
#13007=FACE_OUTER_BOUND ( 'NONE', #17499, .T. ) ;
#13010=VERTEX_POINT ( 'NONE', #15998 ) ;
#13011=EDGE_CURVE ( 'NONE', #26241, #33406, #25332, .T. ) ;
#13012=ADVANCED_FACE ( 'NONE', ( #13543 ), #22881, .T. ) ;
#13014=DIRECTION ( 'NONE',  ( -0.9781476007338069101, -0.2079116908177533751, 0.000000000000000000 ) ) ;
#13015=LINE ( 'NONE', #31510, #34901 ) ;
#13016=VERTEX_POINT ( 'NONE', #19638 ) ;
#13022=EDGE_LOOP ( 'NONE', ( #18172, #12714, #14702, #34423 ) ) ;
#13024=PLANE ( 'NONE',  #23035 ) ;
#13028=CARTESIAN_POINT ( 'NONE',  ( 11.11016527260166953, 31.83082137946472656, 11.00000000000000000 ) ) ;
#13029=VERTEX_POINT ( 'NONE', #13338 ) ;
#13032=CARTESIAN_POINT ( 'NONE',  ( 7.766013557953380442, 28.81973365084987293, 10.49999999999999467 ) ) ;
#13034=ORIENTED_EDGE ( 'NONE', *, *, #33614, .F. ) ;
#13036=EDGE_CURVE ( 'NONE', #34540, #19729, #9619, .T. ) ;
#13042=LINE ( 'NONE', #37831, #1372 ) ;
#13044=AXIS2_PLACEMENT_3D ( 'NONE', #29098, #8371, #30310 ) ;
#13047=PLANE ( 'NONE',  #24054 ) ;
#13049=CARTESIAN_POINT ( 'NONE',  ( -4.794796183862964689, 36.71301971979259804, 7.000000000000000000 ) ) ;
#13052=LINE ( 'NONE', #10419, #20922 ) ;
#13053=ADVANCED_FACE ( 'NONE', ( #22089 ), #10252, .T. ) ;
#13055=VERTEX_POINT ( 'NONE', #6835 ) ;
#13058=CARTESIAN_POINT ( 'NONE',  ( 10.47540670418223208, 32.60491492691330961, 10.99999999999999645 ) ) ;
#13060=ORIENTED_EDGE ( 'NONE', *, *, #12811, .F. ) ;
#13062=LINE ( 'NONE', #31558, #20326 ) ;
#13063=ORIENTED_EDGE ( 'NONE', *, *, #25974, .F. ) ;
#13065=CARTESIAN_POINT ( 'NONE',  ( 8.315274455032101386, 10.01576150750513250, 7.500000000000000888 ) ) ;
#13067=CARTESIAN_POINT ( 'NONE',  ( 12.48446084878463225, 14.34248059624565563, 10.49999999999999822 ) ) ;
#13068=VECTOR ( 'NONE', #4671, 1000.000000000000000 ) ;
#13069=ORIENTED_EDGE ( 'NONE', *, *, #29468, .F. ) ;
#13072=DIRECTION ( 'NONE',  ( 1.000000000000000000, 0.000000000000000000, 0.000000000000000000 ) ) ;
#13074=ORIENTED_EDGE ( 'NONE', *, *, #2328, .T. ) ;
#13079=CARTESIAN_POINT ( 'NONE',  ( -10.17939521785135071, 33.00296324411767301, 10.49999999999999822 ) ) ;
#13082=EDGE_CURVE ( 'NONE', #36614, #32296, #15054, .T. ) ;
#13084=EDGE_CURVE ( 'NONE', #2909, #1082, #34488, .T. ) ;
#13086=ORIENTED_EDGE ( 'NONE', *, *, #30958, .F. ) ;
#13088=DIRECTION ( 'NONE',  ( 1.000000000000000000, 0.000000000000000000, 0.000000000000000000 ) ) ;
#13089=ADVANCED_FACE ( 'NONE', ( #25931 ), #38330, .T. ) ;
#13090=EDGE_LOOP ( 'NONE', ( #26795, #16644, #36132, #23744, #29365 ) ) ;
#13092=CARTESIAN_POINT ( 'NONE',  ( -10.44103466624267362, 32.57396620494225914, 11.00000000000000000 ) ) ;
#13093=DIRECTION ( 'NONE',  ( -0.9135454576426059736, -0.4067366430757889395, 0.000000000000000000 ) ) ;
#13096=ORIENTED_EDGE ( 'NONE', *, *, #12500, .T. ) ;
#13097=CARTESIAN_POINT ( 'NONE',  ( 8.910254037844367758, 17.93301270189219210, 10.00000000000000000 ) ) ;
#13098=CARTESIAN_POINT ( 'NONE',  ( 1.439880186556678821, -2.006054360071897857, 9.500000000000000000 ) ) ;
#13100=EDGE_CURVE ( 'NONE', #37186, #7787, #32331, .T. ) ;
#13107=FACE_OUTER_BOUND ( 'NONE', #39902, .T. ) ;
#13108=EDGE_LOOP ( 'NONE', ( #13520, #20429, #2899, #31364 ) ) ;
#13110=DIRECTION ( 'NONE',  ( -0.000000000000000000, -0.000000000000000000, -1.000000000000000000 ) ) ;
#13114=CARTESIAN_POINT ( 'NONE',  ( -7.929471891321301591, 25.60217271033470610, 9.000000000000001776 ) ) ;
#13118=ORIENTED_EDGE ( 'NONE', *, *, #30794, .T. ) ;
#13119=CARTESIAN_POINT ( 'NONE',  ( 14.42035624161478857, 26.65972665747660031, 10.49999999999999822 ) ) ;
#13129=VERTEX_POINT ( 'NONE', #10300 ) ;
#13133=CIRCLE ( 'NONE', #17042, 0.5000000000000004441 ) ;
#13135=ADVANCED_FACE ( 'NONE', ( #28984 ), #1162, .T. ) ;
#13137=DIRECTION ( 'NONE',  ( 0.9945218953682730678, -0.1045284632676569819, 0.000000000000000000 ) ) ;
#13138=AXIS2_PLACEMENT_3D ( 'NONE', #12106, #11711, #21055 ) ;
#13140=AXIS2_PLACEMENT_3D ( 'NONE', #19400, #19603, #1124 ) ;
#13142=VERTEX_POINT ( 'NONE', #32855 ) ;
#13143=AXIS2_PLACEMENT_3D ( 'NONE', #3055, #33754, #12198 ) ;
#13148=DIRECTION ( 'NONE',  ( 0.000000000000000000, 0.000000000000000000, 1.000000000000000000 ) ) ;
#13149=ORIENTED_EDGE ( 'NONE', *, *, #35765, .T. ) ;
#13151=CARTESIAN_POINT ( 'NONE',  ( -14.03791758423776592, 27.78611923485716773, 7.485699520496972070 ) ) ;
#13152=CARTESIAN_POINT ( 'NONE',  ( -14.94482798346716557, 26.50521816028930999, 7.000000000000000000 ) ) ;
#13155=DIRECTION ( 'NONE',  ( 0.9781476007338042455, -0.2079116908177663647, 0.000000000000000000 ) ) ;
#13157=DIRECTION ( 'NONE',  ( 1.000000000000000000, 0.000000000000000000, 0.000000000000000000 ) ) ;
#13161=DIRECTION ( 'NONE',  ( 0.000000000000000000, 0.000000000000000000, 1.000000000000000000 ) ) ;
#13163=LINE ( 'NONE', #16227, #37970 ) ;
#13164=EDGE_CURVE ( 'NONE', #32632, #21064, #13948, .T. ) ;
#13173=CARTESIAN_POINT ( 'NONE',  ( 14.08493436138100030, 27.60220370627940767, 10.68306085400108074 ) ) ;
#13174=PLANE ( 'NONE',  #36490 ) ;
#13179=ORIENTED_EDGE ( 'NONE', *, *, #22198, .T. ) ;
#13181=CARTESIAN_POINT ( 'NONE',  ( -2.036571916123809167, 8.108948098542077432, 9.500000000000000000 ) ) ;
#13187=VERTEX_POINT ( 'NONE', #23091 ) ;
#13189=VECTOR ( 'NONE', #11323, 1000.000000000000227 ) ;
#13190=ORIENTED_EDGE ( 'NONE', *, *, #29239, .T. ) ;
#13193=CARTESIAN_POINT ( 'NONE',  ( 6.651296319737277862, 27.81603774131160023, 9.000000000000001776 ) ) ;
#13194=CARTESIAN_POINT ( 'NONE',  ( -0.9674447320696243358, 37.46890771325332281, 7.339470489435490741 ) ) ;
#13197=FACE_OUTER_BOUND ( 'NONE', #28361, .T. ) ;
#13198=EDGE_LOOP ( 'NONE', ( #5692, #8899, #13403, #21303 ) ) ;
#13199=PRESENTATION_STYLE_ASSIGNMENT (( #14010 ) ) ;
#13202=PLANE ( 'NONE',  #32519 ) ;
#13205=AXIS2_PLACEMENT_3D ( 'NONE', #7294, #29644, #14207 ) ;
#13206=ORIENTED_EDGE ( 'NONE', *, *, #22684, .F. ) ;
#13207=EDGE_CURVE ( 'NONE', #28046, #4170, #17624, .T. ) ;
#13209=DIRECTION ( 'NONE',  ( 0.7771459614569745655, 0.6293203910498328391, 0.000000000000000000 ) ) ;
#13210=FACE_OUTER_BOUND ( 'NONE', #7779, .T. ) ;
#13211=ORIENTED_EDGE ( 'NONE', *, *, #969, .F. ) ;
#13213=AXIS2_PLACEMENT_3D ( 'NONE', #1521, #14108, #38697 ) ;
#13216=ADVANCED_FACE ( 'NONE', ( #8462 ), #33062, .F. ) ;
#13218=EDGE_CURVE ( 'NONE', #38584, #40188, #18068, .T. ) ;
#13220=ORIENTED_EDGE ( 'NONE', *, *, #8221, .F. ) ;
#13222=CARTESIAN_POINT ( 'NONE',  ( -10.44103466624267185, 32.57396620494226624, 9.000000000000001776 ) ) ;
#13224=VECTOR ( 'NONE', #3371, 999.9999999999998863 ) ;
#13226=DIRECTION ( 'NONE',  ( 1.000000000000000000, 0.000000000000000000, 0.000000000000000000 ) ) ;
#13231=CARTESIAN_POINT ( 'NONE',  ( 14.64659974985904967, 21.96608861361208298, 10.49999999999999645 ) ) ;
#13235=ORIENTED_EDGE ( 'NONE', *, *, #21061, .T. ) ;
#13240=EDGE_CURVE ( 'NONE', #5911, #9357, #2170, .T. ) ;
#13241=ORIENTED_EDGE ( 'NONE', *, *, #2346, .T. ) ;
#13243=ADVANCED_FACE ( 'NONE', ( #14555 ), #36886, .T. ) ;
#13244=DIRECTION ( 'NONE',  ( -0.000000000000000000, -0.000000000000000000, -1.000000000000000000 ) ) ;
#13247=CARTESIAN_POINT ( 'NONE',  ( 12.30736835487432579, 14.81698729810772619, 7.499999999999997335 ) ) ;
#13248=LINE ( 'NONE', #6944, #18858 ) ;
#13250=CONICAL_SURFACE ( 'NONE', #32765, 0.5000000000000002220, 0.7853981633974514986 ) ;
#13255=CARTESIAN_POINT ( 'NONE',  ( -13.19674782540811186, 16.00858767546144534, 10.49999999999999467 ) ) ;
#13259=ORIENTED_EDGE ( 'NONE', *, *, #9158, .T. ) ;
#13262=DIRECTION ( 'NONE',  ( 0.000000000000000000, -0.6037757019622788102, -0.7971542521494553446 ) ) ;
#13264=ORIENTED_EDGE ( 'NONE', *, *, #571, .F. ) ;
#13266=CARTESIAN_POINT ( 'NONE',  ( -10.39021566973307031, 20.90519018800561568, 11.00000000000000000 ) ) ;
#13267=VERTEX_POINT ( 'NONE', #39131 ) ;
#13271=DIRECTION ( 'NONE',  ( 1.000000000000000000, 0.000000000000000000, 0.000000000000000000 ) ) ;
#13272=VERTEX_POINT ( 'NONE', #29388 ) ;
#13277=ORIENTED_EDGE ( 'NONE', *, *, #11770, .F. ) ;
#13281=VERTEX_POINT ( 'NONE', #35892 ) ;
#13286=ORIENTED_EDGE ( 'NONE', *, *, #7533, .T. ) ;
#13288=AXIS2_PLACEMENT_3D ( 'NONE', #10268, #28156, #332 ) ;
#13290=PLANE ( 'NONE',  #6309 ) ;
#13291=AXIS2_PLACEMENT_3D ( 'NONE', #31646, #16214, #28597 ) ;
#13294=CARTESIAN_POINT ( 'NONE',  ( 0.000000000000000000, 37.50000000000000711, 7.000000000000000000 ) ) ;
#13297=ORIENTED_EDGE ( 'NONE', *, *, #13544, .F. ) ;
#13299=DIRECTION ( 'NONE',  ( -0.000000000000000000, 0.000000000000000000, 1.000000000000000000 ) ) ;
#13301=CARTESIAN_POINT ( 'NONE',  ( 10.44103466624280507, 32.57396620494213124, 11.00000000000000000 ) ) ;
#13302=CARTESIAN_POINT ( 'NONE',  ( 9.771904059883945948, 33.31711103041952526, 7.000000000000000000 ) ) ;
#13304=VECTOR ( 'NONE', #29871, 1000.000000000000000 ) ;
#13310=CARTESIAN_POINT ( 'NONE',  ( 13.28710335604435144, 15.51393809808774549, 10.49999999999999822 ) ) ;
#13313=CARTESIAN_POINT ( 'NONE',  ( -3.597409820281606940, 14.42008525284352594, 9.000000000000001776 ) ) ;
#13317=ORIENTED_EDGE ( 'NONE', *, *, #27356, .T. ) ;
#13318=AXIS2_PLACEMENT_3D ( 'NONE', #15977, #23064, #34660 ) ;
#13320=FACE_OUTER_BOUND ( 'NONE', #32342, .T. ) ;
#13324=ADVANCED_FACE ( 'NONE', ( #14354 ), #1884, .T. ) ;
#13325=CIRCLE ( 'NONE', #18528, 0.5000000000000004441 ) ;
#13333=ORIENTED_EDGE ( 'NONE', *, *, #14389, .F. ) ;
#13336=ORIENTED_EDGE ( 'NONE', *, *, #20700, .F. ) ;
#13338=CARTESIAN_POINT ( 'NONE',  ( -5.537946624085887670, 36.44027069998197277, 7.000000000000000000 ) ) ;
#13342=ADVANCED_FACE ( 'NONE', ( #1360 ), #1215, .T. ) ;
#13344=EDGE_LOOP ( 'NONE', ( #12436, #32560, #35741, #198 ) ) ;
#13345=EDGE_LOOP ( 'NONE', ( #25330, #20796, #38435 ) ) ;
#13349=CIRCLE ( 'NONE', #27626, 6.000000000000005329 ) ;
#13355=CIRCLE ( 'NONE', #25682, 0.5000000000000012212 ) ;
#13356=CYLINDRICAL_SURFACE ( 'NONE', #17576, 0.5000000000000004441 ) ;
#13357=FACE_OUTER_BOUND ( 'NONE', #3447, .T. ) ;
#13360=CARTESIAN_POINT ( 'NONE',  ( 2.618397918551820247, 7.776539141412873946, 10.76099332938164110 ) ) ;
#13366=CARTESIAN_POINT ( 'NONE',  ( -8.007761790012255076, 9.776959832083379709, 7.000000000000000000 ) ) ;
#13367=CARTESIAN_POINT ( 'NONE',  ( 13.94482798346721175, 26.50521816028912525, 7.000000000000000000 ) ) ;
#13370=CARTESIAN_POINT ( 'NONE',  ( -10.06946225350398194, 32.23940090176283491, 10.00000000000000000 ) ) ;
#13373=CARTESIAN_POINT ( 'NONE',  ( 0.000000000000000000, 0.000000000000000000, 11.00000000000000000 ) ) ;
#13382=CIRCLE ( 'NONE', #25697, 1.000000000000000888 ) ;
#13383=AXIS2_PLACEMENT_3D ( 'NONE', #24473, #12083, #3335 ) ;
#13384=CARTESIAN_POINT ( 'NONE',  ( 14.97009266215791889, 21.42933399866927857, 10.49999999999999822 ) ) ;
#13385=ORIENTED_EDGE ( 'NONE', *, *, #6640, .F. ) ;
#13387=DIRECTION ( 'NONE',  ( 0.7431448254773863615, -0.6691306063588671194, 0.000000000000000000 ) ) ;
#13388=VECTOR ( 'NONE', #17149, 1000.000000000000000 ) ;
#13389=DIRECTION ( 'NONE',  ( 1.224646799147351235E-16, -1.000000000000000000, -0.000000000000000000 ) ) ;
#13390=VERTEX_POINT ( 'NONE', #3701 ) ;
#13392=FACE_OUTER_BOUND ( 'NONE', #29133, .T. ) ;
#13395=EDGE_CURVE ( 'NONE', #33406, #29912, #3808, .T. ) ;
#13396=ORIENTED_EDGE ( 'NONE', *, *, #7990, .F. ) ;
#13399=DIRECTION ( 'NONE',  ( 0.000000000000000000, 0.000000000000000000, -1.000000000000000000 ) ) ;
#13400=CARTESIAN_POINT ( 'NONE',  ( -4.244684691011856081, 8.112536183716212435, 7.202682876670047918 ) ) ;
#13402=CARTESIAN_POINT ( 'NONE',  ( 5.068835528549735514, 13.82204480395803081, 10.49999999999999822 ) ) ;
#13403=ORIENTED_EDGE ( 'NONE', *, *, #29999, .F. ) ;
#13406=DIRECTION ( 'NONE',  ( 1.000000000000000000, 0.000000000000000000, 0.000000000000000000 ) ) ;
#13407=DIRECTION ( 'NONE',  ( -1.000000000000000000, 0.000000000000000000, 0.000000000000000000 ) ) ;
#13409=AXIS2_PLACEMENT_3D ( 'NONE', #18007, #12098, #24289 ) ;
#13411=VERTEX_POINT ( 'NONE', #25237 ) ;
#13412=CARTESIAN_POINT ( 'NONE',  ( -10.14060191828654034, 25.26915018278948111, 10.00000000000000000 ) ) ;
#13423=ORIENTED_EDGE ( 'NONE', *, *, #16600, .T. ) ;
#13424=ORIENTED_EDGE ( 'NONE', *, *, #2018, .T. ) ;
#13427=CARTESIAN_POINT ( 'NONE',  ( -14.86556419889029534, 20.43481210330121556, 10.49999999999999822 ) ) ;
#13430=VERTEX_POINT ( 'NONE', #7340 ) ;
#13432=CARTESIAN_POINT ( 'NONE',  ( 14.06932099033143757, 26.54566839026256631, 11.00000000000000355 ) ) ;
#13433=FACE_OUTER_BOUND ( 'NONE', #32690, .T. ) ;
#13434=VERTEX_POINT ( 'NONE', #38634 ) ;
#13436=CARTESIAN_POINT ( 'NONE',  ( -5.238409041734074734, 36.41108174777520645, 10.49999999999999822 ) ) ;
#13437=ORIENTED_EDGE ( 'NONE', *, *, #5617, .T. ) ;
#13443=EDGE_CURVE ( 'NONE', #22657, #21143, #32140, .T. ) ;
#13446=VECTOR ( 'NONE', #36139, 1000.000000000000000 ) ;
#13449=DIRECTION ( 'NONE',  ( 0.4156269377774580720, 0.5720614028176809196, -0.7071067811865475727 ) ) ;
#13450=DIRECTION ( 'NONE',  ( -0.7431448254773862505, 0.6691306063588670083, 0.000000000000000000 ) ) ;
#13452=CARTESIAN_POINT ( 'NONE',  ( -11.11016527260153097, 31.83082137946489354, 11.00000000000000000 ) ) ;
#13456=CARTESIAN_POINT ( 'NONE',  ( -0.5000000000000004441, 36.00000000000000711, 9.500000000000000000 ) ) ;
#13459=CIRCLE ( 'NONE', #22537, 6.000000000000013323 ) ;
#13460=ORIENTED_EDGE ( 'NONE', *, *, #32277, .F. ) ;
#13462=AXIS2_PLACEMENT_3D ( 'NONE', #3149, #27729, #30789 ) ;
#13464=EDGE_CURVE ( 'NONE', #10797, #8399, #23195, .T. ) ;
#13465=CARTESIAN_POINT ( 'NONE',  ( 8.927394655428274817, 11.06314620770945290, 11.00000000000000000 ) ) ;
#13467=ORIENTED_EDGE ( 'NONE', *, *, #32019, .F. ) ;
#13469=CARTESIAN_POINT ( 'NONE',  ( -5.644276917315534270, 36.40655018617698602, 10.49999999999999822 ) ) ;
#13471=AXIS2_PLACEMENT_3D ( 'NONE', #24895, #12107, #9667 ) ;
#13473=CARTESIAN_POINT ( 'NONE',  ( -14.97009266215794021, 21.42933399866948463, 10.49999999999999822 ) ) ;
#13475=LINE ( 'NONE', #22819, #27027 ) ;
#13477=ORIENTED_EDGE ( 'NONE', *, *, #17243, .F. ) ;
#13480=DIRECTION ( 'NONE',  ( 1.000000000000000000, 0.000000000000000000, 0.000000000000000000 ) ) ;
#13484=FACE_OUTER_BOUND ( 'NONE', #20710, .T. ) ;
#13490=VERTEX_POINT ( 'NONE', #35184 ) ;
#13491=EDGE_CURVE ( 'NONE', #26306, #18033, #31708, .T. ) ;
#13493=DIRECTION ( 'NONE',  ( 0.000000000000000000, 0.000000000000000000, 1.000000000000000000 ) ) ;
#13495=AXIS2_PLACEMENT_3D ( 'NONE', #30738, #21388, #33795 ) ;
#13496=DIRECTION ( 'NONE',  ( 0.000000000000000000, 0.000000000000000000, -1.000000000000000000 ) ) ;
#13497=EDGE_CURVE ( 'NONE', #13434, #23843, #16296, .T. ) ;
#13499=AXIS2_PLACEMENT_3D ( 'NONE', #35843, #2324, #1929 ) ;
#13500=AXIS2_PLACEMENT_3D ( 'NONE', #19481, #32497, #1406 ) ;
#13501=DIRECTION ( 'NONE',  ( 0.4067366430758009299, 0.9135454576426006446, 0.000000000000000000 ) ) ;
#13502=PLANE ( 'NONE',  #4794 ) ;
#13503=CARTESIAN_POINT ( 'NONE',  ( -13.32151712420406398, 20.09434385051854122, 9.500000000000000000 ) ) ;
#13505=CARTESIAN_POINT ( 'NONE',  ( -6.354454053420247384, 35.54304081427990525, 10.99999999999999289 ) ) ;
#13508=CARTESIAN_POINT ( 'NONE',  ( -7.014595103779441843, 35.79644522156330311, 11.00000000000000000 ) ) ;
#13509=CARTESIAN_POINT ( 'NONE',  ( 13.46929972531963848, 26.35070966310165375, 7.500000000000000000 ) ) ;
#13511=CARTESIAN_POINT ( 'NONE',  ( -6.980762143445979895, 14.59310681135558241, 11.00000000000000000 ) ) ;
#13512=ORIENTED_EDGE ( 'NONE', *, *, #15353, .T. ) ;
#13517=EDGE_CURVE ( 'NONE', #32632, #5452, #32348, .T. ) ;
#13520=ORIENTED_EDGE ( 'NONE', *, *, #11173, .F. ) ;
#13522=ORIENTED_EDGE ( 'NONE', *, *, #7253, .T. ) ;
#13524=DIRECTION ( 'NONE',  ( 1.000000000000000000, 0.000000000000000000, 0.000000000000000000 ) ) ;
#13527=AXIS2_PLACEMENT_3D ( 'NONE', #7651, #38736, #29589 ) ;
#13528=AXIS2_PLACEMENT_3D ( 'NONE', #16420, #22704, #19460 ) ;
#13535=CARTESIAN_POINT ( 'NONE',  ( -12.37185181069348161, 14.01743714881896530, 7.203056206335839207 ) ) ;
#13538=ORIENTED_EDGE ( 'NONE', *, *, #21533, .F. ) ;
#13540=CARTESIAN_POINT ( 'NONE',  ( -14.11133924723977628, 27.61078317377193869, 10.50000000000000000 ) ) ;
#13541=ORIENTED_EDGE ( 'NONE', *, *, #30308, .F. ) ;
#13543=FACE_OUTER_BOUND ( 'NONE', #33439, .T. ) ;
#13544=EDGE_CURVE ( 'NONE', #24143, #13849, #21964, .T. ) ;
#13547=ORIENTED_EDGE ( 'NONE', *, *, #29005, .F. ) ;
#13549=FACE_OUTER_BOUND ( 'NONE', #4661, .T. ) ;
#13550=CYLINDRICAL_SURFACE ( 'NONE', #7152, 0.5000000000000004441 ) ;
#13551=VECTOR ( 'NONE', #39651, 1000.000000000000000 ) ;
#13552=CIRCLE ( 'NONE', #33046, 1.000000000000004441 ) ;
#13553=CARTESIAN_POINT ( 'NONE',  ( 0.000000000000000000, 22.50000000000000355, 7.000000000000000000 ) ) ;
#13556=CARTESIAN_POINT ( 'NONE',  ( -13.77067693704740492, 28.44713853003868564, 7.000000000000000000 ) ) ;
#13557=CARTESIAN_POINT ( 'NONE',  ( -10.04974741695039242, 22.44923726269184527, 10.49999999999999467 ) ) ;
#13558=VECTOR ( 'NONE', #4312, 1000.000000000000000 ) ;
#13559=CARTESIAN_POINT ( 'NONE',  ( -3.153820973115282644, 32.04219121950185212, 10.50000000000000533 ) ) ;
#13560=DIRECTION ( 'NONE',  ( -0.07391278520355981652, 0.7032331762534046460, 0.7071067811865479058 ) ) ;
#13561=CARTESIAN_POINT ( 'NONE',  ( -9.911438049898041669, 11.24107483890965575, 7.000000000000000000 ) ) ;
#13564=VERTEX_POINT ( 'NONE', #12377 ) ;
#13566=CARTESIAN_POINT ( 'NONE',  ( -7.611215932167763043, 18.68301270189229513, 9.000000000000001776 ) ) ;
#13569=CARTESIAN_POINT ( 'NONE',  ( 12.49038105676654276, 14.13397459621550389, 10.49999999999999822 ) ) ;
#13573=ADVANCED_FACE ( 'NONE', ( #393 ), #15827, .F. ) ;
#13579=CARTESIAN_POINT ( 'NONE',  ( 5.092030333742720849, 36.31140934042893065, 10.49999999999999822 ) ) ;
#13584=FACE_OUTER_BOUND ( 'NONE', #10499, .T. ) ;
#13588=FACE_OUTER_BOUND ( 'NONE', #9547, .T. ) ;
#13589=VECTOR ( 'NONE', #13804, 1000.000000000000114 ) ;
#13591=ORIENTED_EDGE ( 'NONE', *, *, #4282, .F. ) ;
#13593=EDGE_CURVE ( 'NONE', #29442, #12596, #28014, .T. ) ;
#13596=EDGE_CURVE ( 'NONE', #22179, #15406, #4458, .T. ) ;
#13597=ORIENTED_EDGE ( 'NONE', *, *, #10777, .T. ) ;
#13600=FACE_OUTER_BOUND ( 'NONE', #24152, .T. ) ;
#13601=CARTESIAN_POINT ( 'NONE',  ( -4.475131784526824141, 8.183115020678636498, 7.000000000000000000 ) ) ;
#13605=ORIENTED_EDGE ( 'NONE', *, *, #25974, .T. ) ;
#13606=( LENGTH_UNIT ( ) NAMED_UNIT ( * ) SI_UNIT ( .MILLI., .METRE. ) );
#13607=CARTESIAN_POINT ( 'NONE',  ( 7.618377661053323813, 10.47536095541698486, 7.500000000000000888 ) ) ;
#13608=LINE ( 'NONE', #38798, #13068 ) ;
#13609=FACE_OUTER_BOUND ( 'NONE', #2905, .T. ) ;
#13612=VECTOR ( 'NONE', #3321, 1000.000000000000114 ) ;
#13613=ORIENTED_EDGE ( 'NONE', *, *, #33112, .T. ) ;
#13618=AXIS2_PLACEMENT_3D ( 'NONE', #33907, #16209, #22891 ) ;
#13619=EDGE_CURVE ( 'NONE', #15223, #11176, #37565, .T. ) ;
#13620=DIRECTION ( 'NONE',  ( 0.000000000000000000, 0.000000000000000000, 1.000000000000000000 ) ) ;
#13621=EDGE_CURVE ( 'NONE', #5398, #16864, #20364, .T. ) ;
#13622=ORIENTED_EDGE ( 'NONE', *, *, #14285, .T. ) ;
#13626=CYLINDRICAL_SURFACE ( 'NONE', #28289, 0.5000000000000004441 ) ;
#13628=B_SPLINE_CURVE_WITH_KNOTS ( 'NONE', 3,
 ( #5026, #38954, #26759, #19870, #35713, #29003 ),
 .UNSPECIFIED., .F., .F.,
 ( 4, 2, 4 ),
 ( 0.3999999999265801964, 0.6999999999632900982, 1.000000000000000000 ),
 .UNSPECIFIED. ) ;
#13629=ORIENTED_EDGE ( 'NONE', *, *, #17865, .F. ) ;
#13631=CARTESIAN_POINT ( 'NONE',  ( -6.354454053420242943, 35.54304081427989814, 11.00000000000000000 ) ) ;
#13634=CARTESIAN_POINT ( 'NONE',  ( -8.927394655428429360, 11.06314620770957013, 9.000000000000001776 ) ) ;
#13637=DIRECTION ( 'NONE',  ( 0.5877852522924690293, -0.8090169943749503378, 0.000000000000000000 ) ) ;
#13638=CARTESIAN_POINT ( 'NONE',  ( 14.92615392307456368, 21.72537115092769611, 10.49999999999999467 ) ) ;
#13639=UNCERTAINTY_MEASURE_WITH_UNIT (LENGTH_MEASURE( 1.000000000000000082E-05 ), #26344, 'distance_accuracy_value', 'NONE');
#13640=VERTEX_POINT ( 'NONE', #6866 ) ;
#13642=CARTESIAN_POINT ( 'NONE',  ( -5.305271391458861174, 36.43775379931907565, 10.49999999999999822 ) ) ;
#13643=ADVANCED_FACE ( 'NONE', ( #34516 ), #23283, .T. ) ;
#13644=ORIENTED_EDGE ( 'NONE', *, *, #14361, .T. ) ;
#13646=DIRECTION ( 'NONE',  ( -0.5877852522924796874, -0.8090169943749426773, 0.000000000000000000 ) ) ;
#13649=VERTEX_POINT ( 'NONE', #37961 ) ;
#13652=DIRECTION ( 'NONE',  ( -2.168404344971006896E-16, 1.000000000000000000, 0.000000000000000000 ) ) ;
#13654=CARTESIAN_POINT ( 'NONE',  ( 11.94134295108990074, 16.18301270189217433, 9.500000000000000000 ) ) ;
#13655=CARTESIAN_POINT ( 'NONE',  ( -3.610593701936585909, 31.83882289796395426, 10.50000000000000888 ) ) ;
#13656=VECTOR ( 'NONE', #3115, 999.9999999999998863 ) ;
#13657=CARTESIAN_POINT ( 'NONE',  ( -8.238488885696254371, 24.65111619403957022, 7.000000000000000000 ) ) ;
#13659=VECTOR ( 'NONE', #25301, 1000.000000000000000 ) ;
#13662=CARTESIAN_POINT ( 'NONE',  ( -14.45538749008468038, 26.50521816028845734, 7.489440493383480835 ) ) ;
#13664=ORIENTED_EDGE ( 'NONE', *, *, #22736, .T. ) ;
#13667=CARTESIAN_POINT ( 'NONE',  ( 10.81260707898150386, 32.90853150812155548, 10.49999999999999822 ) ) ;
#13669=ORIENTED_EDGE ( 'NONE', *, *, #27618, .F. ) ;
#13672=DIRECTION ( 'NONE',  ( 0.4731467892558179900, 0.5254827454987496260, -0.7071067811865524577 ) ) ;
#13673=CIRCLE ( 'NONE', #24066, 1.000000000000004441 ) ;
#13674=EDGE_LOOP ( 'NONE', ( #12640, #28464, #4141, #38378 ) ) ;
#13676=DIRECTION ( 'NONE',  ( 0.000000000000000000, 0.000000000000000000, -1.000000000000000000 ) ) ;
#13678=CARTESIAN_POINT ( 'NONE',  ( 13.58398418571186816, 16.13684478916777820, 7.102637441331451029 ) ) ;
#13679=ORIENTED_EDGE ( 'NONE', *, *, #23257, .F. ) ;
#13682=CARTESIAN_POINT ( 'NONE',  ( 14.36830325120613594, 20.48707633493483371, 9.000000000000001776 ) ) ;
#13684=ORIENTED_EDGE ( 'NONE', *, *, #32693, .T. ) ;
#13686=DIRECTION ( 'NONE',  ( -0.000000000000000000, -0.000000000000000000, -1.000000000000000000 ) ) ;
#13688=EDGE_LOOP ( 'NONE', ( #6296, #21525, #39014, #24223, #16580, #29436, #32013, #33040, #6978, #11752, #21024, #35094, #24463, #14031, #21149, #6891, #4305, #15647, #19092, #7277, #3153, #24922, #26956, #19218, #19558, #27014, #32044, #2888, #26281, #37455, #6594, #20990, #3161, #34884, #5454, #35886, #26608, #20237, #18206, #31972, #14532, #17950, #30605, #14898, #5797, #8260, #6062, #8833, #13264, #13888, #11043, #2176, #28537, #28420, #14401, #37684, #1123, #28534, #16482, #3266, #29640, #35105 ) ) ;
#13693=VECTOR ( 'NONE', #661, 1000.000000000000000 ) ;
#13694=VERTEX_POINT ( 'NONE', #15428 ) ;
#13697=LINE ( 'NONE', #32406, #16709 ) ;
#13698=CARTESIAN_POINT ( 'NONE',  ( -14.47283171447380390, 21.48159823030330884, 7.000000000000000000 ) ) ;
#13699=EDGE_CURVE ( 'NONE', #37009, #15678, #9361, .T. ) ;
#13701=CARTESIAN_POINT ( 'NONE',  ( -11.58426073497328801, 31.66040656113770169, 10.49999999999999822 ) ) ;
#13703=DIRECTION ( 'NONE',  ( -0.9135454576426004225, 0.4067366430758009854, 0.000000000000000000 ) ) ;
#13704=VERTEX_POINT ( 'NONE', #18680 ) ;
#13705=DIRECTION ( 'NONE',  ( 0.8660254037844364872, -0.5000000000000038858, 0.000000000000000000 ) ) ;
#13706=DIRECTION ( 'NONE',  ( -0.7431448254773862505, 0.6691306063588672304, -0.000000000000000000 ) ) ;
#13709=CARTESIAN_POINT ( 'NONE',  ( -2.317734025672945286, 9.191051544684766483, 10.50000000000000000 ) ) ;
#13716=CONICAL_SURFACE ( 'NONE', #27269, 0.4999999999999947264, 0.7853981633974479459 ) ;
#13721=EDGE_LOOP ( 'NONE', ( #32784, #21173, #37393, #35181, #37844, #38957 ) ) ;
#13723=ORIENTED_EDGE ( 'NONE', *, *, #16513, .T. ) ;
#13725=CARTESIAN_POINT ( 'NONE',  ( 8.118377661053333583, 10.47536095541699197, 11.00000000000000000 ) ) ;
#13731=EDGE_CURVE ( 'NONE', #17829, #23066, #39277, .T. ) ;
#13732=VERTEX_POINT ( 'NONE', #28213 ) ;
#13735=VECTOR ( 'NONE', #36980, 1000.000000000000000 ) ;
#13737=EDGE_CURVE ( 'NONE', #34838, #36944, #32358, .T. ) ;
#13741=FACE_OUTER_BOUND ( 'NONE', #8088, .T. ) ;
#13748=EDGE_CURVE ( 'NONE', #21064, #9701, #188, .T. ) ;
#13750=ADVANCED_FACE ( 'NONE', ( #3630 ), #588, .T. ) ;
#13751=CYLINDRICAL_SURFACE ( 'NONE', #16502, 6.000000000000004441 ) ;
#13752=DIRECTION ( 'NONE',  ( -1.000000000000000000, 0.000000000000000000, 0.000000000000000000 ) ) ;
#13756=CARTESIAN_POINT ( 'NONE',  ( -9.221287281574669592, 10.65863771052209863, 10.50000000000000000 ) ) ;
#13757=DIRECTION ( 'NONE',  ( 1.000000000000000000, 0.000000000000000000, 0.000000000000000000 ) ) ;
#13758=CIRCLE ( 'NONE', #134, 0.5000000000000004441 ) ;
#13759=LINE ( 'NONE', #26756, #30974 ) ;
#13760=CARTESIAN_POINT ( 'NONE',  ( -15.02235689379176620, 21.92659494635362449, 10.49999999999999467 ) ) ;
#13761=DIRECTION ( 'NONE',  ( -0.2079116908177533751, 0.9781476007338069101, 0.000000000000000000 ) ) ;
#13764=ORIENTED_EDGE ( 'NONE', *, *, #8732, .T. ) ;
#13765=AXIS2_PLACEMENT_3D ( 'NONE', #12289, #12483, #24877 ) ;
#13767=DIRECTION ( 'NONE',  ( 0.6216356077939706459, 0.000000000000000000, 0.7833065626704660556 ) ) ;
#13769=AXIS2_PLACEMENT_3D ( 'NONE', #33416, #11667, #21203 ) ;
#13771=FACE_OUTER_BOUND ( 'NONE', #30015, .T. ) ;
#13774=EDGE_CURVE ( 'NONE', #14341, #31871, #8347, .T. ) ;
#13777=CONICAL_SURFACE ( 'NONE', #4027, 1.000000000000006883, 0.7853981633974549403 ) ;
#13781=DIRECTION ( 'NONE',  ( 0.000000000000000000, 0.000000000000000000, 1.000000000000000000 ) ) ;
#13783=ORIENTED_EDGE ( 'NONE', *, *, #34955, .T. ) ;
#13787=CARTESIAN_POINT ( 'NONE',  ( 21.39877161664088590, 15.54711762656346075, 7.000000000000000000 ) ) ;
#13788=ORIENTED_EDGE ( 'NONE', *, *, #5548, .T. ) ;
#13789=LINE ( 'NONE', #26181, #36237 ) ;
#13790=AXIS2_PLACEMENT_3D ( 'NONE', #29687, #5497, #10806 ) ;
#13791=CARTESIAN_POINT ( 'NONE',  ( -7.309360666678539786, 9.887575703124607429, 7.000000000000000000 ) ) ;
#13792=EDGE_LOOP ( 'NONE', ( #18991, #7159, #13783 ) ) ;
#13796=VECTOR ( 'NONE', #16285, 1000.000000000000000 ) ;
#13801=DIRECTION ( 'NONE',  ( 0.000000000000000000, 0.000000000000000000, -1.000000000000000000 ) ) ;
#13802=DIRECTION ( 'NONE',  ( -0.1045284632676563991, -0.9945218953682730678, 0.000000000000000000 ) ) ;
#13804=DIRECTION ( 'NONE',  ( -0.5877852522924690293, 0.8090169943749503378, 0.000000000000000000 ) ) ;
#13807=CARTESIAN_POINT ( 'NONE',  ( 19.48557158514997667, 33.74999999999982236, 7.000000000000000000 ) ) ;
#13808=CARTESIAN_POINT ( 'NONE',  ( 13.49038105676655164, 15.86602540378438064, 10.50000000000000178 ) ) ;
#13810=CIRCLE ( 'NONE', #13140, 0.5000000000000000000 ) ;
#13813=DIRECTION ( 'NONE',  ( -1.000000000000000000, 0.000000000000000000, 0.000000000000000000 ) ) ;
#13814=CARTESIAN_POINT ( 'NONE',  ( -1.000000000000000000, 37.00000000000000711, 7.000000000000000000 ) ) ;
#13819=ORIENTED_EDGE ( 'NONE', *, *, #18917, .T. ) ;
#13825=CARTESIAN_POINT ( 'NONE',  ( -10.44103466624267185, 32.57396620494226624, 7.000000000000000000 ) ) ;
#13829=DIRECTION ( 'NONE',  ( -1.000000000000000000, 0.000000000000000000, 0.000000000000000000 ) ) ;
#13830=AXIS2_PLACEMENT_3D ( 'NONE', #12517, #19404, #31595 ) ;
#13835=VERTEX_POINT ( 'NONE', #29220 ) ;
#13837=PLANE ( 'NONE',  #25804 ) ;
#13838=DIRECTION ( 'NONE',  ( 0.4067366430757889395, -0.9135454576426058626, 0.000000000000000000 ) ) ;
#13839=DIRECTION ( 'NONE',  ( -0.9945218953682742891, -0.1045284632676437425, 0.000000000000000000 ) ) ;
#13843=DIRECTION ( 'NONE',  ( 1.000000000000000000, 0.000000000000000000, 0.000000000000000000 ) ) ;
#13844=ORIENTED_EDGE ( 'NONE', *, *, #36602, .F. ) ;
#13849=VERTEX_POINT ( 'NONE', #1390 ) ;
#13852=ADVANCED_FACE ( 'NONE', ( #10735 ), #23120, .F. ) ;
#13855=DIRECTION ( 'NONE',  ( -0.000000000000000000, 0.000000000000000000, 1.000000000000000000 ) ) ;
#13856=ADVANCED_FACE ( 'NONE', ( #29620 ), #7878, .F. ) ;
#13859=FACE_OUTER_BOUND ( 'NONE', #27057, .T. ) ;
#13860=FACE_OUTER_BOUND ( 'NONE', #23719, .T. ) ;
#13861=B_SPLINE_CURVE_WITH_KNOTS ( 'NONE', 3,
 ( #8871, #39345, #24503, #2581, #39937, #8673 ),
 .UNSPECIFIED., .F., .F.,
 ( 4, 2, 4 ),
 ( 0.000000000000000000, 0.5000000000000000000, 1.000000000000000000 ),
 .UNSPECIFIED. ) ;
#13863=CARTESIAN_POINT ( 'NONE',  ( -12.80736835487442349, 15.68301270189233954, 7.000000000000000000 ) ) ;
#13864=AXIS2_PLACEMENT_3D ( 'NONE', #13863, #11223, #7764 ) ;
#13868=CARTESIAN_POINT ( 'NONE',  ( -13.63581098909220302, 27.45627467658446719, 11.00000000000000000 ) ) ;
#13869=CARTESIAN_POINT ( 'NONE',  ( -13.20348688925211178, 15.99217894729804534, 10.49999999999999822 ) ) ;
#13873=VERTEX_POINT ( 'NONE', #4025 ) ;
#13877=PRODUCT_DEFINITION_FORMATION_WITH_SPECIFIED_SOURCE ( 'ANY', '', #3190, .NOT_KNOWN. ) ;
#13878=CARTESIAN_POINT ( 'NONE',  ( 3.713592597587160871, 7.966960743906808418, 7.499999999999990230 ) ) ;
#13882=ORIENTED_EDGE ( 'NONE', *, *, #842, .T. ) ;
#13888=ORIENTED_EDGE ( 'NONE', *, *, #26921, .F. ) ;
#13893=ORIENTED_EDGE ( 'NONE', *, *, #34978, .T. ) ;
#13895=DIRECTION ( 'NONE',  ( 0.5000000000000038858, 0.8660254037844363761, -0.000000000000000000 ) ) ;
#13896=CARTESIAN_POINT ( 'NONE',  ( -13.87104230352201917, 20.53934056656885687, 7.500000000000004441 ) ) ;
#13900=AXIS2_PLACEMENT_3D ( 'NONE', #16623, #19654, #19453 ) ;
#13902=VERTEX_POINT ( 'NONE', #10330 ) ;
#13905=VECTOR ( 'NONE', #14062, 1000.000000000000114 ) ;
#13907=PLANE ( 'NONE',  #34283 ) ;
#13908=VECTOR ( 'NONE', #1628, 1000.000000000000000 ) ;
#13909=LINE ( 'NONE', #1932, #19476 ) ;
#13910=CARTESIAN_POINT ( 'NONE',  ( 6.407695755496777501, 35.66262363504857547, 11.00000000000000000 ) ) ;
#13912=ORIENTED_EDGE ( 'NONE', *, *, #1153, .T. ) ;
#13913=DIRECTION ( 'NONE',  ( -1.000000000000000000, 0.000000000000000000, 0.000000000000000000 ) ) ;
#13914=FACE_OUTER_BOUND ( 'NONE', #8586, .T. ) ;
#13916=DIRECTION ( 'NONE',  ( -0.000000000000000000, -0.000000000000000000, -1.000000000000000000 ) ) ;
#13917=DIRECTION ( 'NONE',  ( -0.7032331762534058672, -0.07391278520355742954, -0.7071067811865467956 ) ) ;
#13920=ORIENTED_EDGE ( 'NONE', *, *, #18962, .T. ) ;
#13924=DIRECTION ( 'NONE',  ( 0.000000000000000000, 0.000000000000000000, 1.000000000000000000 ) ) ;
#13936=ORIENTED_EDGE ( 'NONE', *, *, #10619, .F. ) ;
#13939=CARTESIAN_POINT ( 'NONE',  ( -10.33795143809923545, 20.40792924032147226, 10.49999999999999467 ) ) ;
#13940=CARTESIAN_POINT ( 'NONE',  ( 2.362621116368220697, 8.178251995481296888, 10.83333333333333037 ) ) ;
#13941=CONICAL_SURFACE ( 'NONE', #32122, 1.000000000000007772, 0.7853981633974560506 ) ;
#13946=ORIENTED_EDGE ( 'NONE', *, *, #22554, .T. ) ;
#13948=LINE ( 'NONE', #1978, #2491 ) ;
#13952=EDGE_CURVE ( 'NONE', #3918, #32089, #38789, .T. ) ;
#13954=DIRECTION ( 'NONE',  ( 0.000000000000000000, -0.6216356077939594327, -0.7833065626704749373 ) ) ;
#13955=DIRECTION ( 'NONE',  ( -5.095851118916442708E-15, -0.7071067811865500152, -0.7071067811865451302 ) ) ;
#13956=CIRCLE ( 'NONE', #22383, 6.000000000000000000 ) ;
#13957=CARTESIAN_POINT ( 'NONE',  ( 0.000000000000000000, 22.50000000000000355, 7.000000000000000000 ) ) ;
#13959=EDGE_CURVE ( 'NONE', #17177, #12432, #12911, .T. ) ;
#13962=CARTESIAN_POINT ( 'NONE',  ( 13.63581098909226519, 27.45627467658428600, 11.00000000000000000 ) ) ;
#13969=CARTESIAN_POINT ( 'NONE',  ( -12.30736835487443415, 14.81698729810790560, 11.00000000000000000 ) ) ;
#13973=CARTESIAN_POINT ( 'NONE',  ( 9.677076426724163127, 26.69573495723207657, 10.50000000000000533 ) ) ;
#13985=LINE ( 'NONE', #4643, #18017 ) ;
#13986=ADVANCED_FACE ( 'NONE', ( #26978 ), #5633, .F. ) ;
#13987=ORIENTED_EDGE ( 'NONE', *, *, #24933, .T. ) ;
#13989=ORIENTED_EDGE ( 'NONE', *, *, #3692, .F. ) ;
#13990=CARTESIAN_POINT ( 'NONE',  ( 7.096882951594523981, 29.56287847632726695, 10.49999999999999645 ) ) ;
#13991=ORIENTED_EDGE ( 'NONE', *, *, #32821, .T. ) ;
#13992=CARTESIAN_POINT ( 'NONE',  ( 12.74038105676654453, 14.56698729810772264, 7.000000000000000000 ) ) ;
#13994=VERTEX_POINT ( 'NONE', #27574 ) ;
#13995=VECTOR ( 'NONE', #4121, 1000.000000000000000 ) ;
#13997=ORIENTED_EDGE ( 'NONE', *, *, #30912, .T. ) ;
#13999=VECTOR ( 'NONE', #16626, 1000.000000000000227 ) ;
#14001=ORIENTED_EDGE ( 'NONE', *, *, #16587, .T. ) ;
#14002=CARTESIAN_POINT ( 'NONE',  ( -10.06946225350398372, 32.23940090176283491, 7.500000000000005329 ) ) ;
#14003=VERTEX_POINT ( 'NONE', #18241 ) ;
#14004=CARTESIAN_POINT ( 'NONE',  ( 11.44473057578109199, 31.45924896672603310, 9.500000000000000000 ) ) ;
#14005=LINE ( 'NONE', #19906, #16897 ) ;
#14006=EDGE_CURVE ( 'NONE', #11050, #18136, #23930, .T. ) ;
#14008=DIRECTION ( 'NONE',  ( -0.7431448254773846962, 0.6691306063588690067, 0.000000000000000000 ) ) ;
#14010=SURFACE_STYLE_USAGE ( .BOTH. , #28847 ) ;
#14013=DIRECTION ( 'NONE',  ( -0.000000000000000000, -0.000000000000000000, -1.000000000000000000 ) ) ;
#14016=VERTEX_POINT ( 'NONE', #36727 ) ;
#14017=CARTESIAN_POINT ( 'NONE',  ( 10.44103466624280685, 32.57396620494213124, 7.499999999999997335 ) ) ;
#14018=CYLINDRICAL_SURFACE ( 'NONE', #17524, 0.5000000000000004441 ) ;
#14022=ORIENTED_EDGE ( 'NONE', *, *, #22281, .F. ) ;
#14024=CONICAL_SURFACE ( 'NONE', #13383, 1.000000000000007772, 0.7853981633974554954 ) ;
#14029=ADVANCED_FACE ( 'NONE', ( #8081 ), #33291, .F. ) ;
#14030=ORIENTED_EDGE ( 'NONE', *, *, #19454, .T. ) ;
#14031=ORIENTED_EDGE ( 'NONE', *, *, #18718, .F. ) ;
#14033=CARTESIAN_POINT ( 'NONE',  ( 14.99905852611806267, 22.33194247983193392, 7.000000000000000000 ) ) ;
#14037=EDGE_LOOP ( 'NONE', ( #33094, #17193, #22632, #1459, #9380 ) ) ;
#14040=FACE_OUTER_BOUND ( 'NONE', #38508, .T. ) ;
#14041=DIRECTION ( 'NONE',  ( -0.4067366430757888285, 0.9135454576426059736, -0.000000000000000000 ) ) ;
#14044=FACE_OUTER_BOUND ( 'NONE', #16655, .T. ) ;
#14045=VERTEX_POINT ( 'NONE', #20491 ) ;
#14052=EDGE_CURVE ( 'NONE', #22956, #18136, #18043, .T. ) ;
#14054=AXIS2_PLACEMENT_3D ( 'NONE', #19778, #13676, #26064 ) ;
#14059=DIRECTION ( 'NONE',  ( -0.4067366430757891060, 0.9135454576426058626, 0.000000000000000000 ) ) ;
#14062=DIRECTION ( 'NONE',  ( -0.3090169943749448977, 0.9510565162951543083, -0.000000000000000000 ) ) ;
#14067=ORIENTED_EDGE ( 'NONE', *, *, #29147, .F. ) ;
#14070=CARTESIAN_POINT ( 'NONE',  ( -14.38243823352021522, 26.25560849141445274, 10.49999999999999822 ) ) ;
#14072=EDGE_LOOP ( 'NONE', ( #21933, #12005, #32209, #21489 ) ) ;
#14077=ADVANCED_FACE ( 'NONE', ( #17851 ), #32885, .T. ) ;
#14079=CARTESIAN_POINT ( 'NONE',  ( 13.63396663385386454, 16.24580510161703728, 7.000000000000000000 ) ) ;
#14081=AXIS2_PLACEMENT_3D ( 'NONE', #39917, #11703, #27337 ) ;
#14082=VECTOR ( 'NONE', #39767, 999.9999999999998863 ) ;
#14088=ORIENTED_EDGE ( 'NONE', *, *, #13100, .T. ) ;
#14090=CARTESIAN_POINT ( 'NONE',  ( -8.412270287199616448, 10.07085245822954533, 10.59344459855563336 ) ) ;
#14092=AXIS2_PLACEMENT_3D ( 'NONE', #1812, #35739, #30449 ) ;
#14093=VERTEX_POINT ( 'NONE', #24330 ) ;
#14096=AXIS2_PLACEMENT_3D ( 'NONE', #19010, #15761, #36905 ) ;
#14098=EDGE_LOOP ( 'NONE', ( #2023, #40114, #7821 ) ) ;
#14101=EDGE_CURVE ( 'NONE', #35217, #10337, #33616, .T. ) ;
#14102=LINE ( 'NONE', #29546, #34916 ) ;
#14103=DIRECTION ( 'NONE',  ( 0.1045284632676569680, 0.9945218953682730678, -0.000000000000000000 ) ) ;
#14105=CIRCLE ( 'NONE', #31656, 0.9999999999999991118 ) ;
#14108=DIRECTION ( 'NONE',  ( -0.1045284632676437842, 0.9945218953682744001, 0.000000000000000000 ) ) ;
#14109=DIRECTION ( 'NONE',  ( 0.000000000000000000, 1.000000000000000000, 0.000000000000000000 ) ) ;
#14110=ORIENTED_EDGE ( 'NONE', *, *, #2715, .F. ) ;
#14112=FACE_OUTER_BOUND ( 'NONE', #30120, .T. ) ;
#14116=DIRECTION ( 'NONE',  ( -1.000000000000000000, 0.000000000000000000, 0.000000000000000000 ) ) ;
#14119=CIRCLE ( 'NONE', #38131, 0.5000000000000000000 ) ;
#14120=FACE_OUTER_BOUND ( 'NONE', #2738, .T. ) ;
#14125=DIRECTION ( 'NONE',  ( 1.000000000000000000, 0.000000000000000000, 0.000000000000000000 ) ) ;
#14127=ORIENTED_EDGE ( 'NONE', *, *, #7401, .T. ) ;
#14131=DIRECTION ( 'NONE',  ( -0.000000000000000000, -0.000000000000000000, 1.000000000000000000 ) ) ;
#14139=ORIENTED_EDGE ( 'NONE', *, *, #10855, .F. ) ;
#14141=DIRECTION ( 'NONE',  ( 0.000000000000000000, -0.7071067811865451302, -0.7071067811865500152 ) ) ;
#14143=CARTESIAN_POINT ( 'NONE',  ( -4.591666147298613332, 15.32946292166675306, 9.000000000000001776 ) ) ;
#14145=ORIENTED_EDGE ( 'NONE', *, *, #37029, .T. ) ;
#14147=VECTOR ( 'NONE', #17310, 1000.000000000000114 ) ;
#14148=VECTOR ( 'NONE', #23243, 1000.000000000000000 ) ;
#14151=DIRECTION ( 'NONE',  ( 0.4156269377774486906, -0.5720614028176846944, -0.7071067811865499042 ) ) ;
#14155=CARTESIAN_POINT ( 'NONE',  ( 3.503793317224329851, 8.420815634768676006, 7.000000000000000000 ) ) ;
#14156=VECTOR ( 'NONE', #6881, 1000.000000000000000 ) ;
#14159=DIRECTION ( 'NONE',  ( 1.000000000000000000, 0.000000000000000000, 0.000000000000000000 ) ) ;
#14163=CARTESIAN_POINT ( 'NONE',  ( 13.76030399595649811, 27.49672490655773416, 11.00000000000000178 ) ) ;
#14164=DIRECTION ( 'NONE',  ( 0.000000000000000000, 0.000000000000000000, 1.000000000000000000 ) ) ;
#14166=CARTESIAN_POINT ( 'NONE',  ( 12.30736835487432757, 14.81698729810772441, 7.000000000000000000 ) ) ;
#14167=VECTOR ( 'NONE', #8254, 1000.000000000000000 ) ;
#14171=ORIENTED_EDGE ( 'NONE', *, *, #18794, .T. ) ;
#14173=CARTESIAN_POINT ( 'NONE',  ( -6.557822374958138134, 35.99981354310120452, 11.00000000000000000 ) ) ;
#14178=AXIS2_PLACEMENT_3D ( 'NONE', #38285, #20210, #29345 ) ;
#14180=DIRECTION ( 'NONE',  ( -0.5000000000000039968, -0.8660254037844363761, 0.000000000000000000 ) ) ;
#14181=CONICAL_SURFACE ( 'NONE', #15400, 1.000000000000000888, 0.7853981633974552734 ) ;
#14187=EDGE_CURVE ( 'NONE', #802, #10420, #20712, .T. ) ;
#14188=ORIENTED_EDGE ( 'NONE', *, *, #12097, .T. ) ;
#14191=CARTESIAN_POINT ( 'NONE',  ( 0.000000000000000000, 22.50000000000000355, 7.000000000000000000 ) ) ;
#14194=CARTESIAN_POINT ( 'NONE',  ( 9.331903152615751651, 11.35703883385569135, 10.49999999999999822 ) ) ;
#14195=VERTEX_POINT ( 'NONE', #5131 ) ;
#14200=AXIS2_PLACEMENT_3D ( 'NONE', #8145, #2259, #23391 ) ;
#14201=VECTOR ( 'NONE', #2911, 1000.000000000000227 ) ;
#14204=CARTESIAN_POINT ( 'NONE',  ( 14.07088901726639918, 27.73527618063598510, 10.49999999999999822 ) ) ;
#14205=ORIENTED_EDGE ( 'NONE', *, *, #17328, .T. ) ;
#14206=VECTOR ( 'NONE', #20162, 1000.000000000000114 ) ;
#14207=DIRECTION ( 'NONE',  ( -0.4067366430757984874, -0.9135454576426016438, 0.000000000000000000 ) ) ;
#14212=DIRECTION ( 'NONE',  ( 1.000000000000000000, 0.000000000000000000, 0.000000000000000000 ) ) ;
#14214=EDGE_CURVE ( 'NONE', #36487, #7885, #34656, .T. ) ;
#14215=DIRECTION ( 'NONE',  ( 0.1470157664652005924, 0.6916548014802259559, -0.7071067811865465735 ) ) ;
#14218=ORIENTED_EDGE ( 'NONE', *, *, #16970, .F. ) ;
#14219=DIRECTION ( 'NONE',  ( -0.4067366430757888285, 0.9135454576426059736, -0.000000000000000000 ) ) ;
#14222=PLANE ( 'NONE',  #10249 ) ;
#14228=EDGE_CURVE ( 'NONE', #11410, #17070, #30454, .T. ) ;
#14229=FACE_OUTER_BOUND ( 'NONE', #30895, .T. ) ;
#14231=ORIENTED_EDGE ( 'NONE', *, *, #37797, .T. ) ;
#14234=DIRECTION ( 'NONE',  ( 0.000000000000000000, 0.000000000000000000, -1.000000000000000000 ) ) ;
#14235=EDGE_CURVE ( 'NONE', #27237, #34166, #16078, .T. ) ;
#14239=ORIENTED_EDGE ( 'NONE', *, *, #32466, .T. ) ;
#14241=EDGE_CURVE ( 'NONE', #16505, #36670, #36016, .T. ) ;
#14242=CARTESIAN_POINT ( 'NONE',  ( -10.47540670418176312, 32.60491492691384252, 11.00000000000000000 ) ) ;
#14243=DIRECTION ( 'NONE',  ( 0.1045284632676436176, -0.9945218953682742891, 0.000000000000000000 ) ) ;
#14244=FACE_OUTER_BOUND ( 'NONE', #19066, .T. ) ;
#14257=VECTOR ( 'NONE', #4364, 1000.000000000000000 ) ;
#14258=DIRECTION ( 'NONE',  ( 0.000000000000000000, 0.000000000000000000, -1.000000000000000000 ) ) ;
#14263=EDGE_CURVE ( 'NONE', #3290, #21446, #3770, .T. ) ;
#14270=DIRECTION ( 'NONE',  ( 1.000000000000000000, 0.000000000000000000, 0.000000000000000000 ) ) ;
#14274=EDGE_LOOP ( 'NONE', ( #26322, #20497, #36017, #28334, #3681 ) ) ;
#14277=CARTESIAN_POINT ( 'NONE',  ( -14.44923221060097696, 26.57085556310783758, 10.49999999999999822 ) ) ;
#14283=DIRECTION ( 'NONE',  ( -0.5000000000000039968, -0.8660254037844363761, 0.000000000000000000 ) ) ;
#14285=EDGE_CURVE ( 'NONE', #35381, #21371, #25153, .T. ) ;
#14286=LINE ( 'NONE', #35628, #16557 ) ;
#14294=CARTESIAN_POINT ( 'NONE',  ( -8.336672018935676221, 10.01592710129222752, 10.49999999999999822 ) ) ;
#14297=ORIENTED_EDGE ( 'NONE', *, *, #25241, .T. ) ;
#14298=ADVANCED_FACE ( 'NONE', ( #16370 ), #34003, .T. ) ;
#14302=ORIENTED_EDGE ( 'NONE', *, *, #2420, .F. ) ;
#14306=CIRCLE ( 'NONE', #29873, 0.5000000000000004441 ) ;
#14310=CARTESIAN_POINT ( 'NONE',  ( -1.734965421685230824, 7.600674680189156263, 7.000000000000000000 ) ) ;
#14313=VERTEX_POINT ( 'NONE', #36217 ) ;
#14315=CARTESIAN_POINT ( 'NONE',  ( 10.39021566973303656, 20.90519018800546291, 10.50000000000000000 ) ) ;
#14318=AXIS2_PLACEMENT_3D ( 'NONE', #28850, #22546, #10976 ) ;
#14319=CARTESIAN_POINT ( 'NONE',  ( -0.5000000000000005551, 33.00000000000000000, 10.00000000000000000 ) ) ;
#14320=DIRECTION ( 'NONE',  ( -0.1045284632676436176, 0.9945218953682742891, 0.000000000000000000 ) ) ;
#14330=CARTESIAN_POINT ( 'NONE',  ( 8.927394655428276593, 11.06314620770945290, 7.000000000000000000 ) ) ;
#14335=EDGE_CURVE ( 'NONE', #21780, #3918, #20780, .T. ) ;
#14341=VERTEX_POINT ( 'NONE', #36610 ) ;
#14342=ADVANCED_FACE ( 'NONE', ( #12023 ), #21564, .T. ) ;
#14344=VECTOR ( 'NONE', #3174, 1000.000000000000000 ) ;
#14347=DIRECTION ( 'NONE',  ( 0.000000000000000000, 0.000000000000000000, 1.000000000000000000 ) ) ;
#14348=EDGE_LOOP ( 'NONE', ( #6128, #9827, #34049, #15044 ) ) ;
#14351=EDGE_CURVE ( 'NONE', #9357, #26640, #21170, .T. ) ;
#14354=FACE_OUTER_BOUND ( 'NONE', #24018, .T. ) ;
#14356=DIRECTION ( 'NONE',  ( -0.8910065241883693421, -0.4539904997395438069, 0.000000000000000000 ) ) ;
#14357=DIRECTION ( 'NONE',  ( -0.000000000000000000, -0.000000000000000000, 1.000000000000000000 ) ) ;
#14358=EDGE_LOOP ( 'NONE', ( #36481, #25574, #10506 ) ) ;
#14361=EDGE_CURVE ( 'NONE', #34828, #4212, #11633, .T. ) ;
#14364=CARTESIAN_POINT ( 'NONE',  ( 15.02235689379175732, 21.92659494635341844, 7.000000000000000000 ) ) ;
#14365=ORIENTED_EDGE ( 'NONE', *, *, #30256, .T. ) ;
#14374=CARTESIAN_POINT ( 'NONE',  ( -13.94482798346716201, 26.50521816028930644, 7.000000000000000000 ) ) ;
#14375=ORIENTED_EDGE ( 'NONE', *, *, #5915, .T. ) ;
#14377=CARTESIAN_POINT ( 'NONE',  ( -7.111215932167764819, 17.81698729810783988, 7.000000000000000000 ) ) ;
#14378=DIRECTION ( 'NONE',  ( 0.000000000000000000, 0.000000000000000000, -1.000000000000000000 ) ) ;
#14381=CARTESIAN_POINT ( 'NONE',  ( 8.927394655428276593, 11.06314620770945290, 9.000000000000001776 ) ) ;
#14384=CARTESIAN_POINT ( 'NONE',  ( 14.36830325120613239, 20.48707633493483371, 7.000000000000000000 ) ) ;
#14389=EDGE_CURVE ( 'NONE', #35442, #38427, #33378, .T. ) ;
#14391=CARTESIAN_POINT ( 'NONE',  ( -2.525645716490712012, 8.212903943950955465, 7.499999999999997335 ) ) ;
#14392=VERTEX_POINT ( 'NONE', #30318 ) ;
#14397=CARTESIAN_POINT ( 'NONE',  ( -14.51390269127088928, 5.102206419419879957, 7.499999999999991118 ) ) ;
#14398=ORIENTED_EDGE ( 'NONE', *, *, #36219, .T. ) ;
#14401=ORIENTED_EDGE ( 'NONE', *, *, #28856, .F. ) ;
#14410=CARTESIAN_POINT ( 'NONE',  ( 3.992867117591230919, 8.524771480177550487, 7.000000000000000000 ) ) ;
#14411=FACE_OUTER_BOUND ( 'NONE', #10657, .T. ) ;
#14412=CARTESIAN_POINT ( 'NONE',  ( -4.003793317224517700, 8.420815634768723967, 7.499999999999997335 ) ) ;
#14415=DIRECTION ( 'NONE',  ( -0.1470157664652036733, -0.6916548014802235134, -0.7071067811865484609 ) ) ;
#14418=EDGE_LOOP ( 'NONE', ( #7209, #24186, #22360 ) ) ;
#14419=CARTESIAN_POINT ( 'NONE',  ( -7.419976537719776388, 10.58597682645832450, 9.500000000000000000 ) ) ;
#14421=CARTESIAN_POINT ( 'NONE',  ( -14.09933648065464062, 26.02968990214173317, 7.499999999999993783 ) ) ;
#14423=DIRECTION ( 'NONE',  ( 0.000000000000000000, 0.000000000000000000, 1.000000000000000000 ) ) ;
#14424=CARTESIAN_POINT ( 'NONE',  ( -10.39021566973305788, 20.90519018800561568, 10.00000000000000000 ) ) ;
#14428=LINE ( 'NONE', #4689, #36104 ) ;
#14430=VERTEX_POINT ( 'NONE', #2488 ) ;
#14432=DIRECTION ( 'NONE',  ( -0.000000000000000000, -0.000000000000000000, -1.000000000000000000 ) ) ;
#14436=ORIENTED_EDGE ( 'NONE', *, *, #31491, .T. ) ;
#14438=CARTESIAN_POINT ( 'NONE',  ( 11.48173768534036121, 32.16538668264416145, 10.63089969389957190 ) ) ;
#14439=DIRECTION ( 'NONE',  ( -0.5877852522924690293, 0.8090169943749503378, 0.000000000000000000 ) ) ;
#14441=B_SPLINE_CURVE_WITH_KNOTS ( 'NONE', 3,
 ( #25346, #37942, #37746, #21899, #37349, #9917 ),
 .UNSPECIFIED., .F., .F.,
 ( 4, 2, 4 ),
 ( 0.000000000000000000, 0.5000000000000000000, 1.000000000000000000 ),
 .UNSPECIFIED. ) ;
#14444=CARTESIAN_POINT ( 'NONE',  ( -13.48130249190472796, 27.93180293473203690, 10.50000000000000533 ) ) ;
#14445=ORIENTED_EDGE ( 'NONE', *, *, #14900, .T. ) ;
#14448=EDGE_LOOP ( 'NONE', ( #16077, #24385, #38228 ) ) ;
#14451=DIRECTION ( 'NONE',  ( -0.000000000000000000, -0.000000000000000000, -1.000000000000000000 ) ) ;
#14453=AXIS2_PLACEMENT_3D ( 'NONE', #21409, #5964, #19714 ) ;
#14454=CARTESIAN_POINT ( 'NONE',  ( 8.238488885696289898, 24.65111619403943877, 7.000000000000000000 ) ) ;
#14456=EDGE_CURVE ( 'NONE', #9704, #7162, #19853, .T. ) ;
#14457=CARTESIAN_POINT ( 'NONE',  ( -8.927394655428429360, 11.06314620770957013, 7.500000000000000888 ) ) ;
#14458=AXIS2_PLACEMENT_3D ( 'NONE', #34154, #23, #9963 ) ;
#14460=B_SPLINE_CURVE_WITH_KNOTS ( 'NONE', 3,
 ( #7063, #31659, #17033, #19259 ),
 .UNSPECIFIED., .F., .F.,
 ( 4, 4 ),
 ( 0.000000000000000000, 1.000000000000000000 ),
 .UNSPECIFIED. ) ;
#14462=CIRCLE ( 'NONE', #2781, 15.00000000000000000 ) ;
#14463=DIRECTION ( 'NONE',  ( 0.000000000000000000, 0.000000000000000000, 1.000000000000000000 ) ) ;
#14468=DIRECTION ( 'NONE',  ( 0.000000000000000000, 0.000000000000000000, -1.000000000000000000 ) ) ;
#14469=CARTESIAN_POINT ( 'NONE',  ( -13.30684946193824914, 15.76689913224038264, 10.49999999999999822 ) ) ;
#14470=DIRECTION ( 'NONE',  ( -1.000000000000000000, -0.000000000000000000, -0.000000000000000000 ) ) ;
#14471=ORIENTED_EDGE ( 'NONE', *, *, #14721, .F. ) ;
#14481=ORIENTED_EDGE ( 'NONE', *, *, #19138, .T. ) ;
#14485=CARTESIAN_POINT ( 'NONE',  ( -13.80736835487442349, 15.68301270189233954, 7.000000000000000000 ) ) ;
#14487=ORIENTED_EDGE ( 'NONE', *, *, #20329, .F. ) ;
#14490=CARTESIAN_POINT ( 'NONE',  ( -3.399837471815634338, 8.909889435135630364, 10.00000000000000000 ) ) ;
#14491=ORIENTED_EDGE ( 'NONE', *, *, #18373, .T. ) ;
#14494=ADVANCED_FACE ( 'NONE', ( #18323 ), #30719, .F. ) ;
#14496=EDGE_CURVE ( 'NONE', #38107, #7643, #30999, .T. ) ;
#14502=ORIENTED_EDGE ( 'NONE', *, *, #29167, .F. ) ;
#14504=DIRECTION ( 'NONE',  ( 0.000000000000000000, 0.000000000000000000, 1.000000000000000000 ) ) ;
#14506=CARTESIAN_POINT ( 'NONE',  ( -12.49038105676665644, 14.13397459621567798, 7.000000000000000000 ) ) ;
#14509=EDGE_CURVE ( 'NONE', #39108, #10259, #6729, .T. ) ;
#14511=CARTESIAN_POINT ( 'NONE',  ( 3.000488737323008248, 30.46850471149999962, 9.000000000000001776 ) ) ;
#14512=DIRECTION ( 'NONE',  ( 0.7431448254773953543, 0.6691306063588570163, 0.000000000000000000 ) ) ;
#14516=DIRECTION ( 'NONE',  ( 0.6724985119639642628, -0.2185080122244146550, -0.7071067811865395791 ) ) ;
#14517=PLANE ( 'NONE',  #17495 ) ;
#14520=CARTESIAN_POINT ( 'NONE',  ( -14.81881748179393199, 20.25565617689067111, 10.49999999999999822 ) ) ;
#14524=APPLICATION_CONTEXT ( 'automotive_design' ) ;
#14528=CARTESIAN_POINT ( 'NONE',  ( -11.22168704032801401, 31.70696390855199454, 10.83333333333332860 ) ) ;
#14531=DIRECTION ( 'NONE',  ( 0.000000000000000000, 0.000000000000000000, -1.000000000000000000 ) ) ;
#14532=ORIENTED_EDGE ( 'NONE', *, *, #7482, .F. ) ;
#14538=AXIS2_PLACEMENT_3D ( 'NONE', #9527, #27257, #6461 ) ;
#14540=CARTESIAN_POINT ( 'NONE',  ( -9.697889840765284930, 31.90483559858339646, 9.500000000000000000 ) ) ;
#14542=ORIENTED_EDGE ( 'NONE', *, *, #22530, .F. ) ;
#14544=DIRECTION ( 'NONE',  ( 0.000000000000000000, 0.000000000000000000, 1.000000000000000000 ) ) ;
#14545=DIRECTION ( 'NONE',  ( -0.9945218953682745111, -0.1045284632676436454, 0.000000000000000000 ) ) ;
#14547=FACE_OUTER_BOUND ( 'NONE', #27323, .T. ) ;
#14550=VECTOR ( 'NONE', #21756, 1000.000000000000000 ) ;
#14555=FACE_OUTER_BOUND ( 'NONE', #21768, .T. ) ;
#14556=B_SPLINE_CURVE_WITH_KNOTS ( 'NONE', 3,
 ( #36740, #3399, #2805, #6634, #21882, #24343, #28183, #33702 ),
 .UNSPECIFIED., .F., .F.,
 ( 4, 2, 2, 4 ),
 ( 0.000000000000000000, 0.0002364868538934255301, 0.0004729737077868510602, 0.0009459474155737019035 ),
 .UNSPECIFIED. ) ;
#14561=CARTESIAN_POINT ( 'NONE',  ( 8.411683849014126579, 19.76687823897103868, 7.000000000000000000 ) ) ;
#14562=EDGE_CURVE ( 'NONE', #21540, #23066, #9778, .T. ) ;
#14563=DIRECTION ( 'NONE',  ( -0.000000000000000000, 0.000000000000000000, 1.000000000000000000 ) ) ;
#14564=ORIENTED_EDGE ( 'NONE', *, *, #31537, .F. ) ;
#14565=AXIS2_PLACEMENT_3D ( 'NONE', #6411, #12122, #25105 ) ;
#14566=ADVANCED_FACE ( 'NONE', ( #28057 ), #3277, .F. ) ;
#14568=LINE ( 'NONE', #11919, #23076 ) ;
#14569=CARTESIAN_POINT ( 'NONE',  ( -13.14827996435949053, 25.72067290776677950, 9.500000000000000000 ) ) ;
#14571=DIRECTION ( 'NONE',  ( 0.000000000000000000, 0.000000000000000000, 1.000000000000000000 ) ) ;
#14574=CARTESIAN_POINT ( 'NONE',  ( 10.44103466624280685, 32.57396620494213124, 7.499999999999997335 ) ) ;
#14575=CIRCLE ( 'NONE', #37281, 0.5000000000000004441 ) ;
#14578=ORIENTED_EDGE ( 'NONE', *, *, #17226, .F. ) ;
#14579=EDGE_CURVE ( 'NONE', #9314, #34341, #40084, .T. ) ;
#14582=CARTESIAN_POINT ( 'NONE',  ( -0.4999999999999998890, 37.23829181892400442, 10.94387467463335462 ) ) ;
#14584=CARTESIAN_POINT ( 'NONE',  ( -13.88403039571018560, 27.53692605078189715, 10.94611345180490503 ) ) ;
#14587=PLANE ( 'NONE',  #7523 ) ;
#14589=CONICAL_SURFACE ( 'NONE', #25590, 0.4999999999999897304, 0.7853981633974529419 ) ;
#14594=CARTESIAN_POINT ( 'NONE',  ( -0.5000000000000005551, 33.00000000000000000, 10.50000000000000000 ) ) ;
#14597=EDGE_CURVE ( 'NONE', #8691, #14016, #28658, .T. ) ;
#14598=EDGE_LOOP ( 'NONE', ( #15819, #38224, #108, #4475 ) ) ;
#14601=ORIENTED_EDGE ( 'NONE', *, *, #14856, .F. ) ;
#14604=EDGE_LOOP ( 'NONE', ( #15776, #11, #34693, #1811 ) ) ;
#14606=EDGE_LOOP ( 'NONE', ( #36834, #31732, #13069, #26986, #25372 ) ) ;
#14608=VECTOR ( 'NONE', #28610, 1000.000000000000000 ) ;
#14609=ORIENTED_EDGE ( 'NONE', *, *, #29796, .F. ) ;
#14610=LINE ( 'NONE', #14002, #21913 ) ;
#14611=VERTEX_POINT ( 'NONE', #28456 ) ;
#14612=CARTESIAN_POINT ( 'NONE',  ( -10.49474413300071340, 21.89971208337387765, 11.00000000000000000 ) ) ;
#14613=DIRECTION ( 'NONE',  ( -0.000000000000000000, -0.000000000000000000, -1.000000000000000000 ) ) ;
#14614=EDGE_CURVE ( 'NONE', #32024, #14045, #13015, .T. ) ;
#14616=VECTOR ( 'NONE', #27720, 1000.000000000000000 ) ;
#14617=CARTESIAN_POINT ( 'NONE',  ( 9.625795778761983001, 10.95253033666821274, 10.49999999999999645 ) ) ;
#14618=ORIENTED_EDGE ( 'NONE', *, *, #1677, .F. ) ;
#14620=DIRECTION ( 'NONE',  ( -0.8090169943749426773, 0.5877852522924796874, 0.000000000000000000 ) ) ;
#14622=CARTESIAN_POINT ( 'NONE',  ( -10.29511041547401717, 24.79362192464190073, 10.50000000000000000 ) ) ;
#14626=EDGE_CURVE ( 'NONE', #7898, #13849, #31706, .T. ) ;
#14628=DIRECTION ( 'NONE',  ( 1.000000000000000000, 0.000000000000000000, 0.000000000000000000 ) ) ;
#14629=DIRECTION ( 'NONE',  ( 1.000000000000000000, 0.000000000000000000, 0.000000000000000000 ) ) ;
#14631=FACE_OUTER_BOUND ( 'NONE', #3722, .T. ) ;
#14632=CARTESIAN_POINT ( 'NONE',  ( -9.221287281574667816, 10.65863771052210041, 10.63089969389957190 ) ) ;
#14636=ORIENTED_EDGE ( 'NONE', *, *, #2120, .T. ) ;
#14637=ORIENTED_EDGE ( 'NONE', *, *, #19413, .F. ) ;
#14640=CARTESIAN_POINT ( 'NONE',  ( -10.39021566973305788, 20.90519018800560858, 10.50000000000000000 ) ) ;
#14641=CARTESIAN_POINT ( 'NONE',  ( -12.62480652560827110, 14.42233381811242410, 10.49999999999999822 ) ) ;
#14642=EDGE_CURVE ( 'NONE', #21611, #16076, #6983, .T. ) ;
#14643=VECTOR ( 'NONE', #23260, 1000.000000000000000 ) ;
#14645=FACE_OUTER_BOUND ( 'NONE', #847, .T. ) ;
#14649=CARTESIAN_POINT ( 'NONE',  ( 10.44103466624280685, 32.57396620494213124, 7.000000000000000000 ) ) ;
#14650=DIRECTION ( 'NONE',  ( -0.5877852522924796874, -0.8090169943749425663, 0.000000000000000000 ) ) ;
#14651=ORIENTED_EDGE ( 'NONE', *, *, #5090, .T. ) ;
#14653=DIRECTION ( 'NONE',  ( 1.000000000000000000, 0.000000000000000000, 0.000000000000000000 ) ) ;
#14654=EDGE_LOOP ( 'NONE', ( #28963, #24661, #19696, #17262 ) ) ;
#14662=DIRECTION ( 'NONE',  ( -0.9781476007338070211, -0.2079116908177534029, 0.000000000000000000 ) ) ;
#14663=ORIENTED_EDGE ( 'NONE', *, *, #20355, .F. ) ;
#14664=EDGE_CURVE ( 'NONE', #31065, #34172, #3477, .T. ) ;
#14666=DIRECTION ( 'NONE',  ( -0.000000000000000000, -0.000000000000000000, 1.000000000000000000 ) ) ;
#14668=CIRCLE ( 'NONE', #4922, 0.5000000000000004441 ) ;
#14670=VECTOR ( 'NONE', #20130, 1000.000000000000000 ) ;
#14673=VECTOR ( 'NONE', #8883, 1000.000000000000114 ) ;
#14676=CARTESIAN_POINT ( 'NONE',  ( 6.651296319737277862, 27.81603774131160023, 9.000000000000001776 ) ) ;
#14680=VERTEX_POINT ( 'NONE', #6709 ) ;
#14683=CARTESIAN_POINT ( 'NONE',  ( 3.790080598862314076, 7.986505539068669890, 7.485646746502365723 ) ) ;
#14687=ORIENTED_EDGE ( 'NONE', *, *, #36568, .T. ) ;
#14689=CARTESIAN_POINT ( 'NONE',  ( 12.37435565298211415, 15.93301270189216545, 9.500000000000000000 ) ) ;
#14691=CARTESIAN_POINT ( 'NONE',  ( 13.48130249190479191, 27.93180293473185927, 10.50000000000000533 ) ) ;
#14692=ORIENTED_EDGE ( 'NONE', *, *, #14235, .F. ) ;
#14696=ORIENTED_EDGE ( 'NONE', *, *, #17243, .T. ) ;
#14698=ADVANCED_FACE ( 'NONE', ( #13210 ), #8953, .T. ) ;
#14699=DIRECTION ( 'NONE',  ( 0.3090169943749572767, 0.9510565162951503115, -0.000000000000000000 ) ) ;
#14701=EDGE_CURVE ( 'NONE', #23066, #23024, #10378, .T. ) ;
#14702=ORIENTED_EDGE ( 'NONE', *, *, #13011, .F. ) ;
#14704=EDGE_LOOP ( 'NONE', ( #10303, #24453, #38788 ) ) ;
#14709=ORIENTED_EDGE ( 'NONE', *, *, #16486, .T. ) ;
#14711=ADVANCED_FACE ( 'NONE', ( #26212 ), #14222, .F. ) ;
#14712=CARTESIAN_POINT ( 'NONE',  ( -10.73859285986284640, 31.49625607628545154, 9.500000000000000000 ) ) ;
#14714=DIRECTION ( 'NONE',  ( 1.000000000000000000, 1.224646799147353947E-16, -0.000000000000000000 ) ) ;
#14715=DIRECTION ( 'NONE',  ( -0.3535533905932752852, -0.6123724356957909176, 0.7071067811865499042 ) ) ;
#14717=DIRECTION ( 'NONE',  ( -1.000000000000000000, 0.000000000000000000, 0.000000000000000000 ) ) ;
#14718=ORIENTED_EDGE ( 'NONE', *, *, #20306, .T. ) ;
#14721=EDGE_CURVE ( 'NONE', #2211, #6988, #11183, .T. ) ;
#14722=DIRECTION ( 'NONE',  ( -0.2926062055178280108, -0.7622652262560040137, 0.5773502691896330585 ) ) ;
#14725=CARTESIAN_POINT ( 'NONE',  ( -8.910254037844422825, 17.93301270189230223, 10.49999999999999822 ) ) ;
#14728=VERTEX_POINT ( 'NONE', #26615 ) ;
#14730=AXIS2_PLACEMENT_3D ( 'NONE', #38264, #19571, #10433 ) ;
#14734=VERTEX_POINT ( 'NONE', #4878 ) ;
#14735=CARTESIAN_POINT ( 'NONE',  ( -14.66026487122501543, 21.46189821169957312, 10.96580508970284384 ) ) ;
#14740=LINE ( 'NONE', #21623, #26945 ) ;
#14748=EDGE_CURVE ( 'NONE', #9203, #29069, #10781, .T. ) ;
#14750=CARTESIAN_POINT ( 'NONE',  ( 13.94482798346721175, 26.50521816028912525, 7.500000000000000888 ) ) ;
#14751=CARTESIAN_POINT ( 'NONE',  ( -2.317734025672944842, 9.191051544684764707, 9.500000000000000000 ) ) ;
#14752=EDGE_LOOP ( 'NONE', ( #37940, #12995, #31293, #19081 ) ) ;
#14755=CARTESIAN_POINT ( 'NONE',  ( -1.500000000000000888, 37.00000000000000711, 7.000000000000000000 ) ) ;
#14756=ADVANCED_FACE ( 'NONE', ( #17292 ), #29265, .T. ) ;
#14760=CARTESIAN_POINT ( 'NONE',  ( 8.410254037844358876, 17.06698729810774395, 10.49999999999999822 ) ) ;
#14761=AXIS2_PLACEMENT_3D ( 'NONE', #27680, #28077, #18939 ) ;
#14762=CONICAL_SURFACE ( 'NONE', #23832, 0.5000000000000039968, 0.7853981633974498333 ) ;
#14766=AXIS2_PLACEMENT_3D ( 'NONE', #2385, #36507, #24705 ) ;
#14768=ORIENTED_EDGE ( 'NONE', *, *, #3242, .T. ) ;
#14770=CARTESIAN_POINT ( 'NONE',  ( -13.48130249190472796, 27.93180293473203690, 10.50000000000000533 ) ) ;
#14771=EDGE_CURVE ( 'NONE', #30975, #20195, #7923, .T. ) ;
#14772=CARTESIAN_POINT ( 'NONE',  ( -12.80736835487441816, 15.68301270189233243, 11.00000000000000000 ) ) ;
#14773=EDGE_CURVE ( 'NONE', #14611, #37418, #38403, .T. ) ;
#14774=CARTESIAN_POINT ( 'NONE',  ( -16.72075857324140102, 7.444561356925720297, 11.00000000000000000 ) ) ;
#14775=CARTESIAN_POINT ( 'NONE',  ( 14.36830325120613594, 20.48707633493483371, 7.000000000000000000 ) ) ;
#14779=CARTESIAN_POINT ( 'NONE',  ( -7.142883826790117574, 35.69074677139154517, 7.203056206335835654 ) ) ;
#14782=DIRECTION ( 'NONE',  ( 0.8153776007405468818, 0.04273212933193557689, 0.5773502691896386096 ) ) ;
#14788=DIRECTION ( 'NONE',  ( -0.9781476007338069101, -0.2079116908177532641, 0.000000000000000000 ) ) ;
#14789=CARTESIAN_POINT ( 'NONE',  ( -2.256323172317922232, 14.28970123917155277, 9.000000000000001776 ) ) ;
#14790=VECTOR ( 'NONE', #33936, 1000.000000000000000 ) ;
#14797=CIRCLE ( 'NONE', #2473, 0.5000000000000001110 ) ;
#14800=AXIS2_PLACEMENT_3D ( 'NONE', #5802, #15342, #5600 ) ;
#14804=CARTESIAN_POINT ( 'NONE',  ( -8.118377661053486349, 10.47536095541708967, 11.00000000000000000 ) ) ;
#14807=EDGE_LOOP ( 'NONE', ( #38772, #16196, #37952 ) ) ;
#14808=FACE_OUTER_BOUND ( 'NONE', #30554, .T. ) ;
#14809=ORIENTED_EDGE ( 'NONE', *, *, #1682, .F. ) ;
#14810=CARTESIAN_POINT ( 'NONE',  ( -2.421689871081829537, 8.701977744317861863, 7.000000000000000000 ) ) ;
#14812=AXIS2_PLACEMENT_3D ( 'NONE', #6635, #34886, #31435 ) ;
#14814=CARTESIAN_POINT ( 'NONE',  ( 9.697889840765411051, 31.90483559858327212, 9.500000000000000000 ) ) ;
#14815=ORIENTED_EDGE ( 'NONE', *, *, #15702, .T. ) ;
#14818=LINE ( 'NONE', #27207, #35125 ) ;
#14820=CARTESIAN_POINT ( 'NONE',  ( 8.412270287199559604, 10.07085245822950981, 7.000000000000000000 ) ) ;
#14822=EDGE_CURVE ( 'NONE', #30937, #6233, #32110, .T. ) ;
#14824=AXIS2_PLACEMENT_3D ( 'NONE', #39622, #39022, #5299 ) ;
#14826=ORIENTED_EDGE ( 'NONE', *, *, #38694, .F. ) ;
#14828=DIRECTION ( 'NONE',  ( -0.000000000000000000, -0.000000000000000000, -1.000000000000000000 ) ) ;
#14829=CARTESIAN_POINT ( 'NONE',  ( -14.81908441805110854, 20.17630175058580022, 7.455686640544910482 ) ) ;
#14831=CARTESIAN_POINT ( 'NONE',  ( -10.44103466624267185, 32.57396620494226624, 7.500000000000004441 ) ) ;
#14832=CARTESIAN_POINT ( 'NONE',  ( 7.111215932167702647, 17.81698729810774751, 7.000000000000000000 ) ) ;
#14836=DIRECTION ( 'NONE',  ( -0.9135454576426059736, -0.4067366430757889395, 0.000000000000000000 ) ) ;
#14837=ORIENTED_EDGE ( 'NONE', *, *, #11269, .F. ) ;
#14838=ORIENTED_EDGE ( 'NONE', *, *, #3566, .T. ) ;
#14843=AXIS2_PLACEMENT_3D ( 'NONE', #28808, #19875, #10323 ) ;
#14844=DIRECTION ( 'NONE',  ( 0.9510565162951541973, 0.3090169943749456194, 6.938893903907225222E-15 ) ) ;
#14847=EDGE_CURVE ( 'NONE', #29442, #7930, #15949, .T. ) ;
#14848=CARTESIAN_POINT ( 'NONE',  ( -14.47283171447380390, 21.48159823030330884, 7.000000000000000000 ) ) ;
#14849=DIRECTION ( 'NONE',  ( 0.000000000000000000, 0.000000000000000000, -1.000000000000000000 ) ) ;
#14851=ORIENTED_EDGE ( 'NONE', *, *, #8912, .F. ) ;
#14853=CARTESIAN_POINT ( 'NONE',  ( 12.30736835487432579, 14.81698729810772619, 9.000000000000001776 ) ) ;
#14856=EDGE_CURVE ( 'NONE', #22181, #36614, #9199, .T. ) ;
#14858=VERTEX_POINT ( 'NONE', #19513 ) ;
#14863=CARTESIAN_POINT ( 'NONE',  ( 3.992867117591230919, 8.524771480177550487, 10.49999999999999289 ) ) ;
#14864=ORIENTED_EDGE ( 'NONE', *, *, #12704, .F. ) ;
#14866=DIRECTION ( 'NONE',  ( -0.9945218953682727347, 0.1045284632676597436, 0.000000000000000000 ) ) ;
#14867=EDGE_CURVE ( 'NONE', #18426, #34264, #26006, .T. ) ;
#14871=VECTOR ( 'NONE', #9073, 1000.000000000000000 ) ;
#14872=DIRECTION ( 'NONE',  ( -1.000000000000000000, 0.000000000000000000, 0.000000000000000000 ) ) ;
#14875=DIRECTION ( 'NONE',  ( 0.2079116908177663092, 0.9781476007338041345, 0.000000000000000000 ) ) ;
#14877=LINE ( 'NONE', #24413, #17071 ) ;
#14881=ORIENTED_EDGE ( 'NONE', *, *, #13491, .F. ) ;
#14884=CARTESIAN_POINT ( 'NONE',  ( -14.42035624161473883, 26.65972665747678150, 10.63089969389956835 ) ) ;
#14888=ORIENTED_EDGE ( 'NONE', *, *, #19803, .F. ) ;
#14890=CARTESIAN_POINT ( 'NONE',  ( 8.172817770806538817, 10.40043057260416504, 10.99387789255783510 ) ) ;
#14894=EDGE_LOOP ( 'NONE', ( #16204, #31901, #1862, #5655, #39619 ) ) ;
#14897=DIRECTION ( 'NONE',  ( 1.000000000000000000, 0.000000000000000000, 0.000000000000000000 ) ) ;
#14898=ORIENTED_EDGE ( 'NONE', *, *, #9288, .T. ) ;
#14900=EDGE_CURVE ( 'NONE', #22179, #18984, #4481, .T. ) ;
#14901=CARTESIAN_POINT ( 'NONE',  ( -8.258442077957658611, 10.28257882428884606, 10.94387467463491248 ) ) ;
#14902=DIRECTION ( 'NONE',  ( -0.000000000000000000, -0.000000000000000000, 1.000000000000000000 ) ) ;
#14905=EDGE_LOOP ( 'NONE', ( #22587, #14, #6879 ) ) ;
#14909=EDGE_LOOP ( 'NONE', ( #12793, #30282, #32727 ) ) ;
#14911=VECTOR ( 'NONE', #39985, 1000.000000000000000 ) ;
#14913=DIRECTION ( 'NONE',  ( -1.000000000000000000, 0.000000000000000000, 0.000000000000000000 ) ) ;
#14915=DIRECTION ( 'NONE',  ( -0.000000000000000000, -0.000000000000000000, -1.000000000000000000 ) ) ;
#14917=PLANE ( 'NONE',  #39924 ) ;
#14923=EDGE_CURVE ( 'NONE', #659, #34496, #29862, .T. ) ;
#14924=CARTESIAN_POINT ( 'NONE',  ( -12.05736835487443237, 14.38397459621567442, 7.499999999999993783 ) ) ;
#14928=ORIENTED_EDGE ( 'NONE', *, *, #13593, .T. ) ;
#14931=LINE ( 'NONE', #21419, #22389 ) ;
#14933=ORIENTED_EDGE ( 'NONE', *, *, #38872, .F. ) ;
#14934=DIRECTION ( 'NONE',  ( 0.5877852522924689183, -0.8090169943749505599, -0.000000000000000000 ) ) ;
#14935=VECTOR ( 'NONE', #24500, 999.9999999999998863 ) ;
#14936=ORIENTED_EDGE ( 'NONE', *, *, #1445, .T. ) ;
#14938=DIRECTION ( 'NONE',  ( 1.000000000000000000, 0.000000000000000000, 0.000000000000000000 ) ) ;
#14943=CARTESIAN_POINT ( 'NONE',  ( 5.034171952702014785, 35.03623199971300295, 7.000000000000000000 ) ) ;
#14945=ORIENTED_EDGE ( 'NONE', *, *, #4112, .F. ) ;
#14950=VERTEX_POINT ( 'NONE', #39805 ) ;
#14953=CIRCLE ( 'NONE', #11786, 0.9999999999999994449 ) ;
#14958=ORIENTED_EDGE ( 'NONE', *, *, #13959, .T. ) ;
#14960=CARTESIAN_POINT ( 'NONE',  ( -7.645071344821658954, 9.594463043616254794, 7.000000000000000000 ) ) ;
#14962=DIRECTION ( 'NONE',  ( -0.9135454576426059736, -0.4067366430757888285, 0.000000000000000000 ) ) ;
#14964=LINE ( 'NONE', #17635, #30830 ) ;
#14965=EDGE_CURVE ( 'NONE', #8131, #19420, #3612, .T. ) ;
#14966=CARTESIAN_POINT ( 'NONE',  ( 14.86556419889026159, 20.43481210330100950, 10.49999999999999822 ) ) ;
#14967=DIRECTION ( 'NONE',  ( 0.000000000000000000, -0.000000000000000000, -1.000000000000000000 ) ) ;
#14968=DIRECTION ( 'NONE',  ( -0.000000000000000000, -0.000000000000000000, -1.000000000000000000 ) ) ;
#14972=DIRECTION ( 'NONE',  ( 0.000000000000000000, 0.000000000000000000, 1.000000000000000000 ) ) ;
#14974=CIRCLE ( 'NONE', #23385, 6.000000000000003553 ) ;
#14976=CARTESIAN_POINT ( 'NONE',  ( -3.503793317224520365, 8.420815634768723967, 11.00000000000000000 ) ) ;
#14977=EDGE_CURVE ( 'NONE', #1404, #5091, #35694, .T. ) ;
#14979=AXIS2_PLACEMENT_3D ( 'NONE', #6215, #22051, #18620 ) ;
#14981=EDGE_CURVE ( 'NONE', #27240, #35073, #8337, .T. ) ;
#14993=ORIENTED_EDGE ( 'NONE', *, *, #1200, .T. ) ;
#14996=VERTEX_POINT ( 'NONE', #2445 ) ;
#14997=CARTESIAN_POINT ( 'NONE',  ( 2.568190708544436873, 12.82247983807080871, 10.50000000000000000 ) ) ;
#14999=DIRECTION ( 'NONE',  ( 0.2079116908177663092, 0.9781476007338041345, 0.000000000000000000 ) ) ;
#15000=EDGE_CURVE ( 'NONE', #7701, #12819, #33131, .T. ) ;
#15004=VECTOR ( 'NONE', #18903, 1000.000000000000000 ) ;
#15005=ORIENTED_EDGE ( 'NONE', *, *, #26901, .T. ) ;
#15006=CARTESIAN_POINT ( 'NONE',  ( 6.654030453887980201, 35.94335816374507431, 7.500000000000000888 ) ) ;
#15009=DIRECTION ( 'NONE',  ( -0.8660254037844432595, -0.4999999999999920619, 0.000000000000000000 ) ) ;
#15012=CARTESIAN_POINT ( 'NONE',  ( 7.935100905948330841, 11.57827057593817344, 7.000000000000000000 ) ) ;
#15013=CARTESIAN_POINT ( 'NONE',  ( -14.47283171447380390, 21.48159823030330884, 11.00000000000000000 ) ) ;
#15014=FACE_OUTER_BOUND ( 'NONE', #2276, .T. ) ;
#15015=EDGE_CURVE ( 'NONE', #15686, #32385, #2245, .T. ) ;
#15019=EDGE_LOOP ( 'NONE', ( #25085, #34662, #36468, #27252 ) ) ;
#15024=CYLINDRICAL_SURFACE ( 'NONE', #39879, 0.4999999999999999445 ) ;
#15030=AXIS2_PLACEMENT_3D ( 'NONE', #12355, #9910, #24553 ) ;
#15031=DIRECTION ( 'NONE',  ( 0.2079116908177533474, -0.9781476007338067991, 0.000000000000000000 ) ) ;
#15032=ORIENTED_EDGE ( 'NONE', *, *, #29796, .T. ) ;
#15033=ORIENTED_EDGE ( 'NONE', *, *, #38895, .T. ) ;
#15035=CARTESIAN_POINT ( 'NONE',  ( 0.9438746746263467768, 37.23829181893392359, 10.49999999999999822 ) ) ;
#15036=DIRECTION ( 'NONE',  ( -0.7431448254773962425, -0.6691306063588561281, -0.000000000000000000 ) ) ;
#15037=CARTESIAN_POINT ( 'NONE',  ( -9.221287281574667816, 10.65863771052210041, 10.49999999999999822 ) ) ;
#15040=DIRECTION ( 'NONE',  ( -0.000000000000000000, -0.000000000000000000, -1.000000000000000000 ) ) ;
#15041=CIRCLE ( 'NONE', #2720, 0.4999999999999995559 ) ;
#15043=EDGE_CURVE ( 'NONE', #257, #14093, #12058, .T. ) ;
#15044=ORIENTED_EDGE ( 'NONE', *, *, #30204, .T. ) ;
#15046=DIRECTION ( 'NONE',  ( 0.7431448254773954654, 0.6691306063588569053, -0.000000000000000000 ) ) ;
#15050=ORIENTED_EDGE ( 'NONE', *, *, #29626, .T. ) ;
#15054=B_SPLINE_CURVE_WITH_KNOTS ( 'NONE', 3,
 ( #12741, #32034, #19044, #7444 ),
 .UNSPECIFIED., .F., .F.,
 ( 4, 4 ),
 ( 0.000000000000000000, 1.000000000000000000 ),
 .UNSPECIFIED. ) ;
#15057=DIRECTION ( 'NONE',  ( 0.6691306063588570163, -0.7431448254773952433, 0.000000000000000000 ) ) ;
#15058=EDGE_LOOP ( 'NONE', ( #8517, #28573, #18553, #19740 ) ) ;
#15060=DIRECTION ( 'NONE',  ( 0.000000000000000000, -0.000000000000000000, 1.000000000000000000 ) ) ;
#15063=DIRECTION ( 'NONE',  ( 0.000000000000000000, 0.000000000000000000, 1.000000000000000000 ) ) ;
#15064=ADVANCED_FACE ( 'NONE', ( #26977 ), #14587, .T. ) ;
#15066=VECTOR ( 'NONE', #15151, 1000.000000000000000 ) ;
#15068=LINE ( 'NONE', #5922, #15185 ) ;
#15071=ORIENTED_EDGE ( 'NONE', *, *, #5903, .T. ) ;
#15072=ORIENTED_EDGE ( 'NONE', *, *, #7809, .T. ) ;
#15074=EDGE_CURVE ( 'NONE', #9989, #481, #24534, .T. ) ;
#15075=VECTOR ( 'NONE', #30785, 1000.000000000000000 ) ;
#15078=CARTESIAN_POINT ( 'NONE',  ( 6.654030453887979313, 35.94335816374508141, 7.000000000000000000 ) ) ;
#15079=ORIENTED_EDGE ( 'NONE', *, *, #12500, .F. ) ;
#15080=EDGE_LOOP ( 'NONE', ( #25035, #13034, #27044, #28546, #26798 ) ) ;
#15082=DIRECTION ( 'NONE',  ( 1.000000000000000000, 0.000000000000000000, 0.000000000000000000 ) ) ;
#15088=VECTOR ( 'NONE', #30957, 1000.000000000000114 ) ;
#15089=CARTESIAN_POINT ( 'NONE',  ( 0.5000000000000000000, 37.26099332938166242, 10.94611345180491035 ) ) ;
#15090=ORIENTED_EDGE ( 'NONE', *, *, #6313, .F. ) ;
#15092=FACE_OUTER_BOUND ( 'NONE', #27874, .T. ) ;
#15095=EDGE_LOOP ( 'NONE', ( #13997, #16119, #35139, #9561 ) ) ;
#15096=ADVANCED_FACE ( 'NONE', ( #1795 ), #27627, .T. ) ;
#15098=ORIENTED_EDGE ( 'NONE', *, *, #39557, .T. ) ;
#15099=ADVANCED_FACE ( 'NONE', ( #30230 ), #21279, .T. ) ;
#15101=VECTOR ( 'NONE', #17179, 1000.000000000000000 ) ;
#15103=ORIENTED_EDGE ( 'NONE', *, *, #15043, .F. ) ;
#15104=CIRCLE ( 'NONE', #13143, 0.5000000000000004441 ) ;
#15106=LINE ( 'NONE', #33213, #17754 ) ;
#15107=CARTESIAN_POINT ( 'NONE',  ( 5.644276917315719899, 36.40655018617690786, 10.49999999999999822 ) ) ;
#15110=DIRECTION ( 'NONE',  ( 0.9945218953682745111, 0.1045284632676437703, -0.000000000000000000 ) ) ;
#15111=EDGE_CURVE ( 'NONE', #35073, #25278, #8286, .T. ) ;
#15114=DIRECTION ( 'NONE',  ( 0.000000000000000000, -0.000000000000000000, 1.000000000000000000 ) ) ;
#15115=ORIENTED_EDGE ( 'NONE', *, *, #21290, .F. ) ;
#15117=LINE ( 'NONE', #12662, #1496 ) ;
#15118=CARTESIAN_POINT ( 'NONE',  ( 8.410254037844358876, 17.06698729810774395, 10.00000000000000000 ) ) ;
#15127=CARTESIAN_POINT ( 'NONE',  ( 13.94482798346721353, 26.50521816028912525, 7.000000000000000000 ) ) ;
#15129=B_SPLINE_CURVE_WITH_KNOTS ( 'NONE', 3,
 ( #29789, #1969, #13940, #32647 ),
 .UNSPECIFIED., .F., .F.,
 ( 4, 4 ),
 ( 0.000000000000000000, 1.000000000000000000 ),
 .UNSPECIFIED. ) ;
#15132=ORIENTED_EDGE ( 'NONE', *, *, #2563, .T. ) ;
#15136=CARTESIAN_POINT ( 'NONE',  ( 7.713869163865849643, 10.18146832927074996, 10.49999999999999822 ) ) ;
#15137=AXIS2_PLACEMENT_3D ( 'NONE', #13508, #25897, #38296 ) ;
#15140=CARTESIAN_POINT ( 'NONE',  ( -12.03571151536224271, 31.45218678977246896, 7.000000000000000000 ) ) ;
#15142=ORIENTED_EDGE ( 'NONE', *, *, #31621, .F. ) ;
#15147=ORIENTED_EDGE ( 'NONE', *, *, #7350, .F. ) ;
#15149=VECTOR ( 'NONE', #13917, 1000.000000000000000 ) ;
#15151=DIRECTION ( 'NONE',  ( -0.4067366430758009299, -0.9135454576426005335, -0.000000000000000000 ) ) ;
#15154=DIRECTION ( 'NONE',  ( 0.000000000000000000, 0.000000000000000000, -1.000000000000000000 ) ) ;
#15155=CARTESIAN_POINT ( 'NONE',  ( -13.94482798346716201, 26.50521816028930644, 7.000000000000000000 ) ) ;
#15158=CARTESIAN_POINT ( 'NONE',  ( -13.63581098909220479, 27.45627467658446008, 9.500000000000000000 ) ) ;
#15159=B_SPLINE_CURVE_WITH_KNOTS ( 'NONE', 3,
 ( #2439, #11778, #30474, #28009, #30271, #14829, #17888, #24759 ),
 .UNSPECIFIED., .F., .F.,
 ( 4, 2, 2, 4 ),
 ( 0.000000000000000000, 0.0004726692273637240907, 0.0007090038410455856482, 0.0009453384547274473141 ),
 .UNSPECIFIED. ) ;
#15160=AXIS2_PLACEMENT_3D ( 'NONE', #24744, #37142, #22097 ) ;
#15161=DIRECTION ( 'NONE',  ( -0.2079116908177533474, 0.9781476007338067991, 0.000000000000000000 ) ) ;
#15162=DIRECTION ( 'NONE',  ( 0.8090169943749504489, 0.5877852522924690293, -0.000000000000000000 ) ) ;
#15164=DIRECTION ( 'NONE',  ( 0.8064441531181091305, 0.1277282058446026769, 0.5773502691896269523 ) ) ;
#15165=CARTESIAN_POINT ( 'NONE',  ( -13.19371393710743412, 15.45995597598988880, 10.76099332938164288 ) ) ;
#15169=CARTESIAN_POINT ( 'NONE',  ( 14.42035624161478857, 26.65972665747660031, 10.49999999999999822 ) ) ;
#15171=CARTESIAN_POINT ( 'NONE',  ( 10.72918489117954088, 32.98258515686300996, 7.000000000000000000 ) ) ;
#15172=ORIENTED_EDGE ( 'NONE', *, *, #1692, .F. ) ;
#15175=AXIS2_PLACEMENT_3D ( 'NONE', #8010, #17380, #9420 ) ;
#15179=DIRECTION ( 'NONE',  ( 1.000000000000000000, 0.000000000000000000, 0.000000000000000000 ) ) ;
#15181=ORIENTED_EDGE ( 'NONE', *, *, #14748, .F. ) ;
#15185=VECTOR ( 'NONE', #234, 1000.000000000000000 ) ;
#15191=CARTESIAN_POINT ( 'NONE',  ( 9.697889840765411051, 31.90483559858327212, 9.500000000000000000 ) ) ;
#15193=VERTEX_POINT ( 'NONE', #33492 ) ;
#15199=ADVANCED_FACE ( 'NONE', ( #8489 ), #5441, .T. ) ;
#15204=EDGE_CURVE ( 'NONE', #22179, #34387, #24125, .T. ) ;
#15205=EDGE_LOOP ( 'NONE', ( #20300, #8195, #21684, #26751 ) ) ;
#15208=ADVANCED_FACE ( 'NONE', ( #27178 ), #30882, .T. ) ;
#15209=DIRECTION ( 'NONE',  ( 0.7032331762534027586, -0.07391278520357077997, -0.7071067811865484609 ) ) ;
#15210=CYLINDRICAL_SURFACE ( 'NONE', #28569, 0.5000000000000004441 ) ;
#15213=CARTESIAN_POINT ( 'NONE',  ( -11.44473057578096764, 31.45924896672619298, 7.000000000000000000 ) ) ;
#15216=LINE ( 'NONE', #15012, #19130 ) ;
#15217=FACE_OUTER_BOUND ( 'NONE', #38282, .T. ) ;
#15218=FACE_OUTER_BOUND ( 'NONE', #30850, .T. ) ;
#15223=VERTEX_POINT ( 'NONE', #8890 ) ;
#15225=EDGE_CURVE ( 'NONE', #15233, #16758, #33690, .T. ) ;
#15227=CARTESIAN_POINT ( 'NONE',  ( 11.11016527260166775, 31.83082137946472656, 11.00000000000000000 ) ) ;
#15232=CARTESIAN_POINT ( 'NONE',  ( 2.140527761532493134, 7.619874298175136396, 11.00000000000000000 ) ) ;
#15233=VERTEX_POINT ( 'NONE', #34666 ) ;
#15236=CARTESIAN_POINT ( 'NONE',  ( 0.5934445985557578185, 37.50000000000000711, 10.49999999999999822 ) ) ;
#15237=DIRECTION ( 'NONE',  ( 0.000000000000000000, 0.000000000000000000, -1.000000000000000000 ) ) ;
#15238=CIRCLE ( 'NONE', #10068, 0.9999999999999986677 ) ;
#15239=CARTESIAN_POINT ( 'NONE',  ( 13.48130249190479191, 27.93180293473185927, 7.000000000000000000 ) ) ;
#15240=VERTEX_POINT ( 'NONE', #40160 ) ;
#15242=PLANE ( 'NONE',  #7656 ) ;
#15245=CIRCLE ( 'NONE', #37286, 0.5000000000000005551 ) ;
#15247=EDGE_CURVE ( 'NONE', #6531, #5452, #33485, .T. ) ;
#15248=DIRECTION ( 'NONE',  ( -0.6691306063588560171, 0.7431448254773962425, 0.000000000000000000 ) ) ;
#15249=ORIENTED_EDGE ( 'NONE', *, *, #8377, .F. ) ;
#15251=VECTOR ( 'NONE', #174, 1000.000000000000000 ) ;
#15254=ADVANCED_FACE ( 'NONE', ( #142 ), #28362, .F. ) ;
#15256=DIRECTION ( 'NONE',  ( 0.8090169943749505599, 0.5877852522924689183, 0.000000000000000000 ) ) ;
#15258=DIRECTION ( 'NONE',  ( 0.6691306063588671194, 0.7431448254773862505, 0.000000000000000000 ) ) ;
#15259=ORIENTED_EDGE ( 'NONE', *, *, #28970, .F. ) ;
#15260=CARTESIAN_POINT ( 'NONE',  ( 3.607749162633208329, 7.931741834401763391, 10.49999999999999822 ) ) ;
#15263=DIRECTION ( 'NONE',  ( -0.9135454576426006446, 0.4067366430758009299, 0.000000000000000000 ) ) ;
#15264=VECTOR ( 'NONE', #37562, 1000.000000000000114 ) ;
#15268=ADVANCED_FACE ( 'NONE', ( #25119 ), #32841, .T. ) ;
#15270=CIRCLE ( 'NONE', #8776, 1.000000000000002665 ) ;
#15271=DIRECTION ( 'NONE',  ( -0.000000000000000000, -0.000000000000000000, -1.000000000000000000 ) ) ;
#15272=CARTESIAN_POINT ( 'NONE',  ( 10.44103466624280507, 32.57396620494213124, 11.00000000000000000 ) ) ;
#15273=ORIENTED_EDGE ( 'NONE', *, *, #9017, .T. ) ;
#15279=CARTESIAN_POINT ( 'NONE',  ( -3.503793317224517700, 8.420815634768723967, 10.99999999999999289 ) ) ;
#15280=EDGE_LOOP ( 'NONE', ( #940, #30045, #28393, #36338 ) ) ;
#15281=ORIENTED_EDGE ( 'NONE', *, *, #2222, .F. ) ;
#15284=DIRECTION ( 'NONE',  ( 1.000000000000000000, 1.387778780781439522E-14, 0.000000000000000000 ) ) ;
#15285=ORIENTED_EDGE ( 'NONE', *, *, #18685, .F. ) ;
#15289=EDGE_LOOP ( 'NONE', ( #21393, #8512, #12047, #8577 ) ) ;
#15300=ORIENTED_EDGE ( 'NONE', *, *, #2466, .F. ) ;
#15303=CARTESIAN_POINT ( 'NONE',  ( -10.47589056713771249, 33.23591321793828257, 7.338691926023217071 ) ) ;
#15307=AXIS2_PLACEMENT_3D ( 'NONE', #31067, #21122, #33729 ) ;
#15308=CARTESIAN_POINT ( 'NONE',  ( 12.49038105676653743, 14.13397459621550745, 10.49999999999999822 ) ) ;
#15313=LINE ( 'NONE', #13412, #8630 ) ;
#15317=EDGE_CURVE ( 'NONE', #12819, #31457, #18560, .T. ) ;
#15319=ORIENTED_EDGE ( 'NONE', *, *, #1055, .T. ) ;
#15322=DIRECTION ( 'NONE',  ( 0.6724985119639617093, -0.2185080122244195122, -0.7071067811865406894 ) ) ;
#15326=EDGE_LOOP ( 'NONE', ( #38541, #32086, #6617, #39135 ) ) ;
#15332=CONICAL_SURFACE ( 'NONE', #36105, 1.000000000000002665, 0.7853981633974509435 ) ;
#15335=CARTESIAN_POINT ( 'NONE',  ( 8.927394655428276593, 11.06314620770945290, 7.000000000000000000 ) ) ;
#15337=EDGE_LOOP ( 'NONE', ( #4719, #25193, #39002 ) ) ;
#15339=VECTOR ( 'NONE', #3140, 1000.000000000000227 ) ;
#15340=DIRECTION ( 'NONE',  ( 1.000000000000000000, 0.000000000000000000, 0.000000000000000000 ) ) ;
#15342=DIRECTION ( 'NONE',  ( -0.8660254037844432595, -0.4999999999999920064, 0.000000000000000000 ) ) ;
#15347=CARTESIAN_POINT ( 'NONE',  ( -4.678013043399448456, 44.50832101651065642, 11.00000000000000000 ) ) ;
#15350=VERTEX_POINT ( 'NONE', #3584 ) ;
#15353=EDGE_CURVE ( 'NONE', #11532, #19973, #15981, .T. ) ;
#15355=DIRECTION ( 'NONE',  ( 1.000000000000000000, 0.000000000000000000, 0.000000000000000000 ) ) ;
#15357=AXIS2_PLACEMENT_3D ( 'NONE', #26876, #39466, #39265 ) ;
#15361=CARTESIAN_POINT ( 'NONE',  ( 2.317734025672766318, 9.191051544684729180, 9.500000000000000000 ) ) ;
#15365=DIRECTION ( 'NONE',  ( -1.000000000000000000, 0.000000000000000000, 0.000000000000000000 ) ) ;
#15367=LINE ( 'NONE', #27559, #22275 ) ;
#15368=ADVANCED_FACE ( 'NONE', ( #27770 ), #30633, .F. ) ;
#15370=DIRECTION ( 'NONE',  ( -0.000000000000000000, -0.000000000000000000, -1.000000000000000000 ) ) ;
#15371=ORIENTED_EDGE ( 'NONE', *, *, #22285, .T. ) ;
#15373=CARTESIAN_POINT ( 'NONE',  ( 9.625795778761983001, 10.95253033666821274, 11.00000000000000000 ) ) ;
#15378=B_SPLINE_CURVE_WITH_KNOTS ( 'NONE', 3,
 ( #20266, #23104, #1373, #20068, #25943, #17225, #29402, #38343 ),
 .UNSPECIFIED., .F., .F.,
 ( 4, 2, 2, 4 ),
 ( 0.000000000000000000, 0.0002364868538934304361, 0.0004729737077868608722, 0.0009459474155737300927 ),
 .UNSPECIFIED. ) ;
#15380=ORIENTED_EDGE ( 'NONE', *, *, #31044, .F. ) ;
#15381=CARTESIAN_POINT ( 'NONE',  ( 14.42035624161478857, 26.65972665747660031, 11.00000000000000000 ) ) ;
#15389=FACE_OUTER_BOUND ( 'NONE', #34482, .T. ) ;
#15393=EDGE_CURVE ( 'NONE', #27469, #38623, #22081, .T. ) ;
#15398=CARTESIAN_POINT ( 'NONE',  ( 21.61735397326475905, 13.43626163844561994, 10.00000000000000000 ) ) ;
#15400=AXIS2_PLACEMENT_3D ( 'NONE', #11753, #39378, #2019 ) ;
#15403=CIRCLE ( 'NONE', #3706, 0.9999999999999985567 ) ;
#15404=ORIENTED_EDGE ( 'NONE', *, *, #29900, .F. ) ;
#15405=CARTESIAN_POINT ( 'NONE',  ( -4.503793317224517700, 8.420815634768723967, 7.000000000000000000 ) ) ;
#15406=VERTEX_POINT ( 'NONE', #21673 ) ;
#15407=CARTESIAN_POINT ( 'NONE',  ( -10.72918489117943963, 32.98258515686311654, 7.000000000000000000 ) ) ;
#15409=CARTESIAN_POINT ( 'NONE',  ( -5.187504188494229673, 36.60991850771488743, 11.00000000000000000 ) ) ;
#15412=CARTESIAN_POINT ( 'NONE',  ( -5.547064146435500831, 36.18820672788730519, 10.94611345180491035 ) ) ;
#15413=FACE_OUTER_BOUND ( 'NONE', #27321, .T. ) ;
#15414=CARTESIAN_POINT ( 'NONE',  ( -7.983541495324330661, 10.37739674670167389, 10.83333333333333215 ) ) ;
#15419=VECTOR ( 'NONE', #39525, 1000.000000000000114 ) ;
#15420=EDGE_LOOP ( 'NONE', ( #14651, #4453, #35372 ) ) ;
#15424=FACE_OUTER_BOUND ( 'NONE', #24773, .T. ) ;
#15428=CARTESIAN_POINT ( 'NONE',  ( 10.39021566973302946, 20.90519018800545581, 11.00000000000000000 ) ) ;
#15429=AXIS2_PLACEMENT_3D ( 'NONE', #33254, #20453, #2163 ) ;
#15433=CARTESIAN_POINT ( 'NONE',  ( -14.36830325120616081, 20.48707633493503977, 11.00000000000000000 ) ) ;
#15434=VERTEX_POINT ( 'NONE', #28168 ) ;
#15436=CARTESIAN_POINT ( 'NONE',  ( 0.5000000000000000000, 37.47223625998415741, 10.68306085400100081 ) ) ;
#15437=CARTESIAN_POINT ( 'NONE',  ( -12.80736835487441816, 15.68301270189233243, 11.00000000000000000 ) ) ;
#15438=CARTESIAN_POINT ( 'NONE',  ( -13.53057405073934838, 22.08338764125509002, 9.500000000000000000 ) ) ;
#15441=DIRECTION ( 'NONE',  ( 1.000000000000000000, 0.000000000000000000, 0.000000000000000000 ) ) ;
#15442=DIRECTION ( 'NONE',  ( 0.9945218953682730678, -0.1045284632676569819, 0.000000000000000000 ) ) ;
#15444=ORIENTED_EDGE ( 'NONE', *, *, #18989, .T. ) ;
#15446=CARTESIAN_POINT ( 'NONE',  ( -9.427394655416351910, 11.16786596286767441, 10.49999999999999822 ) ) ;
#15455=CARTESIAN_POINT ( 'NONE',  ( 6.868154521567912951, 35.60001939699333917, 10.49999999999999467 ) ) ;
#15457=AXIS2_PLACEMENT_3D ( 'NONE', #31678, #1209, #4651 ) ;
#15458=LINE ( 'NONE', #21548, #16180 ) ;
#15459=ORIENTED_EDGE ( 'NONE', *, *, #18694, .T. ) ;
#15460=CARTESIAN_POINT ( 'NONE',  ( 3.998603647807975392, 8.333314792924149117, 10.49999999999999822 ) ) ;
#15462=DIRECTION ( 'NONE',  ( 1.000000000000000000, 0.000000000000000000, 0.000000000000000000 ) ) ;
#15463=DIRECTION ( 'NONE',  ( -0.000000000000000000, -0.000000000000000000, -1.000000000000000000 ) ) ;
#15465=CARTESIAN_POINT ( 'NONE',  ( -2.256323172317922232, 14.28970123917155277, 9.000000000000001776 ) ) ;
#15468=DIRECTION ( 'NONE',  ( 0.5000000000000041078, 0.8660254037844362651, 0.000000000000000000 ) ) ;
#15469=CARTESIAN_POINT ( 'NONE',  ( -5.982165713378355676, 28.55918256678905820, 9.000000000000001776 ) ) ;
#15470=CARTESIAN_POINT ( 'NONE',  ( -12.05736835487443237, 14.38397459621567442, 10.50000000000000000 ) ) ;
#15471=EDGE_CURVE ( 'NONE', #34387, #15406, #37910, .T. ) ;
#15475=VECTOR ( 'NONE', #23114, 1000.000000000000000 ) ;
#15478=EDGE_CURVE ( 'NONE', #36997, #11661, #37400, .T. ) ;
#15479=CARTESIAN_POINT ( 'NONE',  ( -3.542977516905746249, 8.236468469132606884, 10.96580508970282075 ) ) ;
#15481=B_SPLINE_CURVE_WITH_KNOTS ( 'NONE', 3,
 ( #28937, #1115, #35237, #32195 ),
 .UNSPECIFIED., .F., .F.,
 ( 4, 4 ),
 ( 0.000000000000000000, 1.000000000000000000 ),
 .UNSPECIFIED. ) ;
#15482=ORIENTED_EDGE ( 'NONE', *, *, #35193, .T. ) ;
#15483=ORIENTED_EDGE ( 'NONE', *, *, #2944, .T. ) ;
#15484=CIRCLE ( 'NONE', #7032, 6.000000000000015987 ) ;
#15488=AXIS2_PLACEMENT_3D ( 'NONE', #37927, #34885, #16807 ) ;
#15489=ORIENTED_EDGE ( 'NONE', *, *, #20360, .F. ) ;
#15496=LINE ( 'NONE', #2902, #23831 ) ;
#15497=ORIENTED_EDGE ( 'NONE', *, *, #27179, .T. ) ;
#15499=ORIENTED_EDGE ( 'NONE', *, *, #5073, .F. ) ;
#15507=EDGE_CURVE ( 'NONE', #11960, #39304, #25073, .T. ) ;
#15508=CARTESIAN_POINT ( 'NONE',  ( -4.984135866956331817, 36.15314577889358105, 11.00000000000000000 ) ) ;
#15514=VECTOR ( 'NONE', #6549, 999.9999999999998863 ) ;
#15520=CARTESIAN_POINT ( 'NONE',  ( -0.7609933293816388833, 37.44611345180490503, 10.49999999999999467 ) ) ;
#15523=ADVANCED_FACE ( 'NONE', ( #16380 ), #8205, .T. ) ;
#15525=EDGE_LOOP ( 'NONE', ( #22024, #19479, #23796, #29839 ) ) ;
#15531=CARTESIAN_POINT ( 'NONE',  ( 14.52509594610761923, 21.97885917798724975, 7.500000000000010658 ) ) ;
#15540=CARTESIAN_POINT ( 'NONE',  ( 4.003793317224326742, 8.420815634768674229, 11.00000000000000000 ) ) ;
#15545=CARTESIAN_POINT ( 'NONE',  ( 7.143250075007565592, 35.69054364144594871, 7.202682876670055023 ) ) ;
#15547=ORIENTED_EDGE ( 'NONE', *, *, #9315, .T. ) ;
#15550=CARTESIAN_POINT ( 'NONE',  ( -5.599788042746297378, 36.30662653786500016, 10.82238861112318418 ) ) ;
#15552=ORIENTED_EDGE ( 'NONE', *, *, #36674, .T. ) ;
#15553=EDGE_CURVE ( 'NONE', #27538, #36749, #28766, .T. ) ;
#15555=DIRECTION ( 'NONE',  ( -0.000000000000000000, -0.000000000000000000, -1.000000000000000000 ) ) ;
#15556=VERTEX_POINT ( 'NONE', #4384 ) ;
#15557=CARTESIAN_POINT ( 'NONE',  ( 6.282361020112160688, 14.70372268239673197, 10.00000000000000000 ) ) ;
#15558=CIRCLE ( 'NONE', #25934, 0.5000000000000001110 ) ;
#15560=DIRECTION ( 'NONE',  ( 0.5877852522924691403, -0.8090169943749503378, 6.938893903907234689E-15 ) ) ;
#15562=DIRECTION ( 'NONE',  ( 1.000000000000000000, 0.000000000000000000, 0.000000000000000000 ) ) ;
#15563=CARTESIAN_POINT ( 'NONE',  ( -14.36830325120615548, 20.48707633493503621, 7.000000000000000000 ) ) ;
#15566=FACE_OUTER_BOUND ( 'NONE', #36346, .T. ) ;
#15567=CARTESIAN_POINT ( 'NONE',  ( 4.475131784526629630, 8.183115020678576101, 7.000000000000000000 ) ) ;
#15568=ADVANCED_FACE ( 'NONE', ( #13320 ), #10350, .T. ) ;
#15571=VERTEX_POINT ( 'NONE', #13725 ) ;
#15574=CARTESIAN_POINT ( 'NONE',  ( 13.05736835487433467, 16.11602540378438775, 10.49999999999999822 ) ) ;
#15575=EDGE_CURVE ( 'NONE', #33995, #34769, #27905, .T. ) ;
#15585=EDGE_CURVE ( 'NONE', #445, #22181, #1143, .T. ) ;
#15590=CARTESIAN_POINT ( 'NONE',  ( 11.61633080063109702, 31.93537370176170853, 10.49999999999999822 ) ) ;
#15595=ORIENTED_EDGE ( 'NONE', *, *, #19413, .T. ) ;
#15596=FACE_OUTER_BOUND ( 'NONE', #22125, .T. ) ;
#15598=ADVANCED_FACE ( 'NONE', ( #24079 ), #15332, .T. ) ;
#15601=EDGE_CURVE ( 'NONE', #30975, #8691, #33042, .T. ) ;
#15603=EDGE_CURVE ( 'NONE', #20131, #17593, #27655, .T. ) ;
#15606=ORIENTED_EDGE ( 'NONE', *, *, #9109, .T. ) ;
#15610=VERTEX_POINT ( 'NONE', #17996 ) ;
#15612=AXIS2_PLACEMENT_3D ( 'NONE', #36708, #24309, #17432 ) ;
#15613=CARTESIAN_POINT ( 'NONE',  ( 8.221629120123230550, 5.055853521246038262, 10.00000000000000000 ) ) ;
#15614=PLANE ( 'NONE',  #10505 ) ;
#15615=CARTESIAN_POINT ( 'NONE',  ( 14.09933648065468503, 26.02968990214155198, 11.00000000000000000 ) ) ;
#15620=VERTEX_POINT ( 'NONE', #11693 ) ;
#15625=CARTESIAN_POINT ( 'NONE',  ( 9.343266739736584725, 17.68301270189219210, 10.00000000000000000 ) ) ;
#15626=CONICAL_SURFACE ( 'NONE', #20826, 0.9999999999999981126, 0.7853981633974562726 ) ;
#15629=CARTESIAN_POINT ( 'NONE',  ( -3.000488737322915878, 30.46850471150003159, 9.000000000000001776 ) ) ;
#15635=CARTESIAN_POINT ( 'NONE',  ( 5.599788042746504324, 36.30662653786479410, 10.82238861112336537 ) ) ;
#15636=ORIENTED_EDGE ( 'NONE', *, *, #215, .T. ) ;
#15639=CARTESIAN_POINT ( 'NONE',  ( -12.97403502154108779, 15.97168783648715618, 10.66666666666666252 ) ) ;
#15642=ORIENTED_EDGE ( 'NONE', *, *, #29902, .F. ) ;
#15644=VECTOR ( 'NONE', #16916, 1000.000000000000000 ) ;
#15645=CARTESIAN_POINT ( 'NONE',  ( 14.44277748876681855, 26.55045409923015853, 7.500000000000000888 ) ) ;
#15646=DIRECTION ( 'NONE',  ( -1.000000000000000000, 0.000000000000000000, 0.000000000000000000 ) ) ;
#15647=ORIENTED_EDGE ( 'NONE', *, *, #30723, .F. ) ;
#15650=ORIENTED_EDGE ( 'NONE', *, *, #28985, .F. ) ;
#15655=VECTOR ( 'NONE', #34307, 1000.000000000000000 ) ;
#15656=CARTESIAN_POINT ( 'NONE',  ( -8.137585970691985082, 29.15429895402941440, 10.50000000000000000 ) ) ;
#15657=CARTESIAN_POINT ( 'NONE',  ( 6.811226782241714517, 35.33967249274190436, 10.49999999999999822 ) ) ;
#15659=LINE ( 'NONE', #28045, #2565 ) ;
#15661=CARTESIAN_POINT ( 'NONE',  ( 3.781037291632489250, 7.996959361763587459, 10.49999999999999822 ) ) ;
#15663=CARTESIAN_POINT ( 'NONE',  ( 12.59251905104225600, 14.34933092922137021, 7.455539900862797609 ) ) ;
#15664=DIRECTION ( 'NONE',  ( 0.000000000000000000, 0.000000000000000000, 1.000000000000000000 ) ) ;
#15669=LINE ( 'NONE', #31112, #14550 ) ;
#15670=CARTESIAN_POINT ( 'NONE',  ( -12.31033848243476214, 14.30014505118406021, 10.49999999999999822 ) ) ;
#15671=ORIENTED_EDGE ( 'NONE', *, *, #20072, .F. ) ;
#15676=FACE_OUTER_BOUND ( 'NONE', #16286, .T. ) ;
#15678=VERTEX_POINT ( 'NONE', #11298 ) ;
#15682=EDGE_LOOP ( 'NONE', ( #14398, #4684, #22520 ) ) ;
#15685=DIRECTION ( 'NONE',  ( -1.000000000000000000, 0.000000000000000000, 0.000000000000000000 ) ) ;
#15686=VERTEX_POINT ( 'NONE', #26928 ) ;
#15689=DIRECTION ( 'NONE',  ( -0.7071067811865526798, 0.000000000000000000, -0.7071067811865422437 ) ) ;
#15690=VERTEX_POINT ( 'NONE', #38918 ) ;
#15692=ORIENTED_EDGE ( 'NONE', *, *, #18359, .T. ) ;
#15696=ADVANCED_FACE ( 'NONE', ( #8237 ), #30384, .F. ) ;
#15699=CARTESIAN_POINT ( 'NONE',  ( 0.4999999999999990563, 31.00000000000000355, 9.000000000000001776 ) ) ;
#15701=DIRECTION ( 'NONE',  ( -1.000000000000000000, 0.000000000000000000, 0.000000000000000000 ) ) ;
#15702=EDGE_CURVE ( 'NONE', #29636, #11564, #4961, .T. ) ;
#15703=AXIS2_PLACEMENT_3D ( 'NONE', #30601, #8860, #36491 ) ;
#15706=AXIS2_PLACEMENT_3D ( 'NONE', #28319, #2948, #9649 ) ;
#15710=DIRECTION ( 'NONE',  ( -0.000000000000000000, -0.000000000000000000, 1.000000000000000000 ) ) ;
#15713=CARTESIAN_POINT ( 'NONE',  ( -13.30736791469135483, 15.68301270237671474, 10.49999999999999822 ) ) ;
#15717=VECTOR ( 'NONE', #36216, 1000.000000000000000 ) ;
#15723=ORIENTED_EDGE ( 'NONE', *, *, #13207, .T. ) ;
#15725=ORIENTED_EDGE ( 'NONE', *, *, #18485, .F. ) ;
#15727=DIRECTION ( 'NONE',  ( 0.2079116908177533474, -0.9781476007338067991, 0.000000000000000000 ) ) ;
#15729=DIRECTION ( 'NONE',  ( 0.000000000000000000, 0.000000000000000000, 1.000000000000000000 ) ) ;
#15730=ORIENTED_EDGE ( 'NONE', *, *, #34446, .T. ) ;
#15733=DIRECTION ( 'NONE',  ( -0.000000000000000000, -0.000000000000000000, -1.000000000000000000 ) ) ;
#15738=CONICAL_SURFACE ( 'NONE', #2773, 0.4999999999999958922, 0.7853981633974446153 ) ;
#15739=CARTESIAN_POINT ( 'NONE',  ( 9.331903152615748098, 11.35703883385568602, 9.500000000000000000 ) ) ;
#15744=AXIS2_PLACEMENT_3D ( 'NONE', #2898, #6332, #252 ) ;
#15746=ORIENTED_EDGE ( 'NONE', *, *, #10777, .F. ) ;
#15747=B_SPLINE_CURVE_WITH_KNOTS ( 'NONE', 3,
 ( #13065, #29121, #25455, #7174, #31961, #25267, #31767, #4128 ),
 .UNSPECIFIED., .F., .F.,
 ( 4, 2, 2, 4 ),
 ( 0.000000000000000000, 0.0002364868538934306529, 0.0004729737077868613059, 0.0009459474155737255391 ),
 .UNSPECIFIED. ) ;
#15748=EDGE_CURVE ( 'NONE', #34986, #253, #34791, .T. ) ;
#15750=DIRECTION ( 'NONE',  ( -0.000000000000000000, -0.000000000000000000, -1.000000000000000000 ) ) ;
#15754=CYLINDRICAL_SURFACE ( 'NONE', #26, 6.000000000000005329 ) ;
#15755=CARTESIAN_POINT ( 'NONE',  ( 3.914034194965609892, 30.06176806842420035, 7.000000000000000000 ) ) ;
#15757=CARTESIAN_POINT ( 'NONE',  ( 14.47283171447379146, 21.48159823030312054, 11.00000000000000000 ) ) ;
#15761=DIRECTION ( 'NONE',  ( 0.000000000000000000, 0.000000000000000000, -1.000000000000000000 ) ) ;
#15763=LINE ( 'NONE', #28154, #17170 ) ;
#15765=CARTESIAN_POINT ( 'NONE',  ( 3.503793317224320969, 8.420815634768672453, 11.00000000000000000 ) ) ;
#15767=AXIS2_PLACEMENT_3D ( 'NONE', #29763, #13916, #5177 ) ;
#15769=DIRECTION ( 'NONE',  ( -0.8090169943749504489, -0.5877852522924691403, 0.000000000000000000 ) ) ;
#15770=LINE ( 'NONE', #12918, #32847 ) ;
#15776=ORIENTED_EDGE ( 'NONE', *, *, #5213, .T. ) ;
#15777=CARTESIAN_POINT ( 'NONE',  ( -8.744117900323420400, 12.16605582823075160, 9.500000000000000000 ) ) ;
#15786=CARTESIAN_POINT ( 'NONE',  ( -9.331903152615899089, 11.35703883385581037, 10.50000000000000533 ) ) ;
#15796=EDGE_CURVE ( 'NONE', #9989, #24087, #8445, .T. ) ;
#15799=AXIS2_PLACEMENT_3D ( 'NONE', #11961, #24351, #20719 ) ;
#15800=EDGE_LOOP ( 'NONE', ( #14993, #20705, #13467 ) ) ;
#15801=EDGE_CURVE ( 'NONE', #26077, #10259, #29572, .T. ) ;
#15802=CARTESIAN_POINT ( 'NONE',  ( 0.000000000000000000, 22.50000000000000355, 7.000000000000000000 ) ) ;
#15803=ORIENTED_EDGE ( 'NONE', *, *, #28481, .F. ) ;
#15805=DIRECTION ( 'NONE',  ( -0.000000000000000000, -0.000000000000000000, -1.000000000000000000 ) ) ;
#15806=DIRECTION ( 'NONE',  ( 0.6691306063588670083, 0.7431448254773862505, -0.000000000000000000 ) ) ;
#15807=EDGE_CURVE ( 'NONE', #27094, #12629, #26530, .T. ) ;
#15808=DIRECTION ( 'NONE',  ( 0.5000000000000039968, 0.8660254037844363761, 0.000000000000000000 ) ) ;
#15809=ORIENTED_EDGE ( 'NONE', *, *, #34498, .T. ) ;
#15810=AXIS2_PLACEMENT_3D ( 'NONE', #17578, #20418, #35653 ) ;
#15812=CARTESIAN_POINT ( 'NONE',  ( -9.427394655437487003, 10.98460639141788242, 10.49999999999999822 ) ) ;
#15813=DIRECTION ( 'NONE',  ( 0.8090169943749426773, -0.5877852522924796874, 0.000000000000000000 ) ) ;
#15814=CARTESIAN_POINT ( 'NONE',  ( 10.33795143809920702, 20.40792924032132660, 10.50000000000000000 ) ) ;
#15815=LINE ( 'NONE', #578, #12589 ) ;
#15817=AXIS2_PLACEMENT_3D ( 'NONE', #6854, #1178, #36114 ) ;
#15819=ORIENTED_EDGE ( 'NONE', *, *, #23533, .F. ) ;
#15823=FACE_OUTER_BOUND ( 'NONE', #37032, .T. ) ;
#15825=EDGE_CURVE ( 'NONE', #1914, #22876, #8843, .T. ) ;
#15827=PLANE ( 'NONE',  #25843 ) ;
#15828=ADVANCED_FACE ( 'NONE', ( #27716 ), #14024, .T. ) ;
#15829=AXIS2_PLACEMENT_3D ( 'NONE', #12900, #28539, #715 ) ;
#15834=CARTESIAN_POINT ( 'NONE',  ( 8.395951170269764674, 10.09331379572982357, 10.68306085400111982 ) ) ;
#15835=CARTESIAN_POINT ( 'NONE',  ( -10.14060191828655100, 25.26915018278946690, 11.00000000000000000 ) ) ;
#15836=ORIENTED_EDGE ( 'NONE', *, *, #27748, .T. ) ;
#15839=CARTESIAN_POINT ( 'NONE',  ( 11.11016527260166420, 31.83082137946473367, 7.499999999999997335 ) ) ;
#15841=DIRECTION ( 'NONE',  ( -0.000000000000000000, -0.000000000000000000, -1.000000000000000000 ) ) ;
#15844=CARTESIAN_POINT ( 'NONE',  ( -14.46080647158818522, 26.53523365061255745, 10.49999999999999822 ) ) ;
#15845=CARTESIAN_POINT ( 'NONE',  ( -9.151574469205524309, 1.945227203041487218, 11.00000000000000000 ) ) ;
#15846=B_SPLINE_SURFACE_WITH_KNOTS ( 'NONE', 1, 3, ( 
 ( #39156, #22908, #26161, #29816, #4429, #14582, #38556, #23115, #38353, #8076 ),
 ( #20278, #1385, #35514, #20485, #20079, #17443, #17034, #32879, #11337, #5234 ) ),
 .UNSPECIFIED., .F., .F., .F.,
 ( 2, 2 ),
 ( 4, 2, 2, 2, 4 ),
 ( 0.000000000000000000, 1.000000000000000000 ),
 ( 1.570796326794891673, 1.963495408493616923, 2.356194490192342172, 2.748893571891067644, 3.141592653589793116 ),
 .UNSPECIFIED. ) ;
#15847=ORIENTED_EDGE ( 'NONE', *, *, #3771, .F. ) ;
#15850=ADVANCED_FACE ( 'NONE', ( #33832 ), #6375, .F. ) ;
#15853=ADVANCED_FACE ( 'NONE', ( #30779 ), #34419, .F. ) ;
#15854=ORIENTED_EDGE ( 'NONE', *, *, #25457, .T. ) ;
#15859=VECTOR ( 'NONE', #25993, 1000.000000000000000 ) ;
#15860=EDGE_CURVE ( 'NONE', #6329, #20052, #294, .T. ) ;
#15865=CARTESIAN_POINT ( 'NONE',  ( 10.14060191828658120, 25.26915018278934255, 10.50000000000000000 ) ) ;
#15866=DIRECTION ( 'NONE',  ( -0.000000000000000000, -0.000000000000000000, -1.000000000000000000 ) ) ;
#15871=EDGE_CURVE ( 'NONE', #17841, #38914, #18590, .T. ) ;
#15872=CARTESIAN_POINT ( 'NONE',  ( -12.56321727241662423, 14.36790371874266370, 10.49999999999999467 ) ) ;
#15873=EDGE_CURVE ( 'NONE', #34838, #30940, #3137, .T. ) ;
#15874=VECTOR ( 'NONE', #5676, 1000.000000000000000 ) ;
#15875=ORIENTED_EDGE ( 'NONE', *, *, #7273, .F. ) ;
#15879=CARTESIAN_POINT ( 'NONE',  ( -10.70158575030357895, 30.79011836036732319, 10.50000000000000000 ) ) ;
#15881=ORIENTED_EDGE ( 'NONE', *, *, #6213, .T. ) ;
#15883=CIRCLE ( 'NONE', #19127, 0.5000000000000015543 ) ;
#15887=EDGE_LOOP ( 'NONE', ( #5713, #26185, #16354, #2547 ) ) ;
#15890=CARTESIAN_POINT ( 'NONE',  ( 5.982165713378432059, 28.55918256678898715, 9.000000000000001776 ) ) ;
#15891=ORIENTED_EDGE ( 'NONE', *, *, #1682, .T. ) ;
#15893=DIRECTION ( 'NONE',  ( 0.000000000000000000, 0.000000000000000000, -1.000000000000000000 ) ) ;
#15894=DIRECTION ( 'NONE',  ( -0.8660254037844364872, 0.5000000000000038858, 0.000000000000000000 ) ) ;
#15895=ORIENTED_EDGE ( 'NONE', *, *, #34124, .F. ) ;
#15901=ADVANCED_FACE ( 'NONE', ( #9041 ), #5980, .T. ) ;
#15902=VERTEX_POINT ( 'NONE', #40107 ) ;
#15905=CIRCLE ( 'NONE', #30815, 6.000000000000006217 ) ;
#15907=DIRECTION ( 'NONE',  ( -0.6724985119639582676, -0.2185080122244135170, -0.7071067811865457964 ) ) ;
#15908=DIRECTION ( 'NONE',  ( -0.000000000000000000, -0.000000000000000000, -1.000000000000000000 ) ) ;
#15911=TOROIDAL_SURFACE ( 'NONE', #29548, 1.000000000000000000, 0.5000000000000000000 ) ;
#15913=PLANE ( 'NONE',  #1037 ) ;
#15917=CARTESIAN_POINT ( 'NONE',  ( -13.05736835487441994, 16.11602540378456183, 10.49999999999999822 ) ) ;
#15919=EDGE_LOOP ( 'NONE', ( #9454, #24637, #6494, #11974 ) ) ;
#15923=LINE ( 'NONE', #16731, #13995 ) ;
#15925=ORIENTED_EDGE ( 'NONE', *, *, #17514, .T. ) ;
#15928=VERTEX_POINT ( 'NONE', #24278 ) ;
#15930=DIRECTION ( 'NONE',  ( 0.8090169943749505599, 0.5877852522924689183, 0.000000000000000000 ) ) ;
#15936=DIRECTION ( 'NONE',  ( -0.5877852522924797984, -0.8090169943749425663, 0.000000000000000000 ) ) ;
#15938=ORIENTED_EDGE ( 'NONE', *, *, #19552, .T. ) ;
#15942=ADVANCED_FACE ( 'NONE', ( #24673 ), #18976, .T. ) ;
#15943=CARTESIAN_POINT ( 'NONE',  ( -0.4999999999999998890, 37.00000000000000711, 7.000000000000000000 ) ) ;
#15944=CIRCLE ( 'NONE', #12081, 15.00000000000000000 ) ;
#15945=ORIENTED_EDGE ( 'NONE', *, *, #9844, .F. ) ;
#15948=AXIS2_PLACEMENT_3D ( 'NONE', #11074, #29152, #13703 ) ;
#15949=CIRCLE ( 'NONE', #23100, 0.4999999999999998335 ) ;
#15951=VERTEX_POINT ( 'NONE', #34026 ) ;
#15954=ORIENTED_EDGE ( 'NONE', *, *, #662, .T. ) ;
#15955=EDGE_CURVE ( 'NONE', #37418, #28046, #3532, .T. ) ;
#15957=CARTESIAN_POINT ( 'NONE',  ( 12.99377146717206344, 26.19620116591418224, 10.50000000000000000 ) ) ;
#15958=CARTESIAN_POINT ( 'NONE',  ( 5.440908595777817602, 35.94977745735560859, 7.500000000000000888 ) ) ;
#15962=CARTESIAN_POINT ( 'NONE',  ( 14.41430201638238984, 20.48224166989774631, 10.99999999999999289 ) ) ;
#15963=CYLINDRICAL_SURFACE ( 'NONE', #30479, 0.4999999999999999445 ) ;
#15964=CARTESIAN_POINT ( 'NONE',  ( -3.597409820281606940, 14.42008525284352594, 7.000000000000000000 ) ) ;
#15965=PLANE ( 'NONE',  #4763 ) ;
#15966=CARTESIAN_POINT ( 'NONE',  ( 9.303655249773155944, 10.73386218874824216, 7.000000000000000000 ) ) ;
#15970=ORIENTED_EDGE ( 'NONE', *, *, #11235, .F. ) ;
#15973=CARTESIAN_POINT ( 'NONE',  ( 7.659620408498160060, 26.92228390473674793, 9.000000000000001776 ) ) ;
#15977=CARTESIAN_POINT ( 'NONE',  ( 8.927394655428274817, 11.06314620770945290, 7.000000000000000000 ) ) ;
#15981=LINE ( 'NONE', #15381, #2986 ) ;
#15990=CARTESIAN_POINT ( 'NONE',  ( -5.440908595777636414, 35.94977745735568675, 7.000000000000000000 ) ) ;
#15991=EDGE_CURVE ( 'NONE', #30348, #12011, #39341, .T. ) ;
#15993=ORIENTED_EDGE ( 'NONE', *, *, #34983, .F. ) ;
#15996=ORIENTED_EDGE ( 'NONE', *, *, #21290, .T. ) ;
#15997=DIRECTION ( 'NONE',  ( -0.6691306063588653430, -0.7431448254773878048, 0.000000000000000000 ) ) ;
#15998=CARTESIAN_POINT ( 'NONE',  ( 9.697889840765407499, 31.90483559858327212, 7.000000000000000000 ) ) ;
#16002=VECTOR ( 'NONE', #12676, 1000.000000000000000 ) ;
#16005=ORIENTED_EDGE ( 'NONE', *, *, #29264, .F. ) ;
#16006=EDGE_CURVE ( 'NONE', #31354, #400, #3930, .T. ) ;
#16007=CARTESIAN_POINT ( 'NONE',  ( -6.686869517299739663, 14.99761530854305391, 10.50000000000000533 ) ) ;
#16008=DIRECTION ( 'NONE',  ( -1.000000000000000000, 0.000000000000000000, 0.000000000000000000 ) ) ;
#16009=CARTESIAN_POINT ( 'NONE',  ( -4.003810537522578983, 8.420815593655365916, 10.49999999999999822 ) ) ;
#16010=EDGE_LOOP ( 'NONE', ( #35949, #4001, #39093 ) ) ;
#16012=CARTESIAN_POINT ( 'NONE',  ( -9.408554248005561504, 10.90613044664337572, 10.49999999999999467 ) ) ;
#16014=CARTESIAN_POINT ( 'NONE',  ( -4.727507481117100063, 31.88885898370948269, 10.00000000000000000 ) ) ;
#16015=DIRECTION ( 'NONE',  ( 1.000000000000000000, 0.000000000000000000, 0.000000000000000000 ) ) ;
#16016=CARTESIAN_POINT ( 'NONE',  ( 10.21785616688032583, 25.03138605371555414, 10.75000000000000000 ) ) ;
#16018=ORIENTED_EDGE ( 'NONE', *, *, #34596, .F. ) ;
#16020=DIRECTION ( 'NONE',  ( 0.000000000000000000, 0.000000000000000000, 1.000000000000000000 ) ) ;
#16022=LINE ( 'NONE', #13569, #12016 ) ;
#16026=DIRECTION ( 'NONE',  ( 0.6691306063588570163, -0.7431448254773953543, 0.000000000000000000 ) ) ;
#16032=CARTESIAN_POINT ( 'NONE',  ( 8.412270287199559604, 10.07085245822950448, 10.49999999999999822 ) ) ;
#16034=ORIENTED_EDGE ( 'NONE', *, *, #12718, .T. ) ;
#16036=DIRECTION ( 'NONE',  ( 0.2079116908177663092, 0.9781476007338042455, 0.000000000000000000 ) ) ;
#16037=AXIS2_PLACEMENT_3D ( 'NONE', #14775, #2185, #17638 ) ;
#16038=CARTESIAN_POINT ( 'NONE',  ( -0.6108529249775870307, 37.48755679569043053, 7.500000000000000888 ) ) ;
#16041=CARTESIAN_POINT ( 'NONE',  ( -14.33090402811213337, 26.16159042914076949, 10.49999999999999822 ) ) ;
#16042=DIRECTION ( 'NONE',  ( 0.6345370204113957024, -0.5138379476002926660, 0.5773502691896373884 ) ) ;
#16043=ORIENTED_EDGE ( 'NONE', *, *, #31988, .T. ) ;
#16046=ORIENTED_EDGE ( 'NONE', *, *, #37543, .T. ) ;
#16048=ORIENTED_EDGE ( 'NONE', *, *, #1108, .F. ) ;
#16050=DIRECTION ( 'NONE',  ( 0.000000000000000000, -0.000000000000000000, -1.000000000000000000 ) ) ;
#16051=DIRECTION ( 'NONE',  ( 0.000000000000000000, 0.000000000000000000, 1.000000000000000000 ) ) ;
#16055=AXIS2_PLACEMENT_3D ( 'NONE', #35526, #19886, #10951 ) ;
#16057=ORIENTED_EDGE ( 'NONE', *, *, #2091, .T. ) ;
#16058=DIRECTION ( 'NONE',  ( 0.4539904997395417530, 0.8910065241883703413, 0.000000000000000000 ) ) ;
#16060=DIRECTION ( 'NONE',  ( 1.000000000000000000, 0.000000000000000000, 0.000000000000000000 ) ) ;
#16063=AXIS2_PLACEMENT_3D ( 'NONE', #11704, #39918, #27537 ) ;
#16065=ORIENTED_EDGE ( 'NONE', *, *, #31754, .F. ) ;
#16067=DIRECTION ( 'NONE',  ( -0.5000000000000042188, -0.8660254037844361541, 0.000000000000000000 ) ) ;
#16068=CARTESIAN_POINT ( 'NONE',  ( -12.17073081513906985, 14.31852474926588670, 10.49999999999999645 ) ) ;
#16069=EDGE_CURVE ( 'NONE', #21179, #15193, #32246, .T. ) ;
#16070=EDGE_LOOP ( 'NONE', ( #11730, #24874, #26415 ) ) ;
#16074=ADVANCED_FACE ( 'NONE', ( #28916 ), #3727, .T. ) ;
#16076=VERTEX_POINT ( 'NONE', #31561 ) ;
#16077=ORIENTED_EDGE ( 'NONE', *, *, #13731, .F. ) ;
#16078=CIRCLE ( 'NONE', #11624, 0.5000000000000000000 ) ;
#16080=PLANE ( 'NONE',  #24980 ) ;
#16082=VECTOR ( 'NONE', #13839, 1000.000000000000227 ) ;
#16084=EDGE_CURVE ( 'NONE', #1489, #7593, #15747, .T. ) ;
#16088=ORIENTED_EDGE ( 'NONE', *, *, #17381, .F. ) ;
#16091=FACE_OUTER_BOUND ( 'NONE', #24834, .T. ) ;
#16092=AXIS2_PLACEMENT_3D ( 'NONE', #9012, #36647, #28089 ) ;
#16093=VERTEX_POINT ( 'NONE', #10228 ) ;
#16097=AXIS2_PLACEMENT_3D ( 'NONE', #33750, #8352, #36580 ) ;
#16100=ORIENTED_EDGE ( 'NONE', *, *, #31983, .T. ) ;
#16101=ADVANCED_FACE ( 'NONE', ( #10030 ), #29631, .T. ) ;
#16102=ADVANCED_FACE ( 'NONE', ( #22615 ), #32172, .F. ) ;
#16103=CARTESIAN_POINT ( 'NONE',  ( 3.295881626406574672, 9.398963235502481695, 10.00000000000000000 ) ) ;
#16104=EDGE_CURVE ( 'NONE', #11163, #34728, #16130, .T. ) ;
#16108=AXIS2_PLACEMENT_3D ( 'NONE', #32498, #2413, #2020 ) ;
#16109=CONICAL_SURFACE ( 'NONE', #35579, 1.000000000000000888, 0.7853981633974487231 ) ;
#16110=CARTESIAN_POINT ( 'NONE',  ( -11.30412111481561510, 32.00546000420963821, 10.94611345180490680 ) ) ;
#16115=CARTESIAN_POINT ( 'NONE',  ( -14.44707628845733005, 26.53512579137188609, 7.497105610438111967 ) ) ;
#16119=ORIENTED_EDGE ( 'NONE', *, *, #38670, .T. ) ;
#16122=EDGE_CURVE ( 'NONE', #37631, #12591, #3672, .T. ) ;
#16123=FACE_OUTER_BOUND ( 'NONE', #27620, .T. ) ;
#16125=ORIENTED_EDGE ( 'NONE', *, *, #13082, .F. ) ;
#16128=ORIENTED_EDGE ( 'NONE', *, *, #14867, .T. ) ;
#16130=LINE ( 'NONE', #1094, #6905 ) ;
#16133=ORIENTED_EDGE ( 'NONE', *, *, #37090, .T. ) ;
#16141=PLANE ( 'NONE',  #21844 ) ;
#16142=CARTESIAN_POINT ( 'NONE',  ( -10.66948297901429932, 33.02599466632846514, 10.49999999999999822 ) ) ;
#16143=ORIENTED_EDGE ( 'NONE', *, *, #9288, .F. ) ;
#16145=VECTOR ( 'NONE', #10809, 999.9999999999998863 ) ;
#16147=VECTOR ( 'NONE', #4500, 1000.000000000000114 ) ;
#16149=EDGE_LOOP ( 'NONE', ( #23938, #6043, #24350, #31144, #39187 ) ) ;
#16152=DIRECTION ( 'NONE',  ( 0.5254827454987487378, -0.4731467892558173238, 0.7071067811865534569 ) ) ;
#16154=EDGE_CURVE ( 'NONE', #20195, #9989, #33687, .T. ) ;
#16155=LINE ( 'NONE', #3559, #19746 ) ;
#16156=LINE ( 'NONE', #26089, #17561 ) ;
#16159=DIRECTION ( 'NONE',  ( -0.8090169943749504489, -0.5877852522924690293, 0.000000000000000000 ) ) ;
#16160=VERTEX_POINT ( 'NONE', #25862 ) ;
#16161=CARTESIAN_POINT ( 'NONE',  ( -6.492361549288664158, 35.85278612139737220, 10.87262190629282799 ) ) ;
#16165=FACE_OUTER_BOUND ( 'NONE', #39542, .T. ) ;
#16173=DIRECTION ( 'NONE',  ( 1.000000000000000000, 0.000000000000000000, 0.000000000000000000 ) ) ;
#16176=LINE ( 'NONE', #9875, #21757 ) ;
#16180=VECTOR ( 'NONE', #15258, 1000.000000000000000 ) ;
#16181=B_SPLINE_SURFACE_WITH_KNOTS ( 'NONE', 1, 3, ( 
 ( #20403, #14090, #32798, #4955, #39479, #14901, #29737, #2312, #26487, #23641 ),
 ( #24237, #14294, #2114, #30342, #26686, #26886, #38881, #2513, #36245, #11252 ) ),
 .UNSPECIFIED., .F., .F., .F.,
 ( 2, 2 ),
 ( 4, 2, 2, 2, 4 ),
 ( 0.000000000000000000, 1.000000000000000000 ),
 ( 4.237807397716013114, 4.630506479414739474, 5.023205561113466722, 5.415904642812193970, 5.808603724510920330 ),
 .UNSPECIFIED. ) ;
#16182=VERTEX_POINT ( 'NONE', #16739 ) ;
#16189=ORIENTED_EDGE ( 'NONE', *, *, #25481, .T. ) ;
#16196=ORIENTED_EDGE ( 'NONE', *, *, #23281, .F. ) ;
#16197=DIRECTION ( 'NONE',  ( 0.000000000000000000, 0.000000000000000000, -1.000000000000000000 ) ) ;
#16202=AXIS2_PLACEMENT_3D ( 'NONE', #3175, #13299, #37298 ) ;
#16203=ADVANCED_FACE ( 'NONE', ( #7372 ), #29324, .F. ) ;
#16204=ORIENTED_EDGE ( 'NONE', *, *, #21555, .F. ) ;
#16205=ORIENTED_EDGE ( 'NONE', *, *, #23363, .F. ) ;
#16206=VECTOR ( 'NONE', #33115, 1000.000000000000000 ) ;
#16207=CARTESIAN_POINT ( 'NONE',  ( 4.003793317224326742, 8.420815634768674229, 7.499999999999990230 ) ) ;
#16208=CARTESIAN_POINT ( 'NONE',  ( -2.421689871081827317, 8.701977744317861863, 9.500000000000000000 ) ) ;
#16209=DIRECTION ( 'NONE',  ( -0.5877852522924796874, -0.8090169943749426773, 0.000000000000000000 ) ) ;
#16210=ORIENTED_EDGE ( 'NONE', *, *, #691, .F. ) ;
#16211=ADVANCED_FACE ( 'NONE', ( #38464 ), #12774, .T. ) ;
#16213=EDGE_CURVE ( 'NONE', #13704, #7803, #2303, .T. ) ;
#16214=DIRECTION ( 'NONE',  ( 0.6123724356957989112, 0.3535533905932687349, -0.7071067811865463515 ) ) ;
#16215=LINE ( 'NONE', #13152, #27988 ) ;
#16216=EDGE_CURVE ( 'NONE', #113, #8524, #38061, .T. ) ;
#16217=DIRECTION ( 'NONE',  ( 0.6916548014802315070, 0.1470157664651950413, -0.7071067811865424657 ) ) ;
#16218=DIRECTION ( 'NONE',  ( 0.9781476007338043566, -0.2079116908177657264, 0.000000000000000000 ) ) ;
#16219=DIRECTION ( 'NONE',  ( -0.9781476007338042455, 0.2079116908177664758, 0.000000000000000000 ) ) ;
#16221=DIRECTION ( 'NONE',  ( -1.000000000000000000, 0.000000000000000000, 0.000000000000000000 ) ) ;
#16222=ORIENTED_EDGE ( 'NONE', *, *, #24007, .F. ) ;
#16227=CARTESIAN_POINT ( 'NONE',  ( -5.620290338810452369, 13.91368318151059214, 10.75000000000001066 ) ) ;
#16236=EDGE_CURVE ( 'NONE', #13390, #18096, #31564, .T. ) ;
#16238=LINE ( 'NONE', #28620, #31942 ) ;
#16243=CARTESIAN_POINT ( 'NONE',  ( 14.56494338438156610, 21.47191690367849048, 10.99387789255783687 ) ) ;
#16244=ORIENTED_EDGE ( 'NONE', *, *, #17367, .T. ) ;
#16246=FACE_OUTER_BOUND ( 'NONE', #32601, .T. ) ;
#16250=LINE ( 'NONE', #25381, #21560 ) ;
#16256=LINE ( 'NONE', #37389, #30712 ) ;
#16257=CARTESIAN_POINT ( 'NONE',  ( 6.557822374958316658, 35.99981354310111215, 10.49999999999999822 ) ) ;
#16258=EDGE_CURVE ( 'NONE', #16887, #32514, #17349, .T. ) ;
#16260=CARTESIAN_POINT ( 'NONE',  ( 14.36830325120613594, 20.48707633493483371, 9.000000000000001776 ) ) ;
#16261=VERTEX_POINT ( 'NONE', #29525 ) ;
#16265=CARTESIAN_POINT ( 'NONE',  ( -11.11016527260153808, 31.83082137946488643, 7.000000000000000000 ) ) ;
#16270=LINE ( 'NONE', #34558, #19118 ) ;
#16277=CARTESIAN_POINT ( 'NONE',  ( 0.000000000000000000, 22.50000000000000355, 7.000000000000000000 ) ) ;
#16279=VERTEX_POINT ( 'NONE', #20792 ) ;
#16280=ORIENTED_EDGE ( 'NONE', *, *, #35101, .F. ) ;
#16285=DIRECTION ( 'NONE',  ( 0.000000000000000000, 0.000000000000000000, -1.000000000000000000 ) ) ;
#16286=EDGE_LOOP ( 'NONE', ( #38908, #31570, #24032, #36025 ) ) ;
#16289=CARTESIAN_POINT ( 'NONE',  ( 14.76265446396241110, 21.90695576875680217, 10.49999999999999822 ) ) ;
#16290=CIRCLE ( 'NONE', #80, 15.00000000000000000 ) ;
#16291=ORIENTED_EDGE ( 'NONE', *, *, #17852, .F. ) ;
#16296=LINE ( 'NONE', #28682, #38849 ) ;
#16301=ADVANCED_FACE ( 'NONE', ( #1700 ), #32992, .T. ) ;
#16303=VECTOR ( 'NONE', #17879, 1000.000000000000000 ) ;
#16304=DIRECTION ( 'NONE',  ( 0.6691306063588569053, -0.7431448254773954654, 0.000000000000000000 ) ) ;
#16305=EDGE_CURVE ( 'NONE', #35366, #31091, #29726, .T. ) ;
#16306=VECTOR ( 'NONE', #27443, 1000.000000000000114 ) ;
#16307=EDGE_CURVE ( 'NONE', #13873, #4778, #7979, .T. ) ;
#16308=FACE_OUTER_BOUND ( 'NONE', #21881, .T. ) ;
#16314=DIRECTION ( 'NONE',  ( -0.9335804264971965249, 0.3583679495453138131, 0.000000000000000000 ) ) ;
#16315=VERTEX_POINT ( 'NONE', #14689 ) ;
#16317=ORIENTED_EDGE ( 'NONE', *, *, #5023, .F. ) ;
#16320=CARTESIAN_POINT ( 'NONE',  ( 10.81260707898150208, 32.90853150812155548, 10.49999999999999645 ) ) ;
#16326=ORIENTED_EDGE ( 'NONE', *, *, #17564, .F. ) ;
#16331=CARTESIAN_POINT ( 'NONE',  ( 12.62480652560819472, 14.42233381811226600, 10.49999999999999822 ) ) ;
#16333=CIRCLE ( 'NONE', #19574, 1.000000000000002665 ) ;
#16339=EDGE_LOOP ( 'NONE', ( #17311, #38210, #34760 ) ) ;
#16341=CARTESIAN_POINT ( 'NONE',  ( 13.24038105676655164, 15.43301270189216368, 10.49999999999999822 ) ) ;
#16342=DIRECTION ( 'NONE',  ( 0.000000000000000000, 0.000000000000000000, -1.000000000000000000 ) ) ;
#16343=ORIENTED_EDGE ( 'NONE', *, *, #37701, .F. ) ;
#16348=AXIS2_PLACEMENT_3D ( 'NONE', #16907, #111, #10197 ) ;
#16350=EDGE_CURVE ( 'NONE', #38194, #25405, #32896, .T. ) ;
#16351=DIRECTION ( 'NONE',  ( 1.000000000000000000, 0.000000000000000000, 0.000000000000000000 ) ) ;
#16353=ADVANCED_FACE ( 'NONE', ( #29923 ), #2104, .T. ) ;
#16354=ORIENTED_EDGE ( 'NONE', *, *, #13240, .T. ) ;
#16356=DIRECTION ( 'NONE',  ( 0.000000000000000000, 0.000000000000000000, -1.000000000000000000 ) ) ;
#16359=CARTESIAN_POINT ( 'NONE',  ( 14.60301432615392514, 21.46791548645758141, 11.00000000000000178 ) ) ;
#16361=CARTESIAN_POINT ( 'NONE',  ( 12.03571151536236528, 31.45218678977230908, 7.000000000000000000 ) ) ;
#16364=CARTESIAN_POINT ( 'NONE',  ( 14.62786683182123859, 20.45979510329145157, 10.94611345180490503 ) ) ;
#16365=CARTESIAN_POINT ( 'NONE',  ( 1.000000000000000000, 37.50000000000000711, 11.00000000000000000 ) ) ;
#16370=FACE_OUTER_BOUND ( 'NONE', #9504, .T. ) ;
#16371=CARTESIAN_POINT ( 'NONE',  ( 13.23567246089205618, 15.94827353676168613, 10.49999999999999822 ) ) ;
#16374=CARTESIAN_POINT ( 'NONE',  ( 14.36830325120613239, 20.48707633493482660, 11.00000000000000000 ) ) ;
#16378=ORIENTED_EDGE ( 'NONE', *, *, #3168, .T. ) ;
#16380=FACE_OUTER_BOUND ( 'NONE', #34153, .T. ) ;
#16384=VECTOR ( 'NONE', #25367, 1000.000000000000000 ) ;
#16392=EDGE_LOOP ( 'NONE', ( #22557, #25631, #33870, #19682, #35178 ) ) ;
#16395=ORIENTED_EDGE ( 'NONE', *, *, #22788, .F. ) ;
#16400=EDGE_CURVE ( 'NONE', #22349, #13390, #21221, .T. ) ;
#16403=ORIENTED_EDGE ( 'NONE', *, *, #10340, .F. ) ;
#16404=CARTESIAN_POINT ( 'NONE',  ( 11.11016527260166420, 31.83082137946473367, 9.000000000000001776 ) ) ;
#16406=AXIS2_PLACEMENT_3D ( 'NONE', #25276, #37669, #13072 ) ;
#16407=LINE ( 'NONE', #1170, #1956 ) ;
#16410=DIRECTION ( 'NONE',  ( 0.9781476007338070211, 0.2079116908177534029, -0.000000000000000000 ) ) ;
#16411=DIRECTION ( 'NONE',  ( 0.3090169943749573878, 0.9510565162951503115, 0.000000000000000000 ) ) ;
#16412=CARTESIAN_POINT ( 'NONE',  ( 8.472151273871505239, 28.78272654129060371, 10.50000000000000000 ) ) ;
#16413=FACE_OUTER_BOUND ( 'NONE', #5296, .T. ) ;
#16414=VECTOR ( 'NONE', #21461, 999.9999999999998863 ) ;
#16415=DIRECTION ( 'NONE',  ( 0.000000000000000000, -0.5821182788257928120, 0.8131041196900287149 ) ) ;
#16417=CARTESIAN_POINT ( 'NONE',  ( 2.363107919609636731, 7.722275577008987035, 10.49999999999999822 ) ) ;
#16418=ORIENTED_EDGE ( 'NONE', *, *, #35361, .F. ) ;
#16420=CARTESIAN_POINT ( 'NONE',  ( -10.70158575030358072, 30.79011836036732674, 9.500000000000000000 ) ) ;
#16423=FACE_OUTER_BOUND ( 'NONE', #10747, .T. ) ;
#16432=ADVANCED_FACE ( 'NONE', ( #6673 ), #25249, .T. ) ;
#16434=DIRECTION ( 'NONE',  ( -0.000000000000000000, -0.000000000000000000, -1.000000000000000000 ) ) ;
#16436=ORIENTED_EDGE ( 'NONE', *, *, #8273, .F. ) ;
#16439=CARTESIAN_POINT ( 'NONE',  ( 14.66026487122505451, 21.46189821169926759, 10.96580508970281542 ) ) ;
#16440=ORIENTED_EDGE ( 'NONE', *, *, #15801, .F. ) ;
#16443=DIRECTION ( 'NONE',  ( 1.000000000000000000, 0.000000000000000000, 0.000000000000000000 ) ) ;
#16445=ADVANCED_FACE ( 'NONE', ( #25175 ), #31090, .T. ) ;
#16446=VERTEX_POINT ( 'NONE', #34719 ) ;
#16449=AXIS2_PLACEMENT_3D ( 'NONE', #5178, #38905, #2136 ) ;
#16457=CARTESIAN_POINT ( 'NONE',  ( -3.996141029131407230, 8.041929616041358031, 7.381627713044569106 ) ) ;
#16459=AXIS2_PLACEMENT_3D ( 'NONE', #20477, #26153, #25948 ) ;
#16460=CARTESIAN_POINT ( 'NONE',  ( -11.44473057578096764, 31.45924896672619298, 10.49999999999999822 ) ) ;
#16461=EDGE_LOOP ( 'NONE', ( #12645, #26156, #18657, #4073 ) ) ;
#16462=SURFACE_STYLE_FILL_AREA ( #38195 ) ;
#16466=EDGE_CURVE ( 'NONE', #15571, #26406, #3635, .T. ) ;
#16467=DIRECTION ( 'NONE',  ( -0.000000000000000000, -0.000000000000000000, -1.000000000000000000 ) ) ;
#16474=DIRECTION ( 'NONE',  ( 0.8090169943749426773, -0.5877852522924797984, 0.000000000000000000 ) ) ;
#16475=DIRECTION ( 'NONE',  ( 0.7431448254773954654, 0.6691306063588569053, -0.000000000000000000 ) ) ;
#16476=EDGE_LOOP ( 'NONE', ( #22077, #4663, #1331, #26554 ) ) ;
#16478=VECTOR ( 'NONE', #3956, 1000.000000000000000 ) ;
#16481=CARTESIAN_POINT ( 'NONE',  ( -7.935100905948476502, 11.57827057593827469, 7.000000000000000000 ) ) ;
#16482=ORIENTED_EDGE ( 'NONE', *, *, #32983, .T. ) ;
#16486=EDGE_CURVE ( 'NONE', #31354, #23547, #17712, .T. ) ;
#16488=AXIS2_PLACEMENT_3D ( 'NONE', #21168, #28055, #15468 ) ;
#16490=CARTESIAN_POINT ( 'NONE',  ( -5.473344025737326035, 14.11593743010433677, 10.50000000000000355 ) ) ;
#16495=DIRECTION ( 'NONE',  ( -0.000000000000000000, -0.000000000000000000, -1.000000000000000000 ) ) ;
#16499=CARTESIAN_POINT ( 'NONE',  ( -1.278175571584109660, 14.08178954835378427, 9.000000000000001776 ) ) ;
#16502=AXIS2_PLACEMENT_3D ( 'NONE', #26141, #23096, #7658 ) ;
#16503=DIRECTION ( 'NONE',  ( 1.000000000000000000, 0.000000000000000000, 0.000000000000000000 ) ) ;
#16505=VERTEX_POINT ( 'NONE', #26173 ) ;
#16507=DIRECTION ( 'NONE',  ( -0.9945218953682742891, -0.1045284632676437425, 0.000000000000000000 ) ) ;
#16509=CIRCLE ( 'NONE', #3510, 1.000000000000004441 ) ;
#16510=FACE_OUTER_BOUND ( 'NONE', #35025, .T. ) ;
#16513=EDGE_CURVE ( 'NONE', #39537, #15233, #7691, .T. ) ;
#16515=CIRCLE ( 'NONE', #32738, 0.5000000000000015543 ) ;
#16520=DIRECTION ( 'NONE',  ( 1.000000000000000000, 1.224646799147351235E-16, -0.000000000000000000 ) ) ;
#16526=CARTESIAN_POINT ( 'NONE',  ( 10.81260707898162821, 32.90853150812142047, 10.59344459855564047 ) ) ;
#16528=VERTEX_POINT ( 'NONE', #17252 ) ;
#16530=CARTESIAN_POINT ( 'NONE',  ( 14.47283171447379502, 21.48159823030311344, 9.000000000000001776 ) ) ;
#16531=EDGE_LOOP ( 'NONE', ( #33793, #25882, #20033, #25029 ) ) ;
#16533=CARTESIAN_POINT ( 'NONE',  ( -14.47283171447380390, 21.48159823030330529, 11.00000000000000000 ) ) ;
#16537=VERTEX_POINT ( 'NONE', #1395 ) ;
#16540=FACE_OUTER_BOUND ( 'NONE', #7544, .T. ) ;
#16544=FACE_OUTER_BOUND ( 'NONE', #24680, .T. ) ;
#16545=CARTESIAN_POINT ( 'NONE',  ( -14.44277748876676881, 26.55045409923033972, 7.499999999999993783 ) ) ;
#16547=ORIENTED_EDGE ( 'NONE', *, *, #15991, .T. ) ;
#16552=EDGE_LOOP ( 'NONE', ( #32863, #36815, #22860, #25352 ) ) ;
#16553=VECTOR ( 'NONE', #7006, 1000.000000000000000 ) ;
#16555=DIRECTION ( 'NONE',  ( 0.000000000000000000, 0.000000000000000000, 1.000000000000000000 ) ) ;
#16556=VECTOR ( 'NONE', #2182, 999.9999999999998863 ) ;
#16557=VECTOR ( 'NONE', #25864, 1000.000000000000000 ) ;
#16559=CARTESIAN_POINT ( 'NONE',  ( 13.48130249190479191, 27.93180293473185927, 7.000000000000000000 ) ) ;
#16561=CARTESIAN_POINT ( 'NONE',  ( 5.187504188494417079, 36.60991850771481637, 10.49999999999999467 ) ) ;
#16564=ORIENTED_EDGE ( 'NONE', *, *, #15247, .T. ) ;
#16568=CARTESIAN_POINT ( 'NONE',  ( -22.37674264578614469, 24.85189042352228839, 7.000000000000000000 ) ) ;
#16569=CARTESIAN_POINT ( 'NONE',  ( 9.331903152615748098, 11.35703883385568780, 7.500000000000000888 ) ) ;
#16570=B_SPLINE_CURVE_WITH_KNOTS ( 'NONE', 3,
 ( #29185, #4801, #13535, #37574, #35884, #1761, #1152, #7434 ),
 .UNSPECIFIED., .F., .F.,
 ( 4, 2, 2, 4 ),
 ( 0.000000000000000000, 0.0004726692273637163929, 0.0007090038410455775167, 0.0009453384547274386405 ),
 .UNSPECIFIED. ) ;
#16571=AXIS2_PLACEMENT_3D ( 'NONE', #20936, #17704, #29676 ) ;
#16573=DIRECTION ( 'NONE',  ( -0.6691306063588671194, -0.7431448254773863615, 0.000000000000000000 ) ) ;
#16574=ORIENTED_EDGE ( 'NONE', *, *, #18184, .F. ) ;
#16578=CARTESIAN_POINT ( 'NONE',  ( 7.713869163865849643, 10.18146832927074996, 11.00000000000000000 ) ) ;
#16580=ORIENTED_EDGE ( 'NONE', *, *, #5799, .F. ) ;
#16585=CARTESIAN_POINT ( 'NONE',  ( 13.94482798346721175, 26.50521816028912525, 10.99999999999999289 ) ) ;
#16587=EDGE_CURVE ( 'NONE', #3128, #9203, #16642, .T. ) ;
#16592=ORIENTED_EDGE ( 'NONE', *, *, #27775, .F. ) ;
#16593=EDGE_CURVE ( 'NONE', #31286, #4629, #25096, .T. ) ;
#16600=EDGE_CURVE ( 'NONE', #3128, #34232, #35521, .T. ) ;
#16601=CYLINDRICAL_SURFACE ( 'NONE', #38410, 0.5000000000000002220 ) ;
#16602=ORIENTED_EDGE ( 'NONE', *, *, #18565, .T. ) ;
#16608=ORIENTED_EDGE ( 'NONE', *, *, #39999, .T. ) ;
#16611=FACE_OUTER_BOUND ( 'NONE', #32335, .T. ) ;
#16612=EDGE_CURVE ( 'NONE', #34166, #15690, #4238, .T. ) ;
#16614=AXIS2_PLACEMENT_3D ( 'NONE', #37753, #3821, #34907 ) ;
#16616=DIRECTION ( 'NONE',  ( -8.659560562354955045E-17, 0.7071067811865489050, -0.7071067811865462405 ) ) ;
#16621=CARTESIAN_POINT ( 'NONE',  ( 12.67417846324118180, 14.47720745114811258, 7.000000000000000000 ) ) ;
#16622=DIRECTION ( 'NONE',  ( 0.6724985119639532716, 0.2185080122244073830, -0.7071067811865523467 ) ) ;
#16623=CARTESIAN_POINT ( 'NONE',  ( -10.44103466624267185, 32.57396620494226624, 7.000000000000000000 ) ) ;
#16624=CYLINDRICAL_SURFACE ( 'NONE', #16459, 6.000000000000005329 ) ;
#16626=DIRECTION ( 'NONE',  ( 0.9781476007338042455, -0.2079116908177656431, 0.000000000000000000 ) ) ;
#16627=EDGE_LOOP ( 'NONE', ( #3333, #1044, #34409, #21155 ) ) ;
#16629=CARTESIAN_POINT ( 'NONE',  ( 9.356056665764066693, 26.06569820189703179, 10.49999999999999822 ) ) ;
#16632=DIRECTION ( 'NONE',  ( 0.5877852522924690293, -0.8090169943749504489, 0.000000000000000000 ) ) ;
#16636=EDGE_CURVE ( 'NONE', #12323, #36981, #26405, .T. ) ;
#16640=EDGE_CURVE ( 'NONE', #25293, #37715, #13985, .T. ) ;
#16642=LINE ( 'NONE', #35120, #19917 ) ;
#16643=DIRECTION ( 'NONE',  ( -1.000000000000000000, 0.000000000000000000, 0.000000000000000000 ) ) ;
#16644=ORIENTED_EDGE ( 'NONE', *, *, #8926, .F. ) ;
#16646=ORIENTED_EDGE ( 'NONE', *, *, #3667, .F. ) ;
#16648=CARTESIAN_POINT ( 'NONE',  ( 14.97009266215789758, 21.42933399866903699, 10.59344459855564580 ) ) ;
#16649=ORIENTED_EDGE ( 'NONE', *, *, #12994, .F. ) ;
#16651=DIRECTION ( 'NONE',  ( 0.6691306063588687847, 0.7431448254773848072, 0.000000000000000000 ) ) ;
#16655=EDGE_LOOP ( 'NONE', ( #37048, #38889, #22541, #32741 ) ) ;
#16657=ORIENTED_EDGE ( 'NONE', *, *, #38570, .T. ) ;
#16660=DIRECTION ( 'NONE',  ( -0.4067366430757888840, 0.9135454576426059736, 0.000000000000000000 ) ) ;
#16661=CARTESIAN_POINT ( 'NONE',  ( -0.4999999999999995559, 37.00000000000000711, 11.00000000000000000 ) ) ;
#16666=CARTESIAN_POINT ( 'NONE',  ( 3.503793317224327186, 8.420815634768674229, 7.499999999999990230 ) ) ;
#16668=ADVANCED_FACE ( 'NONE', ( #38365 ), #6303, .T. ) ;
#16669=B_SPLINE_CURVE_WITH_KNOTS ( 'NONE', 3,
 ( #1424, #26200, #38595, #32915, #36155, #27403 ),
 .UNSPECIFIED., .F., .F.,
 ( 4, 2, 4 ),
 ( 0.000000000000000000, 0.4999999999999988898, 1.000000000000000000 ),
 .UNSPECIFIED. ) ;
#16672=VECTOR ( 'NONE', #9248, 999.9999999999998863 ) ;
#16676=DIRECTION ( 'NONE',  ( -0.6459741880212513943, 0.2876062384759537349, -0.7071067811865459074 ) ) ;
#16677=CARTESIAN_POINT ( 'NONE',  ( -1.000000000000000000, 37.00000000000000711, 10.50000000000000178 ) ) ;
#16685=CARTESIAN_POINT ( 'NONE',  ( 0.5000000000000001110, 33.00000000000000000, 11.00000000000000000 ) ) ;
#16686=ORIENTED_EDGE ( 'NONE', *, *, #21798, .T. ) ;
#16692=CARTESIAN_POINT ( 'NONE',  ( -13.55123249967971510, 16.06769038696092622, 7.165319362607849740 ) ) ;
#16697=ADVANCED_FACE ( 'NONE', ( #23337 ), #19267, .T. ) ;
#16701=ORIENTED_EDGE ( 'NONE', *, *, #39444, .T. ) ;
#16703=CIRCLE ( 'NONE', #39395, 0.9999999999999994449 ) ;
#16704=AXIS2_PLACEMENT_3D ( 'NONE', #14391, #11548, #5044 ) ;
#16709=VECTOR ( 'NONE', #10251, 1000.000000000000000 ) ;
#16711=FACE_OUTER_BOUND ( 'NONE', #21398, .T. ) ;
#16713=VECTOR ( 'NONE', #3176, 1000.000000000000114 ) ;
#16715=EDGE_CURVE ( 'NONE', #6329, #4036, #18648, .T. ) ;
#16716=DIRECTION ( 'NONE',  ( 0.000000000000000000, 0.000000000000000000, 1.000000000000000000 ) ) ;
#16723=CARTESIAN_POINT ( 'NONE',  ( -13.13294332834922251, 16.07239217250488750, 10.49999999999999822 ) ) ;
#16726=AXIS2_PLACEMENT_3D ( 'NONE', #15845, #9352, #5695 ) ;
#16727=ORIENTED_EDGE ( 'NONE', *, *, #10369, .T. ) ;
#16731=CARTESIAN_POINT ( 'NONE',  ( -1.590043107810761525, 12.61456814725308817, 10.50000000000001066 ) ) ;
#16736=VERTEX_POINT ( 'NONE', #30640 ) ;
#16737=AXIS2_PLACEMENT_3D ( 'NONE', #36347, #8511, #27198 ) ;
#16739=CARTESIAN_POINT ( 'NONE',  ( 6.572794801194151049, 16.58182897866491956, 7.000000000000000000 ) ) ;
#16741=DIRECTION ( 'NONE',  ( 0.3090169943749573878, 0.9510565162951503115, 0.000000000000000000 ) ) ;
#16743=ORIENTED_EDGE ( 'NONE', *, *, #7884, .T. ) ;
#16746=CARTESIAN_POINT ( 'NONE',  ( 0.5000000000000001110, 37.00000000000000711, 7.000000000000000000 ) ) ;
#16748=ORIENTED_EDGE ( 'NONE', *, *, #38451, .T. ) ;
#16750=DIRECTION ( 'NONE',  ( -1.000000000000000000, 0.000000000000000000, 0.000000000000000000 ) ) ;
#16751=EDGE_CURVE ( 'NONE', #11294, #33679, #37457, .T. ) ;
#16753=ADVANCED_FACE ( 'NONE', ( #17455 ), #25131, .T. ) ;
#16754=VERTEX_POINT ( 'NONE', #33093 ) ;
#16758=VERTEX_POINT ( 'NONE', #30236 ) ;
#16760=CARTESIAN_POINT ( 'NONE',  ( -6.762317648414995830, 29.93445088906605989, 10.49999999999999822 ) ) ;
#16762=VECTOR ( 'NONE', #23031, 1000.000000000000000 ) ;
#16763=DIRECTION ( 'NONE',  ( 0.000000000000000000, 0.000000000000000000, 1.000000000000000000 ) ) ;
#16766=ADVANCED_FACE ( 'NONE', ( #8897 ), #8902, .T. ) ;
#16769=LINE ( 'NONE', #1320, #8783 ) ;
#16770=ORIENTED_EDGE ( 'NONE', *, *, #34881, .F. ) ;
#16771=CARTESIAN_POINT ( 'NONE',  ( 10.10646936306337729, 32.94553861768082470, 10.49999999999999645 ) ) ;
#16772=CARTESIAN_POINT ( 'NONE',  ( -8.118377661053489902, 10.47536095541709322, 7.000000000000000000 ) ) ;
#16774=LINE ( 'NONE', #25492, #3074 ) ;
#16775=DIRECTION ( 'NONE',  ( -0.6691306063588670083, -0.7431448254773863615, 0.000000000000000000 ) ) ;
#16777=DIRECTION ( 'NONE',  ( 0.6691306063588678965, 0.7431448254773855844, 0.000000000000000000 ) ) ;
#16778=ORIENTED_EDGE ( 'NONE', *, *, #1565, .T. ) ;
#16788=CARTESIAN_POINT ( 'NONE',  ( 14.39395135575595042, 26.65114718998425047, 10.68306085400107719 ) ) ;
#16791=VECTOR ( 'NONE', #34120, 999.9999999999998863 ) ;
#16807=DIRECTION ( 'NONE',  ( 1.000000000000000000, 0.000000000000000000, 0.000000000000000000 ) ) ;
#16812=ORIENTED_EDGE ( 'NONE', *, *, #2222, .T. ) ;
#16813=DIRECTION ( 'NONE',  ( -0.000000000000000000, -0.000000000000000000, 1.000000000000000000 ) ) ;
#16817=LINE ( 'NONE', #5017, #11690 ) ;
#16821=CYLINDRICAL_SURFACE ( 'NONE', #17874, 0.4999999999999997780 ) ;
#16823=ADVANCED_FACE ( 'NONE', ( #36331 ), #11350, .T. ) ;
#16824=VECTOR ( 'NONE', #38795, 1000.000000000000114 ) ;
#16825=CARTESIAN_POINT ( 'NONE',  ( 12.83926296998458128, 26.67172942406175906, 7.000000000000000000 ) ) ;
#16826=LINE ( 'NONE', #19869, #30783 ) ;
#16827=CARTESIAN_POINT ( 'NONE',  ( -14.91782843052412488, 20.93207305098534832, 7.000000000000000000 ) ) ;
#16829=FACE_OUTER_BOUND ( 'NONE', #852, .T. ) ;
#16833=FACE_OUTER_BOUND ( 'NONE', #366, .T. ) ;
#16834=CARTESIAN_POINT ( 'NONE',  ( -14.11133924723972655, 27.61078317377209501, 10.59344459855564757 ) ) ;
#16836=CARTESIAN_POINT ( 'NONE',  ( 12.80736835487433289, 15.68301270189216545, 7.499999999999997335 ) ) ;
#16839=CARTESIAN_POINT ( 'NONE',  ( 0.000000000000000000, 22.50000000000000355, 7.000000000000000000 ) ) ;
#16846=EDGE_CURVE ( 'NONE', #22802, #23608, #24131, .T. ) ;
#16847=VERTEX_POINT ( 'NONE', #8699 ) ;
#16849=EDGE_CURVE ( 'NONE', #16537, #19499, #26777, .T. ) ;
#16850=ORIENTED_EDGE ( 'NONE', *, *, #19505, .T. ) ;
#16852=EDGE_CURVE ( 'NONE', #35202, #13016, #34213, .T. ) ;
#16853=VECTOR ( 'NONE', #37104, 1000.000000000000114 ) ;
#16854=DIRECTION ( 'NONE',  ( -1.000000000000000000, 0.000000000000000000, 0.000000000000000000 ) ) ;
#16855=ORIENTED_EDGE ( 'NONE', *, *, #19639, .F. ) ;
#16857=CARTESIAN_POINT ( 'NONE',  ( -7.929471891321299815, 25.60217271033470965, 7.000000000000000000 ) ) ;
#16858=CARTESIAN_POINT ( 'NONE',  ( -8.411683849014160330, 19.76687823897114882, 9.000000000000001776 ) ) ;
#16859=AXIS2_PLACEMENT_3D ( 'NONE', #14814, #32912, #32712 ) ;
#16860=VERTEX_POINT ( 'NONE', #33499 ) ;
#16862=ORIENTED_EDGE ( 'NONE', *, *, #22710, .T. ) ;
#16864=VERTEX_POINT ( 'NONE', #20894 ) ;
#16866=CARTESIAN_POINT ( 'NONE',  ( -8.412270287199726582, 10.07085245822961994, 7.000000000000000000 ) ) ;
#16870=CARTESIAN_POINT ( 'NONE',  ( -1.642021030515208979, 12.37003124706962787, 10.75000000000001421 ) ) ;
#16871=ORIENTED_EDGE ( 'NONE', *, *, #33612, .T. ) ;
#16876=CYLINDRICAL_SURFACE ( 'NONE', #28584, 6.000000000000014211 ) ;
#16879=VECTOR ( 'NONE', #23969, 1000.000000000000227 ) ;
#16880=ORIENTED_EDGE ( 'NONE', *, *, #11766, .T. ) ;
#16882=CARTESIAN_POINT ( 'NONE',  ( 7.929471891321336230, 25.60217271033461373, 7.000000000000000000 ) ) ;
#16886=CARTESIAN_POINT ( 'NONE',  ( 1.000000000000000222, 36.50000000000000711, 10.50000000000000000 ) ) ;
#16887=VERTEX_POINT ( 'NONE', #39966 ) ;
#16893=ORIENTED_EDGE ( 'NONE', *, *, #11180, .T. ) ;
#16896=CARTESIAN_POINT ( 'NONE',  ( -12.51373512357471363, 14.69784138864699230, 10.94387467463490893 ) ) ;
#16897=VECTOR ( 'NONE', #25989, 1000.000000000000000 ) ;
#16900=EDGE_LOOP ( 'NONE', ( #30681, #39483, #16418, #38369 ) ) ;
#16903=CARTESIAN_POINT ( 'NONE',  ( -9.892954722048921568, 20.95745441963943634, 10.00000000000000000 ) ) ;
#16904=UNCERTAINTY_MEASURE_WITH_UNIT (LENGTH_MEASURE( 1.000000000000000082E-05 ), #13606, 'distance_accuracy_value', 'NONE');
#16907=CARTESIAN_POINT ( 'NONE',  ( 0.000000000000000000, 22.50000000000000355, 7.000000000000000000 ) ) ;
#16916=DIRECTION ( 'NONE',  ( -0.6916548014802318400, -0.1470157664651949581, -0.7071067811865421326 ) ) ;
#16919=DIRECTION ( 'NONE',  ( 0.8090169943749504489, 0.5877852522924690293, -0.000000000000000000 ) ) ;
#16923=VECTOR ( 'NONE', #40140, 1000.000000000000000 ) ;
#16927=DIRECTION ( 'NONE',  ( -0.8660254037844432595, -0.4999999999999921729, 0.000000000000000000 ) ) ;
#16930=EDGE_LOOP ( 'NONE', ( #17456, #40060, #35558 ) ) ;
#16935=ORIENTED_EDGE ( 'NONE', *, *, #3867, .F. ) ;
#16937=AXIS2_PLACEMENT_3D ( 'NONE', #36053, #32813, #30709 ) ;
#16940=CARTESIAN_POINT ( 'NONE',  ( -14.97009266215794199, 21.42933399866948463, 10.63089969389957545 ) ) ;
#16943=VERTEX_POINT ( 'NONE', #11945 ) ;
#16951=LINE ( 'NONE', #10240, #16762 ) ;
#16953=EDGE_LOOP ( 'NONE', ( #21391, #22305, #20717, #33011 ) ) ;
#16956=CIRCLE ( 'NONE', #18259, 1.000000000000000888 ) ;
#16957=EDGE_CURVE ( 'NONE', #25929, #21181, #9656, .T. ) ;
#16959=CIRCLE ( 'NONE', #26693, 6.000000000000003553 ) ;
#16962=EDGE_CURVE ( 'NONE', #14392, #18018, #29018, .T. ) ;
#16964=LINE ( 'NONE', #913, #23842 ) ;
#16967=DIRECTION ( 'NONE',  ( 0.5000000000000043299, 0.8660254037844361541, 0.000000000000000000 ) ) ;
#16968=CARTESIAN_POINT ( 'NONE',  ( 13.94482798346721175, 26.50521816028912525, 11.00000000000000000 ) ) ;
#16969=ORIENTED_EDGE ( 'NONE', *, *, #9017, .F. ) ;
#16970=EDGE_CURVE ( 'NONE', #12750, #26235, #9297, .T. ) ;
#16971=CARTESIAN_POINT ( 'NONE',  ( 8.910254037844364206, 17.93301270189218855, 10.50000000000000000 ) ) ;
#16972=EDGE_CURVE ( 'NONE', #29281, #18489, #28370, .T. ) ;
#16973=CARTESIAN_POINT ( 'NONE',  ( 3.829842517468933671, 8.490119531707911449, 10.66666666666666075 ) ) ;
#16975=DIRECTION ( 'NONE',  ( 0.000000000000000000, 0.000000000000000000, -1.000000000000000000 ) ) ;
#16979=ORIENTED_EDGE ( 'NONE', *, *, #20086, .T. ) ;
#16983=CIRCLE ( 'NONE', #15030, 15.00000000000000000 ) ;
#16987=EDGE_LOOP ( 'NONE', ( #22342, #5624, #2320, #11367, #8350, #23792, #16440 ) ) ;
#16989=EDGE_LOOP ( 'NONE', ( #17339, #32315, #22977, #38982 ) ) ;
#16997=ORIENTED_EDGE ( 'NONE', *, *, #969, .T. ) ;
#17000=VECTOR ( 'NONE', #27628, 1000.000000000000000 ) ;
#17002=CARTESIAN_POINT ( 'NONE',  ( 1.000000000000000000, 37.00000000000000711, 10.50000000000000178 ) ) ;
#17005=EDGE_CURVE ( 'NONE', #2692, #17841, #21875, .T. ) ;
#17007=ORIENTED_EDGE ( 'NONE', *, *, #13952, .T. ) ;
#17011=DIRECTION ( 'NONE',  ( 0.000000000000000000, 0.000000000000000000, 1.000000000000000000 ) ) ;
#17016=DIRECTION ( 'NONE',  ( 0.000000000000000000, 0.000000000000000000, 1.000000000000000000 ) ) ;
#17020=DIRECTION ( 'NONE',  ( -0.7032331762533995390, -0.07391278520355930304, -0.7071067811865530128 ) ) ;
#17021=EDGE_CURVE ( 'NONE', #30083, #17070, #33888, .T. ) ;
#17023=CIRCLE ( 'NONE', #21535, 0.5000000000000004441 ) ;
#17024=ADVANCED_FACE ( 'NONE', ( #22270 ), #2435, .T. ) ;
#17026=PLANE ( 'NONE',  #10005 ) ;
#17029=CARTESIAN_POINT ( 'NONE',  ( -12.53339520833721110, 14.68649063341707972, 10.94611345180490680 ) ) ;
#17030=ORIENTED_EDGE ( 'NONE', *, *, #34050, .T. ) ;
#17031=VECTOR ( 'NONE', #34925, 999.9999999999998863 ) ;
#17033=CARTESIAN_POINT ( 'NONE',  ( -12.14070168820776274, 14.52831216351308541, 10.66666666666666430 ) ) ;
#17034=CARTESIAN_POINT ( 'NONE',  ( -0.9658050764552030820, 37.18846563620834189, 10.49999999999999822 ) ) ;
#17036=CARTESIAN_POINT ( 'NONE',  ( 8.694801740383951483, 1.741858881503470569, 11.00000000000000000 ) ) ;
#17039=B_SPLINE_CURVE_WITH_KNOTS ( 'NONE', 3,
 ( #30332, #27672, #24031, #14691 ),
 .UNSPECIFIED., .F., .F.,
 ( 4, 4 ),
 ( 0.000000000000000000, 1.000000000000000000 ),
 .UNSPECIFIED. ) ;
#17040=DIRECTION ( 'NONE',  ( -0.000000000000000000, 0.000000000000000000, -1.000000000000000000 ) ) ;
#17042=AXIS2_PLACEMENT_3D ( 'NONE', #25442, #31947, #29107 ) ;
#17047=VERTEX_POINT ( 'NONE', #12339 ) ;
#17049=ORIENTED_EDGE ( 'NONE', *, *, #5045, .F. ) ;
#17050=ADVANCED_FACE ( 'NONE', ( #6241 ), #24727, .T. ) ;
#17051=DIRECTION ( 'NONE',  ( 0.5254827454987599511, 0.4731467892558155475, -0.7071067811865464625 ) ) ;
#17052=ORIENTED_EDGE ( 'NONE', *, *, #10865, .T. ) ;
#17054=AXIS2_PLACEMENT_3D ( 'NONE', #4906, #33153, #20354 ) ;
#17055=EDGE_CURVE ( 'NONE', #27384, #1404, #28056, .T. ) ;
#17059=ORIENTED_EDGE ( 'NONE', *, *, #16715, .F. ) ;
#17061=CIRCLE ( 'NONE', #22227, 0.5000000000000004441 ) ;
#17066=LINE ( 'NONE', #29042, #35901 ) ;
#17069=CARTESIAN_POINT ( 'NONE',  ( -11.56932667689144267, 32.06810925246628585, 10.49999999999999822 ) ) ;
#17070=VERTEX_POINT ( 'NONE', #24932 ) ;
#17071=VECTOR ( 'NONE', #8777, 1000.000000000000000 ) ;
#17072=DIRECTION ( 'NONE',  ( 0.000000000000000000, 0.000000000000000000, 1.000000000000000000 ) ) ;
#17073=LINE ( 'NONE', #35757, #97 ) ;
#17082=DIRECTION ( 'NONE',  ( 0.000000000000000000, 0.000000000000000000, -1.000000000000000000 ) ) ;
#17083=CIRCLE ( 'NONE', #33304, 15.00000000000000000 ) ;
#17086=DIRECTION ( 'NONE',  ( -0.4156269377774634011, 0.5720614028176739252, -0.7071067811865500152 ) ) ;
#17089=VECTOR ( 'NONE', #9563, 1000.000000000000000 ) ;
#17094=ORIENTED_EDGE ( 'NONE', *, *, #1920, .T. ) ;
#17096=CARTESIAN_POINT ( 'NONE',  ( 4.155936879284735319, 47.29106893214565588, 9.500000000000000000 ) ) ;
#17097=ADVANCED_FACE ( 'NONE', ( #15389 ), #20597, .T. ) ;
#17101=LINE ( 'NONE', #35984, #29308 ) ;
#17102=ORIENTED_EDGE ( 'NONE', *, *, #367, .F. ) ;
#17105=CARTESIAN_POINT ( 'NONE',  ( -10.73132186042470160, 32.83534196859154974, 10.82238861112338490 ) ) ;
#17106=DIRECTION ( 'NONE',  ( -0.5720614028176844723, -0.4156269377774491347, -0.7071067811865499042 ) ) ;
#17107=CARTESIAN_POINT ( 'NONE',  ( -2.046188276595982014, 8.063706679521100540, 10.49999999999999822 ) ) ;
#17108=ORIENTED_EDGE ( 'NONE', *, *, #40024, .T. ) ;
#17110=FACE_OUTER_BOUND ( 'NONE', #7869, .T. ) ;
#17120=CARTESIAN_POINT ( 'NONE',  ( -9.031213237790245429, -0.7484781929866335393, 9.500000000000000000 ) ) ;
#17123=FACE_OUTER_BOUND ( 'NONE', #38664, .T. ) ;
#17124=ORIENTED_EDGE ( 'NONE', *, *, #27301, .T. ) ;
#17126=ADVANCED_FACE ( 'NONE', ( #12934 ), #14762, .T. ) ;
#17129=DIRECTION ( 'NONE',  ( -0.4067366430758047602, -0.9135454576425988682, 7.055756032835973512E-16 ) ) ;
#17130=VECTOR ( 'NONE', #1681, 1000.000000000000000 ) ;
#17133=CYLINDRICAL_SURFACE ( 'NONE', #29475, 0.5000000000000006661 ) ;
#17141=CARTESIAN_POINT ( 'NONE',  ( -14.03291393139908649, 26.53383901973369774, 10.99387789255785641 ) ) ;
#17145=ORIENTED_EDGE ( 'NONE', *, *, #17641, .F. ) ;
#17149=DIRECTION ( 'NONE',  ( 0.000000000000000000, 0.000000000000000000, -1.000000000000000000 ) ) ;
#17152=ORIENTED_EDGE ( 'NONE', *, *, #27047, .T. ) ;
#17157=ORIENTED_EDGE ( 'NONE', *, *, #17566, .T. ) ;
#17159=EDGE_CURVE ( 'NONE', #12954, #22450, #35482, .T. ) ;
#17162=ORIENTED_EDGE ( 'NONE', *, *, #21242, .F. ) ;
#17165=AXIS2_PLACEMENT_3D ( 'NONE', #38143, #10516, #16218 ) ;
#17170=VECTOR ( 'NONE', #22057, 1000.000000000000000 ) ;
#17172=FACE_OUTER_BOUND ( 'NONE', #38201, .T. ) ;
#17176=CARTESIAN_POINT ( 'NONE',  ( -7.713869163866016621, 10.18146832927085121, 7.500000000000000888 ) ) ;
#17177=VERTEX_POINT ( 'NONE', #23083 ) ;
#17179=DIRECTION ( 'NONE',  ( -1.224646799147351235E-16, 1.000000000000000000, 0.000000000000000000 ) ) ;
#17180=CARTESIAN_POINT ( 'NONE',  ( 16.72075857324119141, 7.444561356925491147, 7.000000000000000000 ) ) ;
#17182=EDGE_CURVE ( 'NONE', #32385, #18932, #28976, .T. ) ;
#17183=FACE_OUTER_BOUND ( 'NONE', #9437, .T. ) ;
#17184=CARTESIAN_POINT ( 'NONE',  ( -14.86556419889030778, 20.43481210330130082, 10.59344459855562270 ) ) ;
#17186=CARTESIAN_POINT ( 'NONE',  ( -5.982165713378355676, 28.55918256678905820, 9.000000000000001776 ) ) ;
#17187=VERTEX_POINT ( 'NONE', #32645 ) ;
#17191=DIRECTION ( 'NONE',  ( -1.000000000000000000, 0.000000000000000000, 0.000000000000000000 ) ) ;
#17193=ORIENTED_EDGE ( 'NONE', *, *, #10144, .T. ) ;
#17197=DIRECTION ( 'NONE',  ( 0.000000000000000000, 0.000000000000000000, -1.000000000000000000 ) ) ;
#17203=ORIENTED_EDGE ( 'NONE', *, *, #40153, .T. ) ;
#17206=CARTESIAN_POINT ( 'NONE',  ( 0.5000000000000000000, 37.04625217320466390, 10.99999999999999645 ) ) ;
#17208=AXIS2_PLACEMENT_3D ( 'NONE', #6804, #37506, #37304 ) ;
#17209=EDGE_LOOP ( 'NONE', ( #155, #26559, #7918, #24622 ) ) ;
#17211=VECTOR ( 'NONE', #7665, 1000.000000000000000 ) ;
#17216=FACE_OUTER_BOUND ( 'NONE', #16010, .T. ) ;
#17219=ORIENTED_EDGE ( 'NONE', *, *, #18087, .T. ) ;
#17220=DIRECTION ( 'NONE',  ( -0.000000000000000000, -0.000000000000000000, -1.000000000000000000 ) ) ;
#17221=AXIS2_PLACEMENT_3D ( 'NONE', #3427, #19464, #34315 ) ;
#17222=DIRECTION ( 'NONE',  ( 1.000000000000000000, 0.000000000000000000, 0.000000000000000000 ) ) ;
#17225=CARTESIAN_POINT ( 'NONE',  ( -14.99497092072327220, 22.09096420981882503, 7.202682876670051471 ) ) ;
#17226=EDGE_CURVE ( 'NONE', #26836, #13142, #22472, .T. ) ;
#17228=CIRCLE ( 'NONE', #12021, 0.5000000000000000000 ) ;
#17229=DIRECTION ( 'NONE',  ( -0.000000000000000000, -0.000000000000000000, -1.000000000000000000 ) ) ;
#17231=DIRECTION ( 'NONE',  ( -0.000000000000000000, 1.000000000000000000, -0.000000000000000000 ) ) ;
#17232=DIRECTION ( 'NONE',  ( 0.000000000000000000, 0.000000000000000000, 1.000000000000000000 ) ) ;
#17235=VECTOR ( 'NONE', #18619, 1000.000000000000000 ) ;
#17236=ORIENTED_EDGE ( 'NONE', *, *, #34105, .F. ) ;
#17238=CIRCLE ( 'NONE', #34102, 0.5000000000000013323 ) ;
#17239=FACE_OUTER_BOUND ( 'NONE', #19428, .T. ) ;
#17241=CARTESIAN_POINT ( 'NONE',  ( 9.427394655428274817, 11.06314620770945290, 7.500000000000000888 ) ) ;
#17243=EDGE_CURVE ( 'NONE', #2054, #18869, #38794, .T. ) ;
#17244=DIRECTION ( 'NONE',  ( -0.4067366430757888840, 0.9135454576426059736, 0.000000000000000000 ) ) ;
#17252=CARTESIAN_POINT ( 'NONE',  ( -1.693998953219646442, 12.12549434688617822, 10.00000000000000000 ) ) ;
#17255=ORIENTED_EDGE ( 'NONE', *, *, #996, .F. ) ;
#17259=EDGE_CURVE ( 'NONE', #12080, #39537, #4800, .T. ) ;
#17260=DIRECTION ( 'NONE',  ( -0.000000000000000000, -0.000000000000000000, -1.000000000000000000 ) ) ;
#17262=ORIENTED_EDGE ( 'NONE', *, *, #21542, .T. ) ;
#17267=AXIS2_PLACEMENT_3D ( 'NONE', #20622, #2723, #5368 ) ;
#17268=VECTOR ( 'NONE', #20737, 1000.000000000000114 ) ;
#17274=DIRECTION ( 'NONE',  ( 0.000000000000000000, 0.000000000000000000, -1.000000000000000000 ) ) ;
#17277=CARTESIAN_POINT ( 'NONE',  ( 12.99377146717206344, 26.19620116591418224, 10.00000000000000000 ) ) ;
#17278=ORIENTED_EDGE ( 'NONE', *, *, #16213, .T. ) ;
#17280=DIRECTION ( 'NONE',  ( 0.6724985119639563802, -0.2185080122244180134, 0.7071067811865461294 ) ) ;
#17281=FACE_OUTER_BOUND ( 'NONE', #13090, .T. ) ;
#17282=CARTESIAN_POINT ( 'NONE',  ( 14.06524961900336734, 27.71236540882597410, 7.000000000000000000 ) ) ;
#17287=CARTESIAN_POINT ( 'NONE',  ( 12.30736835487432757, 14.81698729810772441, 11.00000000000000000 ) ) ;
#17290=DIRECTION ( 'NONE',  ( -0.000000000000000000, -0.000000000000000000, -1.000000000000000000 ) ) ;
#17292=FACE_OUTER_BOUND ( 'NONE', #16987, .T. ) ;
#17298=DIRECTION ( 'NONE',  ( -1.000000000000000000, 0.000000000000000000, 0.000000000000000000 ) ) ;
#17300=ORIENTED_EDGE ( 'NONE', *, *, #37180, .T. ) ;
#17302=CARTESIAN_POINT ( 'NONE',  ( -13.05736835487441994, 16.11602540378456183, 10.49999999999999822 ) ) ;
#17303=CARTESIAN_POINT ( 'NONE',  ( 1.000000000000000666, 33.00000000000000000, 10.50000000000000000 ) ) ;
#17305=CARTESIAN_POINT ( 'NONE',  ( -9.665073660138979506, 25.11464168560200605, 10.49999999999999112 ) ) ;
#17306=EDGE_LOOP ( 'NONE', ( #37110, #30445, #22213 ) ) ;
#17310=DIRECTION ( 'NONE',  ( 0.5720614028176818078, -0.4156269377774653440, -0.7071067811865424657 ) ) ;
#17311=ORIENTED_EDGE ( 'NONE', *, *, #12543, .T. ) ;
#17313=CARTESIAN_POINT ( 'NONE',  ( -9.160254037844421049, 18.36602540378452630, 10.49999999999999822 ) ) ;
#17318=ORIENTED_EDGE ( 'NONE', *, *, #30794, .F. ) ;
#17321=DIRECTION ( 'NONE',  ( 0.6691306063588671194, 0.7431448254773861395, 0.000000000000000000 ) ) ;
#17324=AXIS2_PLACEMENT_3D ( 'NONE', #11647, #33394, #10839 ) ;
#17326=ORIENTED_EDGE ( 'NONE', *, *, #24297, .T. ) ;
#17328=EDGE_CURVE ( 'NONE', #38307, #38835, #17411, .T. ) ;
#17335=CARTESIAN_POINT ( 'NONE',  ( 2.525645716490518389, 8.212903943950921715, 9.500000000000000000 ) ) ;
#17336=CARTESIAN_POINT ( 'NONE',  ( 2.444768620639813594, 7.712926687590050179, 10.49999999999999822 ) ) ;
#17339=ORIENTED_EDGE ( 'NONE', *, *, #14981, .T. ) ;
#17341=EDGE_CURVE ( 'NONE', #12427, #1970, #8289, .T. ) ;
#17343=DIRECTION ( 'NONE',  ( 0.000000000000000000, 0.000000000000000000, 1.000000000000000000 ) ) ;
#17347=ORIENTED_EDGE ( 'NONE', *, *, #17852, .T. ) ;
#17349=LINE ( 'NONE', #35626, #36768 ) ;
#17352=CONICAL_SURFACE ( 'NONE', #14761, 1.000000000000005995, 0.7853981633974537191 ) ;
#17353=VECTOR ( 'NONE', #37326, 1000.000000000000000 ) ;
#17354=ORIENTED_EDGE ( 'NONE', *, *, #9753, .F. ) ;
#17357=DIRECTION ( 'NONE',  ( 1.000000000000000000, 0.000000000000000000, 0.000000000000000000 ) ) ;
#17359=ORIENTED_EDGE ( 'NONE', *, *, #38303, .T. ) ;
#17361=FACE_OUTER_BOUND ( 'NONE', #30117, .T. ) ;
#17364=ORIENTED_EDGE ( 'NONE', *, *, #38848, .T. ) ;
#17365=EDGE_CURVE ( 'NONE', #16528, #1872, #19975, .T. ) ;
#17367=EDGE_CURVE ( 'NONE', #8916, #29799, #32954, .T. ) ;
#17369=CIRCLE ( 'NONE', #14766, 6.000000000000000888 ) ;
#17375=DIRECTION ( 'NONE',  ( -0.9510565162951507556, 0.3090169943749560000, 0.000000000000000000 ) ) ;
#17379=DIRECTION ( 'NONE',  ( -0.6691306063588671194, -0.7431448254773861395, 0.000000000000000000 ) ) ;
#17380=DIRECTION ( 'NONE',  ( 0.000000000000000000, 0.000000000000000000, 1.000000000000000000 ) ) ;
#17381=EDGE_CURVE ( 'NONE', #4180, #29868, #6953, .T. ) ;
#17383=ORIENTED_EDGE ( 'NONE', *, *, #13517, .F. ) ;
#17385=DIRECTION ( 'NONE',  ( -0.000000000000000000, -0.000000000000000000, -1.000000000000000000 ) ) ;
#17386=DIRECTION ( 'NONE',  ( -0.000000000000000000, -0.000000000000000000, -1.000000000000000000 ) ) ;
#17390=CARTESIAN_POINT ( 'NONE',  ( -14.55889214498793471, 20.02072497456995137, 10.49999999999999822 ) ) ;
#17392=AXIS2_PLACEMENT_3D ( 'NONE', #8248, #20654, #5205 ) ;
#17395=CARTESIAN_POINT ( 'NONE',  ( -0.5000000000000003331, 36.50000000000000711, 9.500000000000000000 ) ) ;
#17397=LINE ( 'NONE', #20637, #11396 ) ;
#17399=ORIENTED_EDGE ( 'NONE', *, *, #2043, .F. ) ;
#17401=EDGE_LOOP ( 'NONE', ( #9869, #25721, #39592, #24778, #9187 ) ) ;
#17411=LINE ( 'NONE', #21239, #19297 ) ;
#17412=LINE ( 'NONE', #17815, #24461 ) ;
#17414=ORIENTED_EDGE ( 'NONE', *, *, #22684, .T. ) ;
#17416=AXIS2_PLACEMENT_3D ( 'NONE', #800, #16042, #34533 ) ;
#17417=AXIS2_PLACEMENT_3D ( 'NONE', #17764, #30139, #36636 ) ;
#17423=CARTESIAN_POINT ( 'NONE',  ( 4.096822963000107620, 8.035697679810645866, 7.000000000000000000 ) ) ;
#17424=CARTESIAN_POINT ( 'NONE',  ( 6.651296319737278750, 27.81603774131160023, 9.000000000000001776 ) ) ;
#17427=CARTESIAN_POINT ( 'NONE',  ( 14.99905852611806267, 22.33194247983193392, 7.000000000000000000 ) ) ;
#17428=CARTESIAN_POINT ( 'NONE',  ( 6.557822374958319323, 35.99981354310111215, 10.49999999999999822 ) ) ;
#17429=CARTESIAN_POINT ( 'NONE',  ( -9.160254037844421049, 18.36602540378452630, 10.49999999999999822 ) ) ;
#17432=DIRECTION ( 'NONE',  ( 0.5877852522924791323, 0.8090169943749430104, 0.000000000000000000 ) ) ;
#17435=DIRECTION ( 'NONE',  ( 0.6459741880212536147, -0.2876062384759530688, -0.7071067811865442421 ) ) ;
#17436=VECTOR ( 'NONE', #23740, 1000.000000000000114 ) ;
#17439=VECTOR ( 'NONE', #26834, 1000.000000000000114 ) ;
#17440=VERTEX_POINT ( 'NONE', #20853 ) ;
#17442=CARTESIAN_POINT ( 'NONE',  ( -14.81329996725647469, 19.93755115561707569, 10.50000000000000000 ) ) ;
#17443=CARTESIAN_POINT ( 'NONE',  ( -0.9438746746332824511, 37.23829181892411810, 10.49999999999999822 ) ) ;
#17445=LINE ( 'NONE', #29818, #970 ) ;
#17455=FACE_OUTER_BOUND ( 'NONE', #38430, .T. ) ;
#17456=ORIENTED_EDGE ( 'NONE', *, *, #12269, .T. ) ;
#17459=DIRECTION ( 'NONE',  ( -0.3090169943749573878, -0.9510565162951503115, 0.000000000000000000 ) ) ;
#17462=ADVANCED_FACE ( 'NONE', ( #11899 ), #24288, .T. ) ;
#17469=CIRCLE ( 'NONE', #37577, 1.000000000000002665 ) ;
#17471=ORIENTED_EDGE ( 'NONE', *, *, #789, .T. ) ;
#17472=CARTESIAN_POINT ( 'NONE',  ( -0.4999999999999998890, 37.26099332938164110, 10.94611345180490503 ) ) ;
#17474=EDGE_CURVE ( 'NONE', #28046, #18302, #8041, .T. ) ;
#17475=AXIS2_PLACEMENT_3D ( 'NONE', #8160, #39239, #24400 ) ;
#17476=DIRECTION ( 'NONE',  ( 0.000000000000000000, 0.000000000000000000, 1.000000000000000000 ) ) ;
#17478=DIRECTION ( 'NONE',  ( 1.000000000000000000, 0.000000000000000000, 0.000000000000000000 ) ) ;
#17480=CARTESIAN_POINT ( 'NONE',  ( -9.201548168576545450, 26.54122646004472585, 10.50000000000000533 ) ) ;
#17481=DIRECTION ( 'NONE',  ( 1.000000000000000000, 3.469446951953587368E-15, 0.000000000000000000 ) ) ;
#17482=FACE_OUTER_BOUND ( 'NONE', #9515, .T. ) ;
#17487=CARTESIAN_POINT ( 'NONE',  ( -9.303655249773276736, 10.73386218874833631, 7.500000000000000888 ) ) ;
#17488=ADVANCED_FACE ( 'NONE', ( #32848 ), #5000, .T. ) ;
#17492=B_SPLINE_CURVE_WITH_KNOTS ( 'NONE', 3,
 ( #23752, #33516, #36948, #30050 ),
 .UNSPECIFIED., .F., .F.,
 ( 4, 4 ),
 ( 0.9333335856709981115, 1.000000000000000000 ),
 .UNSPECIFIED. ) ;
#17495=AXIS2_PLACEMENT_3D ( 'NONE', #36265, #36854, #17978 ) ;
#17498=CARTESIAN_POINT ( 'NONE',  ( -13.28503138821885798, 15.53523575316151017, 7.000000000000000000 ) ) ;
#17499=EDGE_LOOP ( 'NONE', ( #4990, #22601, #11847, #33122 ) ) ;
#17500=EDGE_LOOP ( 'NONE', ( #16608, #36785, #38473, #24579 ) ) ;
#17503=DIRECTION ( 'NONE',  ( 0.9945218953682730678, -0.1045284632676569680, 0.000000000000000000 ) ) ;
#17507=ORIENTED_EDGE ( 'NONE', *, *, #8812, .F. ) ;
#17509=CARTESIAN_POINT ( 'NONE',  ( -3.503793317224517700, 8.420815634768727520, 11.00000000000000000 ) ) ;
#17510=CARTESIAN_POINT ( 'NONE',  ( -12.82065967939308493, 40.99677499958261961, 11.00000000000000000 ) ) ;
#17514=EDGE_CURVE ( 'NONE', #22657, #34540, #5401, .T. ) ;
#17515=DIRECTION ( 'NONE',  ( 1.000000000000000000, 0.000000000000000000, 0.000000000000000000 ) ) ;
#17522=CARTESIAN_POINT ( 'NONE',  ( -22.37798348102460722, 33.25980436007204588, 7.499999999999993783 ) ) ;
#17524=AXIS2_PLACEMENT_3D ( 'NONE', #38806, #30066, #14629 ) ;
#17525=CARTESIAN_POINT ( 'NONE',  ( 0.000000000000000000, 22.50000000000000355, 7.000000000000000000 ) ) ;
#17526=ORIENTED_EDGE ( 'NONE', *, *, #1172, .F. ) ;
#17528=LINE ( 'NONE', #20572, #38986 ) ;
#17529=VECTOR ( 'NONE', #9719, 1000.000000000000000 ) ;
#17531=DIRECTION ( 'NONE',  ( -0.9781476007338069101, -0.2079116908177532641, 0.000000000000000000 ) ) ;
#17535=FACE_OUTER_BOUND ( 'NONE', #27228, .T. ) ;
#17536=CARTESIAN_POINT ( 'NONE',  ( -13.10100158616367061, 15.51348347676449357, 10.87262190630137226 ) ) ;
#17538=ORIENTED_EDGE ( 'NONE', *, *, #37427, .F. ) ;
#17540=ORIENTED_EDGE ( 'NONE', *, *, #1108, .T. ) ;
#17543=CARTESIAN_POINT ( 'NONE',  ( -13.98881638187866550, 26.51951085733906410, 10.99999999999999289 ) ) ;
#17547=EDGE_LOOP ( 'NONE', ( #10956, #26398, #6449 ) ) ;
#17556=LINE ( 'NONE', #26883, #37174 ) ;
#17559=CARTESIAN_POINT ( 'NONE',  ( 13.30736835487433289, 15.68301270189216545, 11.00000000000000000 ) ) ;
#17561=VECTOR ( 'NONE', #28739, 1000.000000000000000 ) ;
#17562=ORIENTED_EDGE ( 'NONE', *, *, #4376, .F. ) ;
#17564=EDGE_CURVE ( 'NONE', #5349, #29941, #8651, .T. ) ;
#17566=EDGE_CURVE ( 'NONE', #15223, #4851, #31627, .T. ) ;
#17569=EDGE_CURVE ( 'NONE', #7663, #11410, #14105, .T. ) ;
#17574=ADVANCED_FACE ( 'NONE', ( #34234 ), #31377, .T. ) ;
#17576=AXIS2_PLACEMENT_3D ( 'NONE', #19652, #4418, #13757 ) ;
#17577=CARTESIAN_POINT ( 'NONE',  ( -1.854038262753995303, 7.614540224935766766, 7.102637441331452806 ) ) ;
#17578=CARTESIAN_POINT ( 'NONE',  ( -0.4999999999999998890, 37.00000000000000711, 7.500000000000000888 ) ) ;
#17580=VERTEX_POINT ( 'NONE', #12884 ) ;
#17582=LINE ( 'NONE', #29954, #824 ) ;
#17585=ADVANCED_FACE ( 'NONE', ( #18793 ), #34247, .T. ) ;
#17586=VECTOR ( 'NONE', #2627, 1000.000000000000000 ) ;
#17588=DIRECTION ( 'NONE',  ( 1.000000000000000000, 0.000000000000000000, 0.000000000000000000 ) ) ;
#17590=EDGE_CURVE ( 'NONE', #27094, #6329, #18672, .T. ) ;
#17593=VERTEX_POINT ( 'NONE', #37673 ) ;
#17598=ORIENTED_EDGE ( 'NONE', *, *, #20812, .F. ) ;
#17599=CARTESIAN_POINT ( 'NONE',  ( -14.57109471128386602, 21.97402451295043591, 10.49999999999999822 ) ) ;
#17600=VERTEX_POINT ( 'NONE', #5989 ) ;
#17610=VERTEX_POINT ( 'NONE', #504 ) ;
#17612=VECTOR ( 'NONE', #3704, 1000.000000000000000 ) ;
#17613=CARTESIAN_POINT ( 'NONE',  ( -1.693998953219646664, 12.12549434688617644, 10.50000000000000000 ) ) ;
#17614=CARTESIAN_POINT ( 'NONE',  ( -3.295881626406751419, 9.398963235502531433, 10.00000000000000000 ) ) ;
#17615=CARTESIAN_POINT ( 'NONE',  ( -14.31603901957233660, 19.98981538725089990, 7.500000000000004441 ) ) ;
#17618=EDGE_CURVE ( 'NONE', #14728, #24748, #9593, .T. ) ;
#17624=LINE ( 'NONE', #20255, #7670 ) ;
#17625=VECTOR ( 'NONE', #3418, 1000.000000000000000 ) ;
#17626=DIRECTION ( 'NONE',  ( -0.000000000000000000, -0.000000000000000000, -1.000000000000000000 ) ) ;
#17627=EDGE_CURVE ( 'NONE', #4137, #24512, #11543, .T. ) ;
#17635=CARTESIAN_POINT ( 'NONE',  ( -7.133890061153694617, 30.26901619224549833, 11.00000000000000000 ) ) ;
#17637=FACE_OUTER_BOUND ( 'NONE', #14072, .T. ) ;
#17638=DIRECTION ( 'NONE',  ( 1.000000000000000000, 0.000000000000000000, 0.000000000000000000 ) ) ;
#17639=CARTESIAN_POINT ( 'NONE',  ( -0.5000000000000005551, 33.00000000000000000, 10.50000000000000000 ) ) ;
#17641=EDGE_CURVE ( 'NONE', #34341, #31582, #3543, .T. ) ;
#17643=DIRECTION ( 'NONE',  ( 0.000000000000000000, 0.000000000000000000, 1.000000000000000000 ) ) ;
#17644=ORIENTED_EDGE ( 'NONE', *, *, #17772, .T. ) ;
#17646=CARTESIAN_POINT ( 'NONE',  ( 9.441034666242805073, 32.57396620494213124, 7.000000000000000000 ) ) ;
#17647=CARTESIAN_POINT ( 'NONE',  ( -13.90768907780708474, 27.88359266870287456, 10.49999999999999822 ) ) ;
#17650=CARTESIAN_POINT ( 'NONE',  ( -14.11133924723978161, 27.61078317377194224, 10.49999999999999822 ) ) ;
#17663=CARTESIAN_POINT ( 'NONE',  ( -3.992867117591420545, 8.524771480177605554, 10.50000000000000533 ) ) ;
#17666=PLANE ( 'NONE',  #14092 ) ;
#17673=AXIS2_PLACEMENT_3D ( 'NONE', #14191, #33098, #16854 ) ;
#17674=CARTESIAN_POINT ( 'NONE',  ( 8.339609403135803234, 11.87216320208440123, 10.50000000000000000 ) ) ;
#17676=CYLINDRICAL_SURFACE ( 'NONE', #35934, 6.000000000000002665 ) ;
#17677=CARTESIAN_POINT ( 'NONE',  ( 6.354454053420413473, 35.54304081427980577, 11.00000000000000000 ) ) ;
#17678=CIRCLE ( 'NONE', #8579, 0.5000000000000015543 ) ;
#17679=LINE ( 'NONE', #23957, #16206 ) ;
#17683=CARTESIAN_POINT ( 'NONE',  ( -2.568190708544567435, 12.82247983807085490, 10.50000000000001066 ) ) ;
#17687=ORIENTED_EDGE ( 'NONE', *, *, #32474, .F. ) ;
#17689=CYLINDRICAL_SURFACE ( 'NONE', #2802, 0.4999999999999995559 ) ;
#17691=CARTESIAN_POINT ( 'NONE',  ( -2.143544478356564031, 7.864861742947466539, 10.49999999999999822 ) ) ;
#17698=AXIS2_PLACEMENT_3D ( 'NONE', #2350, #35871, #36278 ) ;
#17699=DIRECTION ( 'NONE',  ( -0.4731467892558186561, 0.5254827454987605062, -0.7071067811865437980 ) ) ;
#17700=ADVANCED_FACE ( 'NONE', ( #9843 ), #37490, .T. ) ;
#17701=ORIENTED_EDGE ( 'NONE', *, *, #2542, .F. ) ;
#17702=ORIENTED_EDGE ( 'NONE', *, *, #5399, .T. ) ;
#17704=DIRECTION ( 'NONE',  ( 0.000000000000000000, -0.000000000000000000, 1.000000000000000000 ) ) ;
#17705=CARTESIAN_POINT ( 'NONE',  ( -12.41469063302772113, 14.32475803611781728, 10.49999999999999822 ) ) ;
#17707=CARTESIAN_POINT ( 'NONE',  ( -10.16122020288868733, 33.53402030034415304, 7.000000000000000000 ) ) ;
#17708=ORIENTED_EDGE ( 'NONE', *, *, #33705, .T. ) ;
#17710=CARTESIAN_POINT ( 'NONE',  ( 6.980762143445867984, 14.59310681135549537, 10.49999999999999645 ) ) ;
#17712=B_SPLINE_CURVE_WITH_KNOTS ( 'NONE', 3,
 ( #6872, #36624, #8796, #21183, #30535, #12035 ),
 .UNSPECIFIED., .F., .F.,
 ( 4, 2, 4 ),
 ( 0.000000000000000000, 0.5000000000000000000, 1.000000000000000000 ),
 .UNSPECIFIED. ) ;
#17713=ORIENTED_EDGE ( 'NONE', *, *, #29605, .T. ) ;
#17715=DIRECTION ( 'NONE',  ( -0.7886751345948098679, -0.2113248654051767539, 0.5773502691896337247 ) ) ;
#17719=VERTEX_POINT ( 'NONE', #37477 ) ;
#17721=ADVANCED_FACE ( 'NONE', ( #6581 ), #22220, .T. ) ;
#17723=CARTESIAN_POINT ( 'NONE',  ( 13.87104230352200140, 20.53934056656866147, 9.500000000000000000 ) ) ;
#17725=TOROIDAL_SURFACE ( 'NONE', #190, 1.000000000000000000, 0.5000000000000000000 ) ;
#17727=ORIENTED_EDGE ( 'NONE', *, *, #15015, .T. ) ;
#17730=FACE_OUTER_BOUND ( 'NONE', #8728, .T. ) ;
#17737=DIRECTION ( 'NONE',  ( -1.000000000000000000, 0.000000000000000000, 0.000000000000000000 ) ) ;
#17738=CARTESIAN_POINT ( 'NONE',  ( 23.80624316739448787, 27.22568555153026537, 7.500000000000000000 ) ) ;
#17740=EDGE_LOOP ( 'NONE', ( #34095, #16547, #8920, #29485 ) ) ;
#17741=VECTOR ( 'NONE', #25898, 1000.000000000000114 ) ;
#17746=ADVANCED_FACE ( 'NONE', ( #13484 ), #16109, .T. ) ;
#17747=CARTESIAN_POINT ( 'NONE',  ( 3.859984908523940828, 8.004988684046397296, 7.455686640544892718 ) ) ;
#17749=EDGE_CURVE ( 'NONE', #6055, #19050, #35224, .T. ) ;
#17750=ORIENTED_EDGE ( 'NONE', *, *, #10443, .F. ) ;
#17754=VECTOR ( 'NONE', #8417, 1000.000000000000000 ) ;
#17756=LINE ( 'NONE', #26878, #39925 ) ;
#17757=COLOUR_RGB ( '', 0.09019608, 0.27058824, 0.51372549) ;
#17758=ORIENTED_EDGE ( 'NONE', *, *, #11180, .F. ) ;
#17761=CARTESIAN_POINT ( 'NONE',  ( -14.36830325120615903, 20.48707633493503621, 7.000000000000000000 ) ) ;
#17762=ORIENTED_EDGE ( 'NONE', *, *, #23922, .F. ) ;
#17764=CARTESIAN_POINT ( 'NONE',  ( 1.590043107810628298, 12.61456814725305442, 10.49999999999999467 ) ) ;
#17772=EDGE_CURVE ( 'NONE', #2261, #26597, #36847, .T. ) ;
#17773=ORIENTED_EDGE ( 'NONE', *, *, #4565, .F. ) ;
#17776=CARTESIAN_POINT ( 'NONE',  ( -10.52298572764586915, 33.18979484031245875, 7.381627713044575323 ) ) ;
#17777=CARTESIAN_POINT ( 'NONE',  ( 14.79657804239838192, 20.03703012860012223, 7.381627713044574435 ) ) ;
#17780=FACE_OUTER_BOUND ( 'NONE', #11842, .T. ) ;
#17783=CARTESIAN_POINT ( 'NONE',  ( 13.49038105676655164, 15.86602540378438064, 10.50000000000000000 ) ) ;
#17786=DIRECTION ( 'NONE',  ( 1.000000000000000000, 0.000000000000000000, 0.000000000000000000 ) ) ;
#17789=CARTESIAN_POINT ( 'NONE',  ( 9.593266739736579396, 18.11602540378440196, 10.50000000000000178 ) ) ;
#17791=EDGE_CURVE ( 'NONE', #36670, #19499, #16951, .T. ) ;
#17794=ORIENTED_EDGE ( 'NONE', *, *, #5690, .T. ) ;
#17798=DIRECTION ( 'NONE',  ( 0.000000000000000000, 0.000000000000000000, -1.000000000000000000 ) ) ;
#17802=ORIENTED_EDGE ( 'NONE', *, *, #21542, .F. ) ;
#17808=CIRCLE ( 'NONE', #18456, 0.5000000000000004441 ) ;
#17810=DIRECTION ( 'NONE',  ( -0.7431448254773862505, 0.6691306063588671194, 0.000000000000000000 ) ) ;
#17814=CARTESIAN_POINT ( 'NONE',  ( 12.37435565298211237, 15.93301270189216545, 7.499999999999997335 ) ) ;
#17815=CARTESIAN_POINT ( 'NONE',  ( -9.221287281574667816, 10.65863771052209863, 11.00000000000000000 ) ) ;
#17816=CARTESIAN_POINT ( 'NONE',  ( -13.22516817658055288, 40.70288237343638826, 7.000000000000000000 ) ) ;
#17819=CIRCLE ( 'NONE', #3514, 0.5000000000000000000 ) ;
#17826=VERTEX_POINT ( 'NONE', #1505 ) ;
#17827=CARTESIAN_POINT ( 'NONE',  ( 10.47804177580207607, 33.28010392086025604, 7.000000000000000000 ) ) ;
#17828=CARTESIAN_POINT ( 'NONE',  ( -13.77067693704740492, 28.44713853003868564, 7.000000000000000000 ) ) ;
#17829=VERTEX_POINT ( 'NONE', #38678 ) ;
#17833=CARTESIAN_POINT ( 'NONE',  ( 3.813962023474617435, 32.29559562678520024, 10.00000000000000000 ) ) ;
#17834=LINE ( 'NONE', #32869, #27721 ) ;
#17840=CARTESIAN_POINT ( 'NONE',  ( -9.343266739736650450, 17.68301270189230578, 10.50000000000000000 ) ) ;
#17841=VERTEX_POINT ( 'NONE', #26283 ) ;
#17843=CARTESIAN_POINT ( 'NONE',  ( -5.034171952701849584, 35.03623199971308111, 10.50000000000000000 ) ) ;
#17844=DIRECTION ( 'NONE',  ( 0.7431448254773961315, 0.6691306063588561281, 0.000000000000000000 ) ) ;
#17847=DIRECTION ( 'NONE',  ( -0.000000000000000000, -0.000000000000000000, -1.000000000000000000 ) ) ;
#17849=AXIS2_PLACEMENT_3D ( 'NONE', #31802, #530, #22449 ) ;
#17850=CARTESIAN_POINT ( 'NONE',  ( 1.100969307443724343, 12.51061230184417816, 10.49999999999999467 ) ) ;
#17851=FACE_OUTER_BOUND ( 'NONE', #12241, .T. ) ;
#17852=EDGE_CURVE ( 'NONE', #13902, #26362, #35431, .T. ) ;
#17859=VERTEX_POINT ( 'NONE', #29334 ) ;
#17861=EDGE_LOOP ( 'NONE', ( #23275, #22200, #33137, #22018 ) ) ;
#17862=DIRECTION ( 'NONE',  ( -0.1470157664651945972, 0.6916548014802286204, -0.7071067811865454633 ) ) ;
#17863=CARTESIAN_POINT ( 'NONE',  ( -8.412270287199728358, 10.07085245822961994, 10.63089969389956835 ) ) ;
#17865=EDGE_CURVE ( 'NONE', #15951, #5508, #8123, .T. ) ;
#17869=ORIENTED_EDGE ( 'NONE', *, *, #32442, .T. ) ;
#17870=DIRECTION ( 'NONE',  ( 0.5254827454987551771, -0.4731467892558188226, -0.7071067811865476838 ) ) ;
#17873=LINE ( 'NONE', #23554, #35802 ) ;
#17874=AXIS2_PLACEMENT_3D ( 'NONE', #13756, #5021, #35708 ) ;
#17876=CARTESIAN_POINT ( 'NONE',  ( -3.607749162633401507, 7.931741834401821123, 10.49999999999999822 ) ) ;
#17878=DIRECTION ( 'NONE',  ( -0.1045284632676569680, -0.9945218953682729568, 0.000000000000000000 ) ) ;
#17879=DIRECTION ( 'NONE',  ( 0.8090169943749505599, 0.5877852522924689183, 0.000000000000000000 ) ) ;
#17880=DIRECTION ( 'NONE',  ( 0.9945218953682731788, -0.1045284632676563297, 0.000000000000000000 ) ) ;
#17887=CARTESIAN_POINT ( 'NONE',  ( 10.63499050845688920, 32.74860482968688302, 10.94611345180490503 ) ) ;
#17888=CARTESIAN_POINT ( 'NONE',  ( -14.83015932036200013, 20.24775513186575537, 7.485646746502382598 ) ) ;
#17889=ADVANCED_FACE ( 'NONE', ( #7184 ), #19582, .T. ) ;
#17892=CARTESIAN_POINT ( 'NONE',  ( -8.927394655428429360, 11.06314620770957013, 11.00000000000000000 ) ) ;
#17896=CYLINDRICAL_SURFACE ( 'NONE', #5582, 0.5000000000000004441 ) ;
#17897=ORIENTED_EDGE ( 'NONE', *, *, #21444, .T. ) ;
#17901=DIRECTION ( 'NONE',  ( 0.6691306063588670083, 0.7431448254773863615, 0.000000000000000000 ) ) ;
#17904=CARTESIAN_POINT ( 'NONE',  ( -8.981834765181659463, 10.98821582489678583, 10.99387789255783510 ) ) ;
#17908=CARTESIAN_POINT ( 'NONE',  ( -7.611215932167762155, 18.68301270189229513, 7.000000000000000000 ) ) ;
#17911=PLANE ( 'NONE',  #38444 ) ;
#17912=ORIENTED_EDGE ( 'NONE', *, *, #306, .F. ) ;
#17917=ADVANCED_FACE ( 'NONE', ( #16544 ), #28926, .F. ) ;
#17923=CARTESIAN_POINT ( 'NONE',  ( 10.59792294478272723, 33.06643021166726015, 10.49999999999999467 ) ) ;
#17924=CARTESIAN_POINT ( 'NONE',  ( 4.980911888400607168, 31.22871793335020030, 10.49999999999999822 ) ) ;
#17925=CONICAL_SURFACE ( 'NONE', #24404, 1.000000000000002665, 0.7853981633974469467 ) ;
#17926=AXIS2_PLACEMENT_3D ( 'NONE', #5829, #6020, #6221 ) ;
#17928=VECTOR ( 'NONE', #17086, 1000.000000000000000 ) ;
#17929=DIRECTION ( 'NONE',  ( -0.4731467892558353650, -0.5254827454987470725, 0.7071067811865425767 ) ) ;
#17931=AXIS2_PLACEMENT_3D ( 'NONE', #36763, #8933, #21324 ) ;
#17934=DIRECTION ( 'NONE',  ( -0.000000000000000000, -0.000000000000000000, -1.000000000000000000 ) ) ;
#17936=VERTEX_POINT ( 'NONE', #31778 ) ;
#17938=VERTEX_POINT ( 'NONE', #32183 ) ;
#17941=CARTESIAN_POINT ( 'NONE',  ( -3.585007771387415332, 8.038731668389095475, 10.82238861112328010 ) ) ;
#17945=ORIENTED_EDGE ( 'NONE', *, *, #33758, .F. ) ;
#17949=CARTESIAN_POINT ( 'NONE',  ( 6.576253646258392926, 14.29921418520925869, 10.50000000000000000 ) ) ;
#17950=ORIENTED_EDGE ( 'NONE', *, *, #20583, .F. ) ;
#17954=ORIENTED_EDGE ( 'NONE', *, *, #33510, .F. ) ;
#17957=CARTESIAN_POINT ( 'NONE',  ( 8.118377661053324701, 10.47536095541698486, 7.000000000000000000 ) ) ;
#17960=EDGE_LOOP ( 'NONE', ( #37926, #754, #22332 ) ) ;
#17963=AXIS2_PLACEMENT_3D ( 'NONE', #37468, #28515, #25663 ) ;
#17964=ADVANCED_FACE ( 'NONE', ( #22419 ), #3940, .F. ) ;
#17965=ORIENTED_EDGE ( 'NONE', *, *, #34596, .T. ) ;
#17969=DIRECTION ( 'NONE',  ( 1.000000000000000000, 0.000000000000000000, 0.000000000000000000 ) ) ;
#17971=LINE ( 'NONE', #24848, #35717 ) ;
#17972=EDGE_CURVE ( 'NONE', #14996, #15951, #7991, .T. ) ;
#17974=CARTESIAN_POINT ( 'NONE',  ( -5.464848148916058967, 36.46930998210962116, 7.485699520496980064 ) ) ;
#17975=ORIENTED_EDGE ( 'NONE', *, *, #40194, .T. ) ;
#17977=FACE_OUTER_BOUND ( 'NONE', #36262, .T. ) ;
#17978=DIRECTION ( 'NONE',  ( 0.5877852522924690293, -0.8090169943749503378, 0.000000000000000000 ) ) ;
#17986=AXIS2_PLACEMENT_3D ( 'NONE', #38666, #23827, #23231 ) ;
#17989=ADVANCED_FACE ( 'NONE', ( #17361 ), #16181, .T. ) ;
#17992=ORIENTED_EDGE ( 'NONE', *, *, #37930, .T. ) ;
#17993=CARTESIAN_POINT ( 'NONE',  ( -14.97009266215795087, 21.42933399866955213, 10.59344459855567422 ) ) ;
#17994=ORIENTED_EDGE ( 'NONE', *, *, #38640, .T. ) ;
#17996=CARTESIAN_POINT ( 'NONE',  ( 6.811226782241714517, 35.33967249274190436, 10.49999999999999822 ) ) ;
#17999=VECTOR ( 'NONE', #7002, 1000.000000000000000 ) ;
#18004=EDGE_LOOP ( 'NONE', ( #4079, #14218, #23638, #24276 ) ) ;
#18006=DIRECTION ( 'NONE',  ( 1.000000000000000000, 0.000000000000000000, 0.000000000000000000 ) ) ;
#18007=CARTESIAN_POINT ( 'NONE',  ( 8.118377661053324701, 10.47536095541698486, 7.500000000000000888 ) ) ;
#18008=LINE ( 'NONE', #36486, #12180 ) ;
#18009=ORIENTED_EDGE ( 'NONE', *, *, #28678, .F. ) ;
#18012=DIRECTION ( 'NONE',  ( -0.9135454576426005335, 0.4067366430758009299, -0.000000000000000000 ) ) ;
#18014=EDGE_CURVE ( 'NONE', #20455, #1674, #1831, .T. ) ;
#18017=VECTOR ( 'NONE', #38973, 1000.000000000000000 ) ;
#18018=VERTEX_POINT ( 'NONE', #39275 ) ;
#18019=DIRECTION ( 'NONE',  ( 0.6691306063588569053, -0.7431448254773954654, 0.000000000000000000 ) ) ;
#18020=CIRCLE ( 'NONE', #32958, 0.9999999999999985567 ) ;
#18025=FACE_OUTER_BOUND ( 'NONE', #26472, .T. ) ;
#18026=CARTESIAN_POINT ( 'NONE',  ( -8.339609403135948895, 11.87216320208451314, 7.000000000000000000 ) ) ;
#18027=LINE ( 'NONE', #30811, #2553 ) ;
#18028=CARTESIAN_POINT ( 'NONE',  ( -21.39877161664097827, 15.54711762656374141, 11.00000000000000000 ) ) ;
#18030=CARTESIAN_POINT ( 'NONE',  ( 14.44975846301061928, 26.39485539169812967, 10.49999999999999822 ) ) ;
#18032=CARTESIAN_POINT ( 'NONE',  ( 13.48130249190479191, 27.93180293473185927, 7.500000000000000888 ) ) ;
#18033=VERTEX_POINT ( 'NONE', #20604 ) ;
#18038=ADVANCED_FACE ( 'NONE', ( #5545 ), #544, .T. ) ;
#18042=DIRECTION ( 'NONE',  ( 0.2079116908177532919, -0.9781476007338070211, -0.000000000000000000 ) ) ;
#18043=LINE ( 'NONE', #29821, #8373 ) ;
#18044=CIRCLE ( 'NONE', #8288, 0.5000000000000004441 ) ;
#18045=AXIS2_PLACEMENT_3D ( 'NONE', #27535, #3346, #36879 ) ;
#18050=DIRECTION ( 'NONE',  ( 0.000000000000000000, 0.000000000000000000, 1.000000000000000000 ) ) ;
#18053=ORIENTED_EDGE ( 'NONE', *, *, #86, .T. ) ;
#18054=CIRCLE ( 'NONE', #14824, 6.000000000000012434 ) ;
#18058=DIRECTION ( 'NONE',  ( 1.000000000000000000, 0.000000000000000000, 0.000000000000000000 ) ) ;
#18063=ORIENTED_EDGE ( 'NONE', *, *, #10113, .T. ) ;
#18065=ORIENTED_EDGE ( 'NONE', *, *, #34244, .T. ) ;
#18066=LINE ( 'NONE', #20908, #37236 ) ;
#18068=CIRCLE ( 'NONE', #26499, 0.5000000000000004441 ) ;
#18071=FACE_OUTER_BOUND ( 'NONE', #32977, .T. ) ;
#18072=ORIENTED_EDGE ( 'NONE', *, *, #37560, .F. ) ;
#18073=CARTESIAN_POINT ( 'NONE',  ( -6.980762143445980783, 14.59310681135558063, 10.50000000000000000 ) ) ;
#18074=LINE ( 'NONE', #21114, #29938 ) ;
#18076=LINE ( 'NONE', #11771, #11112 ) ;
#18079=CIRCLE ( 'NONE', #32927, 0.5000000000000004441 ) ;
#18081=ORIENTED_EDGE ( 'NONE', *, *, #14101, .F. ) ;
#18087=EDGE_CURVE ( 'NONE', #15193, #27705, #27146, .T. ) ;
#18088=ADVANCED_FACE ( 'NONE', ( #32594 ), #5351, .T. ) ;
#18094=LINE ( 'NONE', #23977, #12707 ) ;
#18096=VERTEX_POINT ( 'NONE', #24832 ) ;
#18098=CARTESIAN_POINT ( 'NONE',  ( 0.8726219063013830324, 37.33905845025570613, 10.49999999999999822 ) ) ;
#18099=CARTESIAN_POINT ( 'NONE',  ( 10.06946225350410984, 32.23940090176269990, 7.000000000000000000 ) ) ;
#18100=AXIS2_PLACEMENT_3D ( 'NONE', #23698, #36097, #8051 ) ;
#18102=CARTESIAN_POINT ( 'NONE',  ( -9.221287281574706896, 10.65863771052213238, 10.59344459855561915 ) ) ;
#18103=ORIENTED_EDGE ( 'NONE', *, *, #30515, .T. ) ;
#18107=AXIS2_PLACEMENT_3D ( 'NONE', #31937, #13449, #38642 ) ;
#18108=ORIENTED_EDGE ( 'NONE', *, *, #38179, .F. ) ;
#18110=CARTESIAN_POINT ( 'NONE',  ( -9.393455880287618243, 11.27231877233277224, 10.49999999999999822 ) ) ;
#18111=EDGE_CURVE ( 'NONE', #15686, #37263, #30402, .T. ) ;
#18112=ORIENTED_EDGE ( 'NONE', *, *, #15601, .F. ) ;
#18115=EDGE_CURVE ( 'NONE', #25178, #17580, #23254, .T. ) ;
#18116=ORIENTED_EDGE ( 'NONE', *, *, #7539, .T. ) ;
#18118=DIRECTION ( 'NONE',  ( 1.000000000000000000, 0.000000000000000000, 0.000000000000000000 ) ) ;
#18119=FACE_OUTER_BOUND ( 'NONE', #16461, .T. ) ;
#18123=CARTESIAN_POINT ( 'NONE',  ( -10.14060191828654212, 25.26915018278947755, 10.50000000000000000 ) ) ;
#18125=AXIS2_PLACEMENT_3D ( 'NONE', #39364, #27373, #33493 ) ;
#18127=AXIS2_PLACEMENT_3D ( 'NONE', #24514, #6023, #27763 ) ;
#18128=CARTESIAN_POINT ( 'NONE',  ( -2.672146553953452575, 12.33340603770394139, 10.50000000000000000 ) ) ;
#18131=VECTOR ( 'NONE', #33366, 999.9999999999998863 ) ;
#18133=CARTESIAN_POINT ( 'NONE',  ( 10.32951289851633270, 32.69782367585502669, 10.83333333333333037 ) ) ;
#18134=VERTEX_POINT ( 'NONE', #24633 ) ;
#18136=VERTEX_POINT ( 'NONE', #24435 ) ;
#18144=ORIENTED_EDGE ( 'NONE', *, *, #38050, .F. ) ;
#18146=CARTESIAN_POINT ( 'NONE',  ( 8.247851828378060191, 9.985713325475870761, 10.49999999999999822 ) ) ;
#18149=ORIENTED_EDGE ( 'NONE', *, *, #38612, .F. ) ;
#18153=ORIENTED_EDGE ( 'NONE', *, *, #34014, .F. ) ;
#18155=DIRECTION ( 'NONE',  ( 1.000000000000000000, 0.000000000000000000, 0.000000000000000000 ) ) ;
#18157=ORIENTED_EDGE ( 'NONE', *, *, #4564, .F. ) ;
#18166=DIRECTION ( 'NONE',  ( 0.000000000000000000, 0.000000000000000000, -1.000000000000000000 ) ) ;
#18167=CARTESIAN_POINT ( 'NONE',  ( 4.984135866956514782, 36.15314577889351000, 10.49999999999999467 ) ) ;
#18169=DIRECTION ( 'NONE',  ( 0.2079116908177663092, 0.9781476007338041345, -0.000000000000000000 ) ) ;
#18171=DIRECTION ( 'NONE',  ( 1.000000000000000000, 0.000000000000000000, 0.000000000000000000 ) ) ;
#18172=ORIENTED_EDGE ( 'NONE', *, *, #29468, .T. ) ;
#18175=CARTESIAN_POINT ( 'NONE',  ( -11.11016527260153630, 31.83082137946488643, 7.000000000000000000 ) ) ;
#18177=DIRECTION ( 'NONE',  ( 0.4156269377774490792, -0.5720614028176843613, -0.7071067811865500152 ) ) ;
#18181=EDGE_LOOP ( 'NONE', ( #39029, #24549, #259, #15273 ) ) ;
#18184=EDGE_CURVE ( 'NONE', #3501, #31354, #5944, .T. ) ;
#18185=CARTESIAN_POINT ( 'NONE',  ( -3.057264508911468948, 12.92643568347973826, 10.50000000000000533 ) ) ;
#18188=PLANE ( 'NONE',  #31337 ) ;
#18189=AXIS2_PLACEMENT_3D ( 'NONE', #35043, #7198, #19597 ) ;
#18192=DIRECTION ( 'NONE',  ( -0.6724985119639631526, -0.2185080122244104639, -0.7071067811865420216 ) ) ;
#18194=LINE ( 'NONE', #30386, #4963 ) ;
#18197=FACE_OUTER_BOUND ( 'NONE', #34237, .T. ) ;
#18199=EDGE_CURVE ( 'NONE', #400, #36251, #3118, .T. ) ;
#18204=ADVANCED_FACE ( 'NONE', ( #27679 ), #28076, .T. ) ;
#18206=ORIENTED_EDGE ( 'NONE', *, *, #32442, .F. ) ;
#18212=DIRECTION ( 'NONE',  ( -0.4156269377774534091, 0.5720614028176876920, -0.7071067811865449082 ) ) ;
#18213=ADVANCED_FACE ( 'NONE', ( #15092 ), #18745, .F. ) ;
#18215=EDGE_CURVE ( 'NONE', #9209, #38623, #456, .T. ) ;
#18218=CARTESIAN_POINT ( 'NONE',  ( -4.188939243032555382, 44.61227686191953268, 11.00000000000000000 ) ) ;
#18219=CARTESIAN_POINT ( 'NONE',  ( 3.784955426773477072, 9.502919080911357952, 10.50000000000000000 ) ) ;
#18222=CYLINDRICAL_SURFACE ( 'NONE', #15612, 0.4999999999999997780 ) ;
#18223=CARTESIAN_POINT ( 'NONE',  ( -13.46929972531958697, 26.35070966310183138, 7.000000000000000000 ) ) ;
#18224=LINE ( 'NONE', #30812, #34857 ) ;
#18225=DIRECTION ( 'NONE',  ( -0.3090169943749572767, -0.9510565162951503115, 0.000000000000000000 ) ) ;
#18226=CARTESIAN_POINT ( 'NONE',  ( 4.940908595777813161, 35.94977745735560859, 7.000000000000000000 ) ) ;
#18229=EDGE_LOOP ( 'NONE', ( #25785, #25379, #16855, #7454 ) ) ;
#18231=DIRECTION ( 'NONE',  ( -0.5000000000000039968, -0.8660254037844363761, 0.000000000000000000 ) ) ;
#18233=CIRCLE ( 'NONE', #38320, 0.5000000000000024425 ) ;
#18239=DIRECTION ( 'NONE',  ( 0.000000000000000000, 0.000000000000000000, -1.000000000000000000 ) ) ;
#18240=ADVANCED_FACE ( 'NONE', ( #18346 ), #2901, .T. ) ;
#18241=CARTESIAN_POINT ( 'NONE',  ( 11.80736835487432046, 13.95096189432328693, 7.000000000000000000 ) ) ;
#18248=EDGE_CURVE ( 'NONE', #24077, #31037, #6354, .T. ) ;
#18251=ORIENTED_EDGE ( 'NONE', *, *, #23023, .F. ) ;
#18255=FACE_OUTER_BOUND ( 'NONE', #2069, .T. ) ;
#18259=AXIS2_PLACEMENT_3D ( 'NONE', #20164, #26652, #29502 ) ;
#18262=EDGE_CURVE ( 'NONE', #4778, #23735, #27482, .T. ) ;
#18263=DIRECTION ( 'NONE',  ( -0.5254827454987577307, -0.4731467892558122723, 0.7071067811865503483 ) ) ;
#18264=ORIENTED_EDGE ( 'NONE', *, *, #32604, .F. ) ;
#18266=FACE_OUTER_BOUND ( 'NONE', #25951, .T. ) ;
#18267=LINE ( 'NONE', #24353, #7893 ) ;
#18268=FACE_OUTER_BOUND ( 'NONE', #8227, .T. ) ;
#18271=CARTESIAN_POINT ( 'NONE',  ( -25.19768531712390569, 23.50223830518991619, 7.499999999999999112 ) ) ;
#18273=CARTESIAN_POINT ( 'NONE',  ( 2.525645716490518389, 8.212903943950921715, 7.000000000000000000 ) ) ;
#18277=ORIENTED_EDGE ( 'NONE', *, *, #25063, .T. ) ;
#18279=DIRECTION ( 'NONE',  ( -0.8660254037844363761, 0.5000000000000041078, -0.000000000000000000 ) ) ;
#18285=AXIS2_PLACEMENT_3D ( 'NONE', #11171, #22745, #1835 ) ;
#18288=VECTOR ( 'NONE', #24949, 1000.000000000000000 ) ;
#18290=ORIENTED_EDGE ( 'NONE', *, *, #6160, .F. ) ;
#18291=ORIENTED_EDGE ( 'NONE', *, *, #11747, .T. ) ;
#18293=EDGE_CURVE ( 'NONE', #26406, #5398, #31872, .T. ) ;
#18294=CARTESIAN_POINT ( 'NONE',  ( -9.343266739736652227, 17.68301270189230578, 10.50000000000000000 ) ) ;
#18295=CARTESIAN_POINT ( 'NONE',  ( -14.81329996725647469, 19.93755115561707569, 7.000000000000000000 ) ) ;
#18296=CARTESIAN_POINT ( 'NONE',  ( -8.927394655428429360, 11.06314620770957013, 10.99999999999999289 ) ) ;
#18300=CIRCLE ( 'NONE', #20248, 0.5000000000000002220 ) ;
#18301=DIRECTION ( 'NONE',  ( -0.000000000000000000, -0.000000000000000000, -1.000000000000000000 ) ) ;
#18302=VERTEX_POINT ( 'NONE', #6141 ) ;
#18304=CARTESIAN_POINT ( 'NONE',  ( 13.28503138821876917, 15.53523575316134142, 7.499999999999997335 ) ) ;
#18305=ORIENTED_EDGE ( 'NONE', *, *, #36219, .F. ) ;
#18311=EDGE_CURVE ( 'NONE', #29828, #22802, #18938, .T. ) ;
#18313=DIRECTION ( 'NONE',  ( 0.3090169943749573322, 0.9510565162951504226, 0.000000000000000000 ) ) ;
#18314=ORIENTED_EDGE ( 'NONE', *, *, #33963, .F. ) ;
#18315=CYLINDRICAL_SURFACE ( 'NONE', #6756, 0.5000000000000004441 ) ;
#18316=LINE ( 'NONE', #2874, #10449 ) ;
#18319=CARTESIAN_POINT ( 'NONE',  ( 3.888911272182352441, 9.013845280544455107, 9.500000000000000000 ) ) ;
#18320=VECTOR ( 'NONE', #32695, 1000.000000000000000 ) ;
#18322=FACE_OUTER_BOUND ( 'NONE', #15280, .T. ) ;
#18323=FACE_OUTER_BOUND ( 'NONE', #7569, .T. ) ;
#18325=ORIENTED_EDGE ( 'NONE', *, *, #4556, .F. ) ;
#18327=VECTOR ( 'NONE', #5795, 1000.000000000000000 ) ;
#18330=ADVANCED_FACE ( 'NONE', ( #39868 ), #28460, .T. ) ;
#18331=CARTESIAN_POINT ( 'NONE',  ( -3.699151772512148995, 7.951170058885317360, 10.49999999999999822 ) ) ;
#18337=ORIENTED_EDGE ( 'NONE', *, *, #22762, .F. ) ;
#18346=FACE_OUTER_BOUND ( 'NONE', #29190, .T. ) ;
#18347=DIRECTION ( 'NONE',  ( 0.1045284632676437703, -0.9945218953682745111, -0.000000000000000000 ) ) ;
#18348=ORIENTED_EDGE ( 'NONE', *, *, #10776, .F. ) ;
#18352=CARTESIAN_POINT ( 'NONE',  ( 3.503793317224329851, 8.420815634768676006, 7.000000000000000000 ) ) ;
#18354=ORIENTED_EDGE ( 'NONE', *, *, #12543, .F. ) ;
#18355=AXIS2_PLACEMENT_3D ( 'NONE', #2659, #15046, #27437 ) ;
#18358=CARTESIAN_POINT ( 'NONE',  ( -11.94134295108998245, 16.18301270189233065, 10.00000000000000000 ) ) ;
#18359=EDGE_CURVE ( 'NONE', #25420, #32345, #37819, .T. ) ;
#18360=FACE_OUTER_BOUND ( 'NONE', #16476, .T. ) ;
#18363=CIRCLE ( 'NONE', #32075, 0.9999999999999985567 ) ;
#18365=CONICAL_SURFACE ( 'NONE', #22233, 1.000000000000004441, 0.7853981633974524978 ) ;
#18369=DIRECTION ( 'NONE',  ( -0.6691306063588569053, 0.7431448254773954654, 0.000000000000000000 ) ) ;
#18372=CARTESIAN_POINT ( 'NONE',  ( 14.25384497784216009, 25.55416164399396806, 7.000000000000000000 ) ) ;
#18373=EDGE_CURVE ( 'NONE', #24416, #16847, #2525, .T. ) ;
#18376=VERTEX_POINT ( 'NONE', #25621 ) ;
#18381=LINE ( 'NONE', #27911, #27597 ) ;
#18383=VERTEX_POINT ( 'NONE', #38020 ) ;
#18384=LINE ( 'NONE', #30967, #30707 ) ;
#18385=EDGE_LOOP ( 'NONE', ( #18701, #39986, #30889, #15809 ) ) ;
#18387=CARTESIAN_POINT ( 'NONE',  ( 15.82937963299585071, 7.760892663579005202, 10.00000000000000000 ) ) ;
#18389=CARTESIAN_POINT ( 'NONE',  ( 9.189613563248487438, 10.70223284378001516, 10.76099332938164288 ) ) ;
#18390=AXIS2_PLACEMENT_3D ( 'NONE', #2135, #26912, #26310 ) ;
#18393=DIRECTION ( 'NONE',  ( -0.8090169943749430104, 0.5877852522924791323, 0.000000000000000000 ) ) ;
#18395=ORIENTED_EDGE ( 'NONE', *, *, #16849, .F. ) ;
#18398=LINE ( 'NONE', #27731, #4336 ) ;
#18399=LINE ( 'NONE', #30597, #36206 ) ;
#18402=CIRCLE ( 'NONE', #33964, 1.000000000000006883 ) ;
#18404=DIRECTION ( 'NONE',  ( -0.9135454576425986462, 0.4067366430758054263, 0.000000000000000000 ) ) ;
#18405=VECTOR ( 'NONE', #21847, 1000.000000000000000 ) ;
#18408=FACE_OUTER_BOUND ( 'NONE', #3251, .T. ) ;
#18411=EDGE_LOOP ( 'NONE', ( #4490, #34040, #1982, #7342 ) ) ;
#18412=EDGE_CURVE ( 'NONE', #23249, #4180, #4090, .T. ) ;
#18413=DIRECTION ( 'NONE',  ( -0.6691306063588570163, 0.7431448254773952433, 0.000000000000000000 ) ) ;
#18416=CARTESIAN_POINT ( 'NONE',  ( 13.94482798346721175, 26.50521816028912525, 11.00000000000000000 ) ) ;
#18418=DIRECTION ( 'NONE',  ( 0.5821182788257885932, 0.000000000000000000, -0.8131041196900317125 ) ) ;
#18419=CARTESIAN_POINT ( 'NONE',  ( 14.55573640795740076, 20.46737631633098431, 10.96580508970281542 ) ) ;
#18420=PLANE ( 'NONE',  #24584 ) ;
#18421=CARTESIAN_POINT ( 'NONE',  ( -12.19134295108997712, 16.61602540378455117, 10.00000000000000000 ) ) ;
#18422=CARTESIAN_POINT ( 'NONE',  ( 11.59687233693865593, 32.01413362675371133, 7.485699520496978288 ) ) ;
#18426=VERTEX_POINT ( 'NONE', #28878 ) ;
#18428=FACE_OUTER_BOUND ( 'NONE', #17306, .T. ) ;
#18429=AXIS2_PLACEMENT_3D ( 'NONE', #26506, #4567, #26703 ) ;
#18430=CARTESIAN_POINT ( 'NONE',  ( 13.24038105676659960, 15.43301270189224716, 10.59344459855565468 ) ) ;
#18435=B_SPLINE_SURFACE_WITH_KNOTS ( 'NONE', 1, 3, ( 
 ( #39558, #18430, #30821, #25501, #27961, #31806, #37309, #25311, #28161, #3772 ),
 ( #24915, #13310, #34658, #37901, #733, #16371, #3377, #3971, #19019, #15574 ) ),
 .UNSPECIFIED., .F., .F., .F.,
 ( 2, 2 ),
 ( 4, 2, 2, 2, 4 ),
 ( 0.000000000000000000, 1.000000000000000000 ),
 ( 1.183199640139713571, 1.575898721838439265, 1.968597803537164737, 2.361296885235890208, 2.753995966934615680 ),
 .UNSPECIFIED. ) ;
#18448=ORIENTED_EDGE ( 'NONE', *, *, #16104, .T. ) ;
#18452=CARTESIAN_POINT ( 'NONE',  ( 4.727507481117214638, 31.88885898370941874, 11.00000000000000000 ) ) ;
#18456=AXIS2_PLACEMENT_3D ( 'NONE', #3620, #21902, #16015 ) ;
#18458=ORIENTED_EDGE ( 'NONE', *, *, #10706, .T. ) ;
#18459=DIRECTION ( 'NONE',  ( 0.2079116908177663647, 0.9781476007338042455, 0.000000000000000000 ) ) ;
#18460=ORIENTED_EDGE ( 'NONE', *, *, #11360, .T. ) ;
#18461=PLANE ( 'NONE',  #10613 ) ;
#18464=CARTESIAN_POINT ( 'NONE',  ( -7.611215932167763043, 18.68301270189229513, 7.000000000000000000 ) ) ;
#18468=CARTESIAN_POINT ( 'NONE',  ( -5.494150297853999554, 36.06936027812446355, 11.00000000000000355 ) ) ;
#18469=PLANE ( 'NONE',  #10471 ) ;
#18470=EDGE_CURVE ( 'NONE', #10226, #11532, #25103, .T. ) ;
#18471=LINE ( 'NONE', #12167, #38356 ) ;
#18475=VECTOR ( 'NONE', #10457, 1000.000000000000000 ) ;
#18476=EDGE_LOOP ( 'NONE', ( #23017, #39677, #11351, #12623 ) ) ;
#18480=CARTESIAN_POINT ( 'NONE',  ( 10.44103466624280507, 32.57396620494213124, 11.00000000000000000 ) ) ;
#18485=EDGE_CURVE ( 'NONE', #14611, #15571, #3890, .T. ) ;
#18486=EDGE_CURVE ( 'NONE', #12690, #4300, #21340, .T. ) ;
#18487=DIRECTION ( 'NONE',  ( 0.000000000000000000, 0.000000000000000000, 1.000000000000000000 ) ) ;
#18488=ADVANCED_FACE ( 'NONE', ( #5300 ), #29881, .T. ) ;
#18489=VERTEX_POINT ( 'NONE', #11201 ) ;
#18491=CARTESIAN_POINT ( 'NONE',  ( 1.000000000000000444, 37.04625217320466390, 10.49999999999999822 ) ) ;
#18493=AXIS2_PLACEMENT_3D ( 'NONE', #16836, #23117, #35516 ) ;
#18494=CARTESIAN_POINT ( 'NONE',  ( 9.303655249773111535, 10.73386218874820663, 7.500000000000000888 ) ) ;
#18495=ORIENTED_EDGE ( 'NONE', *, *, #21059, .T. ) ;
#18498=DIRECTION ( 'NONE',  ( -0.1045284632676569819, -0.9945218953682730678, 0.000000000000000000 ) ) ;
#18499=VERTEX_POINT ( 'NONE', #7743 ) ;
#18500=AXIS2_PLACEMENT_3D ( 'NONE', #32624, #32419, #29356 ) ;
#18506=ORIENTED_EDGE ( 'NONE', *, *, #32339, .T. ) ;
#18512=LINE ( 'NONE', #22145, #21368 ) ;
#18513=ORIENTED_EDGE ( 'NONE', *, *, #3692, .T. ) ;
#18514=LINE ( 'NONE', #25203, #7311 ) ;
#18516=CARTESIAN_POINT ( 'NONE',  ( -6.854454053420242943, 35.54304081427989814, 7.500000000000000888 ) ) ;
#18517=CARTESIAN_POINT ( 'NONE',  ( -12.30736835487442704, 14.81698729810789672, 7.000000000000000000 ) ) ;
#18518=AXIS2_PLACEMENT_3D ( 'NONE', #2057, #14432, #2455 ) ;
#18524=CARTESIAN_POINT ( 'NONE',  ( 3.813962023474613439, 32.29559562678520024, 10.50000000000000000 ) ) ;
#18525=DIRECTION ( 'NONE',  ( -0.6691306063588670083, -0.7431448254773863615, 0.000000000000000000 ) ) ;
#18526=ORIENTED_EDGE ( 'NONE', *, *, #12404, .T. ) ;
#18528=AXIS2_PLACEMENT_3D ( 'NONE', #15839, #24979, #28224 ) ;
#18531=CARTESIAN_POINT ( 'NONE',  ( -4.006135375494391582, 8.432903524120151317, 10.49999999999999822 ) ) ;
#18532=EDGE_CURVE ( 'NONE', #28430, #6642, #11404, .T. ) ;
#18534=VERTEX_POINT ( 'NONE', #35988 ) ;
#18538=ADVANCED_FACE ( 'NONE', ( #14040 ), #8353, .T. ) ;
#18539=ORIENTED_EDGE ( 'NONE', *, *, #3467, .T. ) ;
#18546=CARTESIAN_POINT ( 'NONE',  ( -13.37378135583788286, 20.59160479820267398, 9.500000000000000000 ) ) ;
#18547=ORIENTED_EDGE ( 'NONE', *, *, #39557, .F. ) ;
#18549=ORIENTED_EDGE ( 'NONE', *, *, #27283, .T. ) ;
#18553=ORIENTED_EDGE ( 'NONE', *, *, #37229, .F. ) ;
#18555=VECTOR ( 'NONE', #7320, 1000.000000000000000 ) ;
#18556=CARTESIAN_POINT ( 'NONE',  ( -10.24926262130046695, 33.45294210977303351, 7.102474990965862212 ) ) ;
#18557=EDGE_CURVE ( 'NONE', #32632, #11714, #1659, .T. ) ;
#18558=LINE ( 'NONE', #3309, #21289 ) ;
#18559=VECTOR ( 'NONE', #10935, 1000.000000000000000 ) ;
#18560=CIRCLE ( 'NONE', #38007, 6.000000000000003553 ) ;
#18561=DIRECTION ( 'NONE',  ( -0.000000000000000000, -0.000000000000000000, -1.000000000000000000 ) ) ;
#18565=EDGE_CURVE ( 'NONE', #13010, #18932, #19351, .T. ) ;
#18572=LINE ( 'NONE', #280, #15088 ) ;
#18574=ORIENTED_EDGE ( 'NONE', *, *, #17182, .F. ) ;
#18577=LINE ( 'NONE', #3329, #36688 ) ;
#18580=DIRECTION ( 'NONE',  ( -0.5877852522924691403, 0.8090169943749505599, -0.000000000000000000 ) ) ;
#18581=ADVANCED_FACE ( 'NONE', ( #1865 ), #30086, .T. ) ;
#18582=EDGE_LOOP ( 'NONE', ( #32675, #19171, #4907, #18144, #10860 ) ) ;
#18583=AXIS2_PLACEMENT_3D ( 'NONE', #7731, #39213, #29671 ) ;
#18585=CARTESIAN_POINT ( 'NONE',  ( 24.21836086243564523, 15.77821876070162332, 9.500000000000000000 ) ) ;
#18586=ADVANCED_FACE ( 'NONE', ( #33147 ), #26633, .T. ) ;
#18590=CIRCLE ( 'NONE', #23771, 1.000000000000000444 ) ;
#18591=EDGE_LOOP ( 'NONE', ( #7465, #5549, #3354, #8386 ) ) ;
#18594=DIRECTION ( 'NONE',  ( 0.8090169943749426773, -0.5877852522924796874, 0.000000000000000000 ) ) ;
#18596=ORIENTED_EDGE ( 'NONE', *, *, #29980, .F. ) ;
#18598=VECTOR ( 'NONE', #28117, 999.9999999999998863 ) ;
#18600=CARTESIAN_POINT ( 'NONE',  ( 14.86556419889026515, 20.43481210330100595, 10.50000000000000000 ) ) ;
#18605=DIRECTION ( 'NONE',  ( 0.000000000000000000, 0.000000000000000000, -1.000000000000000000 ) ) ;
#18607=EDGE_LOOP ( 'NONE', ( #33178, #180, #39252, #16871 ) ) ;
#18609=ADVANCED_FACE ( 'NONE', ( #26431 ), #26230, .T. ) ;
#18610=CARTESIAN_POINT ( 'NONE',  ( -7.468455364333135726, 29.89744377950679777, 11.00000000000000000 ) ) ;
#18611=ADVANCED_FACE ( 'NONE', ( #5102 ), #4701, .F. ) ;
#18612=ORIENTED_EDGE ( 'NONE', *, *, #2643, .F. ) ;
#18613=DIRECTION ( 'NONE',  ( -0.000000000000000000, -0.000000000000000000, -1.000000000000000000 ) ) ;
#18615=VECTOR ( 'NONE', #4843, 1000.000000000000000 ) ;
#18616=DIRECTION ( 'NONE',  ( 0.9135454576426006446, -0.4067366430758009299, 0.000000000000000000 ) ) ;
#18617=CARTESIAN_POINT ( 'NONE',  ( -1.590043107810771073, 12.61456814725308995, 10.50000000000000000 ) ) ;
#18619=DIRECTION ( 'NONE',  ( -0.000000000000000000, -0.000000000000000000, 1.000000000000000000 ) ) ;
#18620=DIRECTION ( 'NONE',  ( -0.9135454576426004225, 0.4067366430758009854, 0.000000000000000000 ) ) ;
#18621=CARTESIAN_POINT ( 'NONE',  ( 13.30736835487433467, 16.54903810567660472, 7.000000000000000000 ) ) ;
#18622=DIRECTION ( 'NONE',  ( -0.7071067811865504593, 0.000000000000000000, -0.7071067811865445751 ) ) ;
#18623=CARTESIAN_POINT ( 'NONE',  ( 12.03571151536236528, 31.45218678977230908, 7.000000000000000000 ) ) ;
#18624=DIRECTION ( 'NONE',  ( 1.000000000000000000, 0.000000000000000000, 0.000000000000000000 ) ) ;
#18626=FACE_OUTER_BOUND ( 'NONE', #22167, .T. ) ;
#18629=CARTESIAN_POINT ( 'NONE',  ( 12.22403502154099542, 14.67264973081032053, 10.83333333333333037 ) ) ;
#18635=ORIENTED_EDGE ( 'NONE', *, *, #37534, .F. ) ;
#18643=DIRECTION ( 'NONE',  ( -0.000000000000000000, -0.000000000000000000, -1.000000000000000000 ) ) ;
#18647=AXIS2_PLACEMENT_3D ( 'NONE', #24882, #37277, #9451 ) ;
#18648=CIRCLE ( 'NONE', #483, 6.000000000000008882 ) ;
#18650=ORIENTED_EDGE ( 'NONE', *, *, #13036, .F. ) ;
#18651=DIRECTION ( 'NONE',  ( 1.000000000000000000, 0.000000000000000000, 0.000000000000000000 ) ) ;
#18653=AXIS2_PLACEMENT_3D ( 'NONE', #514, #15750, #3556 ) ;
#18657=ORIENTED_EDGE ( 'NONE', *, *, #16466, .F. ) ;
#18658=PLANE ( 'NONE',  #12205 ) ;
#18660=PLANE ( 'NONE',  #12578 ) ;
#18663=ORIENTED_EDGE ( 'NONE', *, *, #6931, .F. ) ;
#18665=CARTESIAN_POINT ( 'NONE',  ( -9.284827327736387304, 10.70480225629000870, 10.49999999999999645 ) ) ;
#18667=DIRECTION ( 'NONE',  ( 1.000000000000000000, 0.000000000000000000, 0.000000000000000000 ) ) ;
#18672=CIRCLE ( 'NONE', #38122, 6.000000000000000888 ) ;
#18678=AXIS2_PLACEMENT_3D ( 'NONE', #14155, #17626, #20259 ) ;
#18680=CARTESIAN_POINT ( 'NONE',  ( 5.198706521309295780, 29.65540566576566661, 9.000000000000001776 ) ) ;
#18685=EDGE_CURVE ( 'NONE', #24743, #23135, #32476, .T. ) ;
#18686=CARTESIAN_POINT ( 'NONE',  ( 5.644276917315719011, 36.40655018617690786, 10.49999999999999822 ) ) ;
#18687=ORIENTED_EDGE ( 'NONE', *, *, #1118, .T. ) ;
#18691=DIRECTION ( 'NONE',  ( -0.4067366430758009299, -0.9135454576426005335, 0.000000000000000000 ) ) ;
#18694=EDGE_CURVE ( 'NONE', #19098, #15240, #37954, .T. ) ;
#18696=DIRECTION ( 'NONE',  ( -1.000000000000000000, 0.000000000000000000, 0.000000000000000000 ) ) ;
#18697=EDGE_CURVE ( 'NONE', #32625, #29611, #35308, .T. ) ;
#18698=EDGE_LOOP ( 'NONE', ( #36622, #9234, #10520, #29643 ) ) ;
#18700=CARTESIAN_POINT ( 'NONE',  ( 4.591666147298500533, 15.32946292166668556, 7.000000000000000000 ) ) ;
#18701=ORIENTED_EDGE ( 'NONE', *, *, #33709, .T. ) ;
#18703=CIRCLE ( 'NONE', #27774, 0.5000000000000004441 ) ;
#18704=VECTOR ( 'NONE', #21982, 1000.000000000000000 ) ;
#18711=CIRCLE ( 'NONE', #1193, 1.000000000000013101 ) ;
#18713=ORIENTED_EDGE ( 'NONE', *, *, #22037, .F. ) ;
#18715=DIRECTION ( 'NONE',  ( -0.3090169943749589976, -0.9510565162951498674, 0.000000000000000000 ) ) ;
#18718=EDGE_CURVE ( 'NONE', #14858, #6691, #985, .T. ) ;
#18719=LINE ( 'NONE', #28051, #25333 ) ;
#18723=DIRECTION ( 'NONE',  ( -0.6691306063588570163, 0.7431448254773953543, -0.000000000000000000 ) ) ;
#18724=AXIS2_PLACEMENT_3D ( 'NONE', #18352, #9999, #31333 ) ;
#18725=EDGE_LOOP ( 'NONE', ( #13684, #37777, #27967, #33051 ) ) ;
#18730=CARTESIAN_POINT ( 'NONE',  ( 3.820972158148982167, 8.017991022712324778, 10.49999999999999467 ) ) ;
#18732=ORIENTED_EDGE ( 'NONE', *, *, #8830, .T. ) ;
#18736=EDGE_CURVE ( 'NONE', #2141, #39108, #14460, .T. ) ;
#18738=EDGE_LOOP ( 'NONE', ( #36432, #8403, #35776, #14928, #25570 ) ) ;
#18744=B_SPLINE_CURVE_WITH_KNOTS ( 'NONE', 3,
 ( #29445, #26395, #7098, #16457, #29043, #13400, #10161, #13601 ),
 .UNSPECIFIED., .F., .F.,
 ( 4, 2, 2, 4 ),
 ( 0.000000000000000000, 0.0002364868538934293248, 0.0004729737077868575112, 0.0009459474155737107939 ),
 .UNSPECIFIED. ) ;
#18745=CYLINDRICAL_SURFACE ( 'NONE', #9620, 6.000000000000008882 ) ;
#18746=LINE ( 'NONE', #12439, #34840 ) ;
#18755=CARTESIAN_POINT ( 'NONE',  ( -14.45538749008468038, 26.50521816028845734, 7.489440493383480835 ) ) ;
#18756=DIRECTION ( 'NONE',  ( -0.4999999999999920064, 0.8660254037844432595, 0.000000000000000000 ) ) ;
#18758=AXIS2_PLACEMENT_3D ( 'NONE', #17843, #36320, #35915 ) ;
#18759=FACE_OUTER_BOUND ( 'NONE', #2351, .T. ) ;
#18760=PLANE ( 'NONE',  #25982 ) ;
#18761=EDGE_CURVE ( 'NONE', #29912, #1935, #3157, .T. ) ;
#18762=B_SPLINE_SURFACE_WITH_KNOTS ( 'NONE', 1, 3, ( 
 ( #2848, #15236, #12188, #39813, #18098, #15035, #27427, #24581, #18491, #9142 ),
 ( #21527, #6086, #15436, #24775, #27827, #12385, #9345, #21725, #17206, #32441 ) ),
 .UNSPECIFIED., .F., .F., .F.,
 ( 2, 2 ),
 ( 4, 2, 2, 2, 4 ),
 ( 0.000000000000000000, 1.000000000000000000 ),
 ( 1.570796326794897002, 1.963495408493620920, 2.356194490192344837, 2.748893571891068976, 3.141592653589793116 ),
 .UNSPECIFIED. ) ;
#18766=CARTESIAN_POINT ( 'NONE',  ( 12.99377146717205633, 26.19620116591417869, 7.000000000000000000 ) ) ;
#18769=FACE_OUTER_BOUND ( 'NONE', #35511, .T. ) ;
#18771=ORIENTED_EDGE ( 'NONE', *, *, #6638, .F. ) ;
#18776=VERTEX_POINT ( 'NONE', #10126 ) ;
#18777=CARTESIAN_POINT ( 'NONE',  ( -20.33644687577595178, 12.50987689638972356, 7.000000000000000000 ) ) ;
#18778=VERTEX_POINT ( 'NONE', #16629 ) ;
#18780=DIRECTION ( 'NONE',  ( 0.5877852522924689183, -0.8090169943749505599, 0.000000000000000000 ) ) ;
#18784=AXIS2_PLACEMENT_3D ( 'NONE', #6408, #12907, #923 ) ;
#18788=LINE ( 'NONE', #10439, #39087 ) ;
#18790=VERTEX_POINT ( 'NONE', #31856 ) ;
#18793=FACE_OUTER_BOUND ( 'NONE', #38373, .T. ) ;
#18794=EDGE_CURVE ( 'NONE', #36223, #38699, #23918, .T. ) ;
#18795=CARTESIAN_POINT ( 'NONE',  ( 6.654030453887980201, 35.94335816374507431, 7.500000000000000888 ) ) ;
#18796=DIRECTION ( 'NONE',  ( 1.000000000000000000, -1.040834085586081417E-14, 0.000000000000000000 ) ) ;
#18797=AXIS2_PLACEMENT_3D ( 'NONE', #23150, #815, #7102 ) ;
#18798=ORIENTED_EDGE ( 'NONE', *, *, #38206, .T. ) ;
#18801=ADVANCED_FACE ( 'NONE', ( #16833 ), #4227, .F. ) ;
#18803=ORIENTED_EDGE ( 'NONE', *, *, #39347, .T. ) ;
#18805=DIRECTION ( 'NONE',  ( -0.7431448254773953543, -0.6691306063588570163, 0.000000000000000000 ) ) ;
#18808=ADVANCED_FACE ( 'NONE', ( #1588 ), #3824, .T. ) ;
#18810=VECTOR ( 'NONE', #25808, 1000.000000000000114 ) ;
#18811=CARTESIAN_POINT ( 'NONE',  ( 6.282361020112160688, 14.70372268239673197, 10.49999999999999822 ) ) ;
#18815=FACE_OUTER_BOUND ( 'NONE', #19636, .T. ) ;
#18817=CONICAL_SURFACE ( 'NONE', #12950, 0.5000000000000013323, 0.7853981633974529419 ) ;
#18818=CARTESIAN_POINT ( 'NONE',  ( 9.665073660139013256, 25.11464168560187460, 10.50000000000000711 ) ) ;
#18823=ORIENTED_EDGE ( 'NONE', *, *, #4478, .T. ) ;
#18825=LINE ( 'NONE', #335, #39518 ) ;
#18826=DIRECTION ( 'NONE',  ( -0.3090169943749573878, -0.9510565162951503115, 0.000000000000000000 ) ) ;
#18832=CARTESIAN_POINT ( 'NONE',  ( 12.80736835487433289, 15.68301270189216545, 7.000000000000000000 ) ) ;
#18834=EDGE_CURVE ( 'NONE', #23552, #18136, #23284, .T. ) ;
#18842=ORIENTED_EDGE ( 'NONE', *, *, #11014, .F. ) ;
#18844=ADVANCED_FACE ( 'NONE', ( #25553 ), #7468, .T. ) ;
#18846=ORIENTED_EDGE ( 'NONE', *, *, #13395, .T. ) ;
#18847=CARTESIAN_POINT ( 'NONE',  ( -2.518583951651200081, 7.712953814960714638, 7.000000000000000000 ) ) ;
#18848=CARTESIAN_POINT ( 'NONE',  ( 10.39021566973303656, 20.90519018800546291, 10.50000000000000000 ) ) ;
#18852=EDGE_LOOP ( 'NONE', ( #9795, #8971, #38786, #29077 ) ) ;
#18855=CARTESIAN_POINT ( 'NONE',  ( -0.9999999999999993339, 32.50000000000000000, 10.50000000000000178 ) ) ;
#18857=ADVANCED_FACE ( 'NONE', ( #26158 ), #35107, .F. ) ;
#18858=VECTOR ( 'NONE', #28092, 999.9999999999998863 ) ;
#18862=AXIS2_PLACEMENT_3D ( 'NONE', #13557, #23315, #25944 ) ;
#18865=CARTESIAN_POINT ( 'NONE',  ( -0.4999999999999998890, 37.50000000000000711, 7.000000000000000000 ) ) ;
#18867=CARTESIAN_POINT ( 'NONE',  ( 9.840690490415067160, 20.46019347195515792, 10.50000000000000533 ) ) ;
#18869=VERTEX_POINT ( 'NONE', #8075 ) ;
#18877=CARTESIAN_POINT ( 'NONE',  ( -10.59792294478258334, 33.06643021166741647, 10.49999999999999822 ) ) ;
#18881=EDGE_CURVE ( 'NONE', #7713, #37486, #39556, .T. ) ;
#18883=CARTESIAN_POINT ( 'NONE',  ( 8.412270287199628882, 10.07085245822955955, 10.59344459855562803 ) ) ;
#18884=CARTESIAN_POINT ( 'NONE',  ( 5.459721035625122454, 35.99203088905944981, 11.00000000000000000 ) ) ;
#18887=LINE ( 'NONE', #33930, #21217 ) ;
#18889=DIRECTION ( 'NONE',  ( -1.000000000000000000, 0.000000000000000000, 0.000000000000000000 ) ) ;
#18894=ORIENTED_EDGE ( 'NONE', *, *, #29593, .T. ) ;
#18901=VECTOR ( 'NONE', #37749, 1000.000000000000114 ) ;
#18902=DIRECTION ( 'NONE',  ( -0.000000000000000000, -0.000000000000000000, -1.000000000000000000 ) ) ;
#18903=DIRECTION ( 'NONE',  ( -1.000000000000000000, 0.000000000000000000, 0.000000000000000000 ) ) ;
#18905=CARTESIAN_POINT ( 'NONE',  ( 22.17929659509128371, 23.57150372095986057, 10.00000000000000000 ) ) ;
#18906=ORIENTED_EDGE ( 'NONE', *, *, #40178, .F. ) ;
#18907=CARTESIAN_POINT ( 'NONE',  ( -14.52509594610762456, 21.97885917798744870, 9.500000000000000000 ) ) ;
#18910=DIRECTION ( 'NONE',  ( -0.8660254037844364872, 0.5000000000000038858, 0.000000000000000000 ) ) ;
#18912=DIRECTION ( 'NONE',  ( 1.000000000000000000, 0.000000000000000000, 0.000000000000000000 ) ) ;
#18915=AXIS2_PLACEMENT_3D ( 'NONE', #31059, #21900, #21705 ) ;
#18917=EDGE_CURVE ( 'NONE', #8131, #38584, #29815, .T. ) ;
#18919=CARTESIAN_POINT ( 'NONE',  ( 9.363324537585983265, 32.27640801132196913, 10.50000000000000000 ) ) ;
#18920=DIRECTION ( 'NONE',  ( 0.000000000000000000, 0.000000000000000000, -1.000000000000000000 ) ) ;
#18925=CONICAL_SURFACE ( 'NONE', #770, 0.9999999999999991118, 0.7853981633974502774 ) ;
#18926=LINE ( 'NONE', #25816, #30906 ) ;
#18927=ORIENTED_EDGE ( 'NONE', *, *, #36802, .T. ) ;
#18928=VERTEX_POINT ( 'NONE', #14377 ) ;
#18932=VERTEX_POINT ( 'NONE', #17646 ) ;
#18938=LINE ( 'NONE', #3496, #5729 ) ;
#18939=DIRECTION ( 'NONE',  ( -1.000000000000000000, 0.000000000000000000, 0.000000000000000000 ) ) ;
#18940=ADVANCED_FACE ( 'NONE', ( #17239 ), #33285, .F. ) ;
#18941=VERTEX_POINT ( 'NONE', #26764 ) ;
#18943=ORIENTED_EDGE ( 'NONE', *, *, #6890, .F. ) ;
#18950=CARTESIAN_POINT ( 'NONE',  ( 5.383930013064285092, 36.46347792550310629, 10.49999999999999467 ) ) ;
#18951=LINE ( 'NONE', #30949, #22633 ) ;
#18954=CARTESIAN_POINT ( 'NONE',  ( -11.44473057578096764, 31.45924896672619298, 10.49999999999999822 ) ) ;
#18957=CARTESIAN_POINT ( 'NONE',  ( -4.096822963000304796, 8.035697679810704486, 10.49999999999999822 ) ) ;
#18959=DIRECTION ( 'NONE',  ( -0.6691306063588569053, 0.7431448254773954654, 0.000000000000000000 ) ) ;
#18962=EDGE_CURVE ( 'NONE', #29758, #20580, #4831, .T. ) ;
#18966=ORIENTED_EDGE ( 'NONE', *, *, #5317, .T. ) ;
#18968=CIRCLE ( 'NONE', #23499, 0.5000000000000004441 ) ;
#18972=ORIENTED_EDGE ( 'NONE', *, *, #34599, .F. ) ;
#18973=LINE ( 'NONE', #9637, #3436 ) ;
#18974=VERTEX_POINT ( 'NONE', #1790 ) ;
#18976=PLANE ( 'NONE',  #34161 ) ;
#18978=FACE_OUTER_BOUND ( 'NONE', #9982, .T. ) ;
#18979=ORIENTED_EDGE ( 'NONE', *, *, #19410, .T. ) ;
#18982=FACE_OUTER_BOUND ( 'NONE', #29336, .T. ) ;
#18984=VERTEX_POINT ( 'NONE', #32677 ) ;
#18986=CARTESIAN_POINT ( 'NONE',  ( 8.744117900323281845, 12.16605582823063614, 9.500000000000000000 ) ) ;
#18987=EDGE_CURVE ( 'NONE', #9209, #10038, #21364, .T. ) ;
#18988=LINE ( 'NONE', #34432, #16672 ) ;
#18989=EDGE_CURVE ( 'NONE', #26812, #11440, #33484, .T. ) ;
#18991=ORIENTED_EDGE ( 'NONE', *, *, #18262, .T. ) ;
#19000=CARTESIAN_POINT ( 'NONE',  ( 10.03245514394483529, 31.53326318584457510, 7.000000000000000000 ) ) ;
#19003=DIRECTION ( 'NONE',  ( 0.000000000000000000, 0.000000000000000000, 1.000000000000000000 ) ) ;
#19007=CARTESIAN_POINT ( 'NONE',  ( 14.31603901957230285, 19.98981538725070450, 10.49999999999999822 ) ) ;
#19010=CARTESIAN_POINT ( 'NONE',  ( -12.30736835487442882, 14.81698729810789672, 7.000000000000000000 ) ) ;
#19011=DIRECTION ( 'NONE',  ( 0.000000000000000000, 0.000000000000000000, -1.000000000000000000 ) ) ;
#19014=CARTESIAN_POINT ( 'NONE',  ( -6.654030453887829211, 35.94335816374515247, 7.500000000000000888 ) ) ;
#19018=CARTESIAN_POINT ( 'NONE',  ( 13.63581098909226874, 27.45627467658428955, 7.000000000000000000 ) ) ;
#19019=CARTESIAN_POINT ( 'NONE',  ( 13.09742388243072320, 16.09289933416717489, 10.49999999999999822 ) ) ;
#19025=DIRECTION ( 'NONE',  ( -1.000000000000000000, 0.000000000000000000, 0.000000000000000000 ) ) ;
#19027=CONICAL_SURFACE ( 'NONE', #14565, 1.000000000000002665, 0.7853981633974530530 ) ;
#19030=AXIS2_PLACEMENT_3D ( 'NONE', #39140, #23504, #36502 ) ;
#19039=EDGE_CURVE ( 'NONE', #17047, #28626, #36285, .T. ) ;
#19043=DIRECTION ( 'NONE',  ( 0.000000000000000000, -0.6729908358753945441, 0.7396508195275239839 ) ) ;
#19044=CARTESIAN_POINT ( 'NONE',  ( -14.33346043011695414, 20.15556903647894416, 10.66666666666666252 ) ) ;
#19048=CONICAL_SURFACE ( 'NONE', #20368, 0.4999999999999980571, 0.7853981633974548293 ) ;
#19049=VERTEX_POINT ( 'NONE', #5626 ) ;
#19050=VERTEX_POINT ( 'NONE', #14976 ) ;
#19055=ORIENTED_EDGE ( 'NONE', *, *, #11014, .T. ) ;
#19056=CIRCLE ( 'NONE', #6712, 0.5000000000000004441 ) ;
#19057=ADVANCED_FACE ( 'NONE', ( #27365 ), #32877, .T. ) ;
#19060=LINE ( 'NONE', #769, #5283 ) ;
#19062=CARTESIAN_POINT ( 'NONE',  ( -7.301172712743408511, 30.08322998587614805, 10.74999999999999467 ) ) ;
#19064=CIRCLE ( 'NONE', #1560, 15.00000000000000000 ) ;
#19066=EDGE_LOOP ( 'NONE', ( #24597, #8249, #21923 ) ) ;
#19067=EDGE_CURVE ( 'NONE', #22041, #23547, #10939, .T. ) ;
#19069=CARTESIAN_POINT ( 'NONE',  ( 5.440908595777815826, 35.94977745735560859, 9.500000000000000000 ) ) ;
#19071=CARTESIAN_POINT ( 'NONE',  ( -14.97009266215794021, 21.42933399866948463, 10.49999999999999822 ) ) ;
#19079=CARTESIAN_POINT ( 'NONE',  ( 13.90768907780713270, 27.88359266870271824, 10.49999999999999822 ) ) ;
#19080=CARTESIAN_POINT ( 'NONE',  ( 11.33320880805461606, 31.58310643763893211, 10.66666666666666607 ) ) ;
#19081=ORIENTED_EDGE ( 'NONE', *, *, #10096, .F. ) ;
#19083=EDGE_CURVE ( 'NONE', #23843, #32713, #32400, .T. ) ;
#19084=CARTESIAN_POINT ( 'NONE',  ( 8.315274455032101386, 10.01576150750513250, 7.500000000000000888 ) ) ;
#19085=EDGE_CURVE ( 'NONE', #12591, #31473, #7049, .T. ) ;
#19088=ORIENTED_EDGE ( 'NONE', *, *, #19083, .F. ) ;
#19090=CARTESIAN_POINT ( 'NONE',  ( -14.22382948751887177, 26.07014013211518133, 10.49999999999999645 ) ) ;
#19091=LINE ( 'NONE', #3649, #3092 ) ;
#19092=ORIENTED_EDGE ( 'NONE', *, *, #33302, .F. ) ;
#19097=AXIS2_PLACEMENT_3D ( 'NONE', #36013, #8173, #17737 ) ;
#19098=VERTEX_POINT ( 'NONE', #9686 ) ;
#19100=FACE_OUTER_BOUND ( 'NONE', #34740, .T. ) ;
#19101=CARTESIAN_POINT ( 'NONE',  ( -3.503793317224517700, 8.420815634768727520, 7.000000000000000000 ) ) ;
#19102=EDGE_CURVE ( 'NONE', #38835, #29659, #12524, .T. ) ;
#19106=ORIENTED_EDGE ( 'NONE', *, *, #35598, .T. ) ;
#19108=DIRECTION ( 'NONE',  ( 1.000000000000000000, 0.000000000000000000, 0.000000000000000000 ) ) ;
#19110=DIRECTION ( 'NONE',  ( 0.000000000000000000, 0.000000000000000000, 1.000000000000000000 ) ) ;
#19111=DIRECTION ( 'NONE',  ( 0.5877852522924689183, -0.8090169943749503378, 0.000000000000000000 ) ) ;
#19117=CARTESIAN_POINT ( 'NONE',  ( 14.47283171447379146, 21.48159823030311344, 7.000000000000000000 ) ) ;
#19118=VECTOR ( 'NONE', #28657, 1000.000000000000114 ) ;
#19119=ORIENTED_EDGE ( 'NONE', *, *, #37352, .F. ) ;
#19123=LINE ( 'NONE', #19521, #25041 ) ;
#19125=EDGE_LOOP ( 'NONE', ( #5757, #36850, #38874, #2597 ) ) ;
#19127=AXIS2_PLACEMENT_3D ( 'NONE', #39749, #23917, #2779 ) ;
#19130=VECTOR ( 'NONE', #27604, 1000.000000000000114 ) ;
#19133=CARTESIAN_POINT ( 'NONE',  ( -3.607749162633401507, 7.931741834401821123, 7.000000000000000000 ) ) ;
#19134=ORIENTED_EDGE ( 'NONE', *, *, #33510, .T. ) ;
#19137=DIRECTION ( 'NONE',  ( 0.9135454576425988682, -0.4067366430758048157, 3.469446951953606300E-15 ) ) ;
#19138=EDGE_CURVE ( 'NONE', #34728, #18136, #2985, .T. ) ;
#19145=VERTEX_POINT ( 'NONE', #6609 ) ;
#19146=CARTESIAN_POINT ( 'NONE',  ( -11.81630298851966288, 31.79381426990562787, 10.49999999999999822 ) ) ;
#19147=VECTOR ( 'NONE', #7126, 999.9999999999998863 ) ;
#19149=CARTESIAN_POINT ( 'NONE',  ( -11.44134295108998955, 15.31698729810788961, 9.500000000000000000 ) ) ;
#19150=LINE ( 'NONE', #31544, #1344 ) ;
#19151=CIRCLE ( 'NONE', #24354, 0.5000000000000000000 ) ;
#19153=CARTESIAN_POINT ( 'NONE',  ( -11.44169217588621201, 32.12932954397595608, 10.76099332938163933 ) ) ;
#19159=ORIENTED_EDGE ( 'NONE', *, *, #37728, .T. ) ;
#19162=CARTESIAN_POINT ( 'NONE',  ( 4.524139159579314118, 31.43208625488810171, 10.49999999999999822 ) ) ;
#19165=FACE_OUTER_BOUND ( 'NONE', #10540, .T. ) ;
#19170=PLANE ( 'NONE',  #39257 ) ;
#19171=ORIENTED_EDGE ( 'NONE', *, *, #11126, .F. ) ;
#19176=EDGE_LOOP ( 'NONE', ( #5566, #7970, #8141, #4646 ) ) ;
#19179=DIRECTION ( 'NONE',  ( 1.000000000000000000, 0.000000000000000000, 0.000000000000000000 ) ) ;
#19180=FACE_OUTER_BOUND ( 'NONE', #15080, .T. ) ;
#19181=FACE_OUTER_BOUND ( 'NONE', #14448, .T. ) ;
#19182=B_SPLINE_CURVE_WITH_KNOTS ( 'NONE', 3,
 ( #15169, #36907, #18030, #40145, #21071, #12123 ),
 .UNSPECIFIED., .F., .F.,
 ( 4, 2, 4 ),
 ( 0.000000000000000000, 0.5000000000000000000, 1.000000000000000000 ),
 .UNSPECIFIED. ) ;
#19184=ORIENTED_EDGE ( 'NONE', *, *, #36222, .F. ) ;
#19188=VECTOR ( 'NONE', #30675, 1000.000000000000000 ) ;
#19189=EDGE_CURVE ( 'NONE', #29941, #35073, #3576, .T. ) ;
#19194=LINE ( 'NONE', #7601, #24498 ) ;
#19195=ORIENTED_EDGE ( 'NONE', *, *, #38386, .T. ) ;
#19198=CARTESIAN_POINT ( 'NONE',  ( 8.401171878996485987, 21.11424711454080594, 9.000000000000001776 ) ) ;
#19200=CARTESIAN_POINT ( 'NONE',  ( -9.941034666242671847, 32.57396620494226624, 7.500000000000004441 ) ) ;
#19201=EDGE_CURVE ( 'NONE', #37486, #33852, #13552, .T. ) ;
#19203=EDGE_CURVE ( 'NONE', #2935, #13994, #1922, .T. ) ;
#19204=DIRECTION ( 'NONE',  ( -0.8660254037844432595, -0.4999999999999921729, 0.000000000000000000 ) ) ;
#19205=DIRECTION ( 'NONE',  ( 0.1045284632676570929, 0.9945218953682730678, 0.000000000000000000 ) ) ;
#19209=DIRECTION ( 'NONE',  ( 0.9781476007338067991, 0.2079116908177533474, 0.000000000000000000 ) ) ;
#19210=ORIENTED_EDGE ( 'NONE', *, *, #29777, .T. ) ;
#19213=DIRECTION ( 'NONE',  ( -0.000000000000000000, 0.000000000000000000, 1.000000000000000000 ) ) ;
#19218=ORIENTED_EDGE ( 'NONE', *, *, #35969, .T. ) ;
#19221=CARTESIAN_POINT ( 'NONE',  ( 3.531008893910514868, 8.292776413244014933, 11.00000000000000000 ) ) ;
#19229=CARTESIAN_POINT ( 'NONE',  ( 1.278175571583998194, 14.08178954835375940, 9.000000000000001776 ) ) ;
#19231=ORIENTED_EDGE ( 'NONE', *, *, #26619, .T. ) ;
#19233=EDGE_CURVE ( 'NONE', #2021, #35146, #18825, .T. ) ;
#19235=ORIENTED_EDGE ( 'NONE', *, *, #24665, .F. ) ;
#19236=CARTESIAN_POINT ( 'NONE',  ( 12.30736835487433112, 14.81698729810772797, 11.00000000000000000 ) ) ;
#19237=DIRECTION ( 'NONE',  ( -0.6691306063588670083, -0.7431448254773863615, 0.000000000000000000 ) ) ;
#19241=AXIS2_PLACEMENT_3D ( 'NONE', #7783, #32582, #11047 ) ;
#19242=ORIENTED_EDGE ( 'NONE', *, *, #1102, .T. ) ;
#19245=CARTESIAN_POINT ( 'NONE',  ( -1.000000000000000000, 37.00000000000000711, 10.50000000000000178 ) ) ;
#19246=CARTESIAN_POINT ( 'NONE',  ( 5.622359283595903534, 36.35732237484523921, 10.76099332938163933 ) ) ;
#19249=LINE ( 'NONE', #6264, #15251 ) ;
#19250=DIRECTION ( 'NONE',  ( 1.000000000000000000, 3.469446951953611033E-15, 0.000000000000000000 ) ) ;
#19251=EDGE_CURVE ( 'NONE', #23547, #39980, #37307, .T. ) ;
#19252=DIRECTION ( 'NONE',  ( 0.9135454576426059736, 0.4067366430757888285, 0.000000000000000000 ) ) ;
#19253=CARTESIAN_POINT ( 'NONE',  ( 15.35385137484828633, 7.606384166391536361, 10.00000000000000000 ) ) ;
#19254=CARTESIAN_POINT ( 'NONE',  ( -10.53831209642071975, 32.66155519649347383, 11.00000000000000000 ) ) ;
#19256=DIRECTION ( 'NONE',  ( 0.000000000000000000, 0.000000000000000000, 1.000000000000000000 ) ) ;
#19259=CARTESIAN_POINT ( 'NONE',  ( -12.05736835487443237, 14.38397459621567442, 10.50000000000000000 ) ) ;
#19260=CARTESIAN_POINT ( 'NONE',  ( -12.30736835487442882, 14.81698729810789672, 7.499999999999993783 ) ) ;
#19267=TOROIDAL_SURFACE ( 'NONE', #27707, 1.000000000000000000, 0.5000000000000000000 ) ;
#19272=CARTESIAN_POINT ( 'NONE',  ( 8.087160441415365497, 9.969847506822922867, 10.49999999999999822 ) ) ;
#19273=CARTESIAN_POINT ( 'NONE',  ( 5.578816091646283226, 36.25952276447326739, 10.87262190629270364 ) ) ;
#19274=VERTEX_POINT ( 'NONE', #37509 ) ;
#19277=ADVANCED_FACE ( 'NONE', ( #18428 ), #24321, .F. ) ;
#19279=LINE ( 'NONE', #31477, #33853 ) ;
#19282=EDGE_CURVE ( 'NONE', #26489, #36944, #11626, .T. ) ;
#19283=DIRECTION ( 'NONE',  ( -0.000000000000000000, 0.000000000000000000, 1.000000000000000000 ) ) ;
#19287=PLANE ( 'NONE',  #11220 ) ;
#19288=EDGE_LOOP ( 'NONE', ( #18732, #39496, #32247, #2624 ) ) ;
#19290=ADVANCED_FACE ( 'NONE', ( #132 ), #6225, .T. ) ;
#19291=EDGE_LOOP ( 'NONE', ( #34806, #30319, #35572 ) ) ;
#19294=CARTESIAN_POINT ( 'NONE',  ( -0.9008293819426604898, 37.47308728914261877, 7.382773698552460573 ) ) ;
#19297=VECTOR ( 'NONE', #39327, 999.9999999999998863 ) ;
#19298=CARTESIAN_POINT ( 'NONE',  ( -9.941034666242673623, 32.57396620494226624, 9.500000000000000000 ) ) ;
#19299=ORIENTED_EDGE ( 'NONE', *, *, #3347, .F. ) ;
#19301=CARTESIAN_POINT ( 'NONE',  ( 6.811226782241714517, 35.33967249274190436, 7.500000000000000888 ) ) ;
#19303=ADVANCED_FACE ( 'NONE', ( #30623 ), #5832, .T. ) ;
#19305=EDGE_CURVE ( 'NONE', #37355, #11442, #39571, .T. ) ;
#19308=VECTOR ( 'NONE', #32850, 999.9999999999998863 ) ;
#19310=ORIENTED_EDGE ( 'NONE', *, *, #39075, .F. ) ;
#19312=CARTESIAN_POINT ( 'NONE',  ( -6.354454053420243831, 35.54304081427989814, 7.000000000000000000 ) ) ;
#19313=DIRECTION ( 'NONE',  ( 0.7431448254773961315, 0.6691306063588561281, 0.000000000000000000 ) ) ;
#19321=AXIS2_PLACEMENT_3D ( 'NONE', #6316, #12818, #34759 ) ;
#19324=ADVANCED_FACE ( 'NONE', ( #5427 ), #18420, .F. ) ;
#19329=CARTESIAN_POINT ( 'NONE',  ( 6.762317648415093529, 29.93445088906596752, 10.50000000000000178 ) ) ;
#19330=EDGE_LOOP ( 'NONE', ( #25992, #22485, #36176, #39062 ) ) ;
#19336=EDGE_LOOP ( 'NONE', ( #36620, #14881, #2631, #26389, #35733 ) ) ;
#19338=PLANE ( 'NONE',  #11187 ) ;
#19339=ORIENTED_EDGE ( 'NONE', *, *, #33203, .T. ) ;
#19341=CIRCLE ( 'NONE', #16097, 0.5000000000000004441 ) ;
#19344=ORIENTED_EDGE ( 'NONE', *, *, #23942, .F. ) ;
#19346=DIRECTION ( 'NONE',  ( 0.8660254037844363761, -0.5000000000000039968, -0.000000000000000000 ) ) ;
#19348=DIRECTION ( 'NONE',  ( -0.4999999999999921729, 0.8660254037844432595, 0.000000000000000000 ) ) ;
#19350=CIRCLE ( 'NONE', #1858, 0.4999999999999988898 ) ;
#19351=CIRCLE ( 'NONE', #34300, 1.000000000000002665 ) ;
#19356=AXIS2_PLACEMENT_3D ( 'NONE', #1316, #35448, #7602 ) ;
#19357=DIRECTION ( 'NONE',  ( -1.224646799147351235E-16, 1.000000000000000000, 0.000000000000000000 ) ) ;
#19362=CARTESIAN_POINT ( 'NONE',  ( 10.66948297901455156, 33.02599466632828751, 10.49999999999999822 ) ) ;
#19366=CARTESIAN_POINT ( 'NONE',  ( -13.63581098909220479, 27.45627467658446008, 7.000000000000000000 ) ) ;
#19367=ORIENTED_EDGE ( 'NONE', *, *, #4167, .T. ) ;
#19371=CARTESIAN_POINT ( 'NONE',  ( 12.47058434440061880, 14.72275450261863838, 10.96580508970282430 ) ) ;
#19372=ORIENTED_EDGE ( 'NONE', *, *, #34556, .T. ) ;
#19375=CARTESIAN_POINT ( 'NONE',  ( -5.136393443230096167, 36.08535633838094725, 10.66666666666666785 ) ) ;
#19377=VERTEX_POINT ( 'NONE', #36709 ) ;
#19380=CARTESIAN_POINT ( 'NONE',  ( 4.984135866956514782, 36.15314577889351000, 7.500000000000000888 ) ) ;
#19381=DIRECTION ( 'NONE',  ( -0.000000000000000000, -0.000000000000000000, -1.000000000000000000 ) ) ;
#19386=VECTOR ( 'NONE', #32264, 1000.000000000000114 ) ;
#19388=ORIENTED_EDGE ( 'NONE', *, *, #27501, .F. ) ;
#19389=AXIS2_PLACEMENT_3D ( 'NONE', #19149, #19348, #3114 ) ;
#19391=DIRECTION ( 'NONE',  ( 0.000000000000000000, -1.000000000000000000, 0.000000000000000000 ) ) ;
#19394=LINE ( 'NONE', #9859, #12979 ) ;
#19395=DIRECTION ( 'NONE',  ( 0.9510565162951541973, 0.3090169943749456194, 0.000000000000000000 ) ) ;
#19397=DIRECTION ( 'NONE',  ( 0.9945218953682730678, -0.1045284632676569819, 0.000000000000000000 ) ) ;
#19400=CARTESIAN_POINT ( 'NONE',  ( 0.5000000000000000000, 37.00000000000000711, 7.500000000000000888 ) ) ;
#19401=CARTESIAN_POINT ( 'NONE',  ( -13.24038105676664401, 15.43301270189234486, 11.00000000000000000 ) ) ;
#19403=LINE ( 'NONE', #28749, #17999 ) ;
#19404=DIRECTION ( 'NONE',  ( -0.000000000000000000, -0.000000000000000000, -1.000000000000000000 ) ) ;
#19407=EDGE_LOOP ( 'NONE', ( #20137, #13920, #25669, #25187, #7233 ) ) ;
#19410=EDGE_CURVE ( 'NONE', #22335, #14611, #21263, .T. ) ;
#19411=CARTESIAN_POINT ( 'NONE',  ( 6.756943768455586863, 44.94911180988961519, 10.00000000000000000 ) ) ;
#19413=EDGE_CURVE ( 'NONE', #12432, #6323, #17469, .T. ) ;
#19414=DIRECTION ( 'NONE',  ( -0.000000000000000000, -0.000000000000000000, -1.000000000000000000 ) ) ;
#19418=AXIS2_PLACEMENT_3D ( 'NONE', #34152, #25201, #31298 ) ;
#19419=B_SPLINE_SURFACE_WITH_KNOTS ( 'NONE', 1, 3, ( 
 ( #16320, #16526, #28306, #26057, #34804, #6955, #29114, #678, #13058, #1285 ),
 ( #13667, #38051, #19362, #486, #6563, #28705, #25260, #12868, #37656, #9825 ) ),
 .UNSPECIFIED., .F., .F., .F.,
 ( 2, 2 ),
 ( 4, 2, 2, 2, 4 ),
 ( 0.000000000000000000, 1.000000000000000000 ),
 ( 2.137751973267104866, 2.530451054965827229, 2.923150136664549592, 3.315849218363272399, 3.708548300061994762 ),
 .UNSPECIFIED. ) ;
#19420=VERTEX_POINT ( 'NONE', #5618 ) ;
#19428=EDGE_LOOP ( 'NONE', ( #23459, #5049, #25068, #10363, #9996 ) ) ;
#19430=DIRECTION ( 'NONE',  ( -0.5877852522924796874, -0.8090169943749426773, 0.000000000000000000 ) ) ;
#19432=ORIENTED_EDGE ( 'NONE', *, *, #9857, .F. ) ;
#19438=EDGE_CURVE ( 'NONE', #9748, #21382, #4485, .T. ) ;
#19441=CONICAL_SURFACE ( 'NONE', #25272, 1.000000000000009548, 0.7853981633974567167 ) ;
#19442=VERTEX_POINT ( 'NONE', #11526 ) ;
#19446=CARTESIAN_POINT ( 'NONE',  ( 13.94482798346721530, 26.50521816028912525, 9.500000000000000000 ) ) ;
#19450=LINE ( 'NONE', #25150, #28239 ) ;
#19452=CYLINDRICAL_SURFACE ( 'NONE', #38998, 0.5000000000000004441 ) ;
#19453=DIRECTION ( 'NONE',  ( 1.000000000000000000, -6.938893903907210234E-15, 0.000000000000000000 ) ) ;
#19454=EDGE_CURVE ( 'NONE', #25405, #25736, #5823, .T. ) ;
#19455=DIRECTION ( 'NONE',  ( 1.000000000000000000, 0.000000000000000000, 0.000000000000000000 ) ) ;
#19460=DIRECTION ( 'NONE',  ( -0.7431448254773871387, 0.6691306063588662312, -6.938893903907226800E-15 ) ) ;
#19461=LINE ( 'NONE', #28407, #34793 ) ;
#19464=DIRECTION ( 'NONE',  ( 0.000000000000000000, -0.000000000000000000, 1.000000000000000000 ) ) ;
#19467=B_SPLINE_CURVE_WITH_KNOTS ( 'NONE', 3,
 ( #15136, #33244, #2356, #33445 ),
 .UNSPECIFIED., .F., .F.,
 ( 4, 4 ),
 ( 0.000000000000000000, 1.000000000000000000 ),
 .UNSPECIFIED. ) ;
#19475=EDGE_LOOP ( 'NONE', ( #28167, #17758, #17750 ) ) ;
#19476=VECTOR ( 'NONE', #17379, 1000.000000000000114 ) ;
#19478=CARTESIAN_POINT ( 'NONE',  ( 14.89501059309194808, 21.76138985984211160, 10.49999999999999822 ) ) ;
#19479=ORIENTED_EDGE ( 'NONE', *, *, #38826, .T. ) ;
#19481=CARTESIAN_POINT ( 'NONE',  ( 0.000000000000000000, 22.50000000000000355, 7.000000000000000000 ) ) ;
#19482=ADVANCED_FACE ( 'NONE', ( #17637 ), #33275, .F. ) ;
#19484=EDGE_CURVE ( 'NONE', #19098, #14611, #33864, .T. ) ;
#19488=ORIENTED_EDGE ( 'NONE', *, *, #4052, .T. ) ;
#19491=CONICAL_SURFACE ( 'NONE', #2654, 1.000000000000004441, 0.7853981633974524978 ) ;
#19494=DIRECTION ( 'NONE',  ( 0.2079116908177532919, -0.9781476007338070211, -0.000000000000000000 ) ) ;
#19495=DIRECTION ( 'NONE',  ( 0.000000000000000000, 0.000000000000000000, -1.000000000000000000 ) ) ;
#19496=CARTESIAN_POINT ( 'NONE',  ( 10.49474413300069386, 21.89971208337373909, 10.00000000000000000 ) ) ;
#19498=CARTESIAN_POINT ( 'NONE',  ( 2.568190708544436873, 12.82247983807080871, 10.50000000000000000 ) ) ;
#19499=VERTEX_POINT ( 'NONE', #17833 ) ;
#19500=( NAMED_UNIT ( * ) PLANE_ANGLE_UNIT ( ) SI_UNIT ( $, .RADIAN. ) );
#19505=EDGE_CURVE ( 'NONE', #18941, #6805, #18027, .T. ) ;
#19508=ORIENTED_EDGE ( 'NONE', *, *, #6413, .T. ) ;
#19511=FACE_OUTER_BOUND ( 'NONE', #8360, .T. ) ;
#19513=CARTESIAN_POINT ( 'NONE',  ( 12.67417846324118358, 14.47720745114811436, 7.499999999999997335 ) ) ;
#19514=B_SPLINE_CURVE_WITH_KNOTS ( 'NONE', 3,
 ( #16460, #28845, #32513, #7712, #17069, #10564 ),
 .UNSPECIFIED., .F., .F.,
 ( 4, 2, 4 ),
 ( 0.000000000000000000, 0.5000000000000000000, 1.000000000000000000 ),
 .UNSPECIFIED. ) ;
#19515=ORIENTED_EDGE ( 'NONE', *, *, #12356, .T. ) ;
#19517=VECTOR ( 'NONE', #7560, 1000.000000000000114 ) ;
#19520=AXIS2_PLACEMENT_3D ( 'NONE', #14569, #39348, #11525 ) ;
#19521=CARTESIAN_POINT ( 'NONE',  ( 3.610593701936705369, 31.83882289796390808, 10.50000000000000000 ) ) ;
#19522=ORIENTED_EDGE ( 'NONE', *, *, #25437, .T. ) ;
#19523=ORIENTED_EDGE ( 'NONE', *, *, #3467, .F. ) ;
#19525=FACE_OUTER_BOUND ( 'NONE', #30491, .T. ) ;
#19526=CARTESIAN_POINT ( 'NONE',  ( -12.74038105676667243, 14.56698729810793935, 10.59344459855562448 ) ) ;
#19532=CARTESIAN_POINT ( 'NONE',  ( 7.133890061153790541, 30.26901619224539175, 10.50000000000000000 ) ) ;
#19533=VECTOR ( 'NONE', #25154, 1000.000000000000114 ) ;
#19538=ADVANCED_FACE ( 'NONE', ( #27161 ), #26960, .T. ) ;
#19540=CARTESIAN_POINT ( 'NONE',  ( -13.63581098909220479, 27.45627467658446008, 7.000000000000000000 ) ) ;
#19542=VERTEX_POINT ( 'NONE', #27556 ) ;
#19548=AXIS2_PLACEMENT_3D ( 'NONE', #29095, #1268, #13652 ) ;
#19549=DIRECTION ( 'NONE',  ( 0.4731467892558179900, 0.5254827454987496260, 0.7071067811865524577 ) ) ;
#19552=EDGE_CURVE ( 'NONE', #28707, #10650, #33474, .T. ) ;
#19557=LINE ( 'NONE', #25649, #31930 ) ;
#19558=ORIENTED_EDGE ( 'NONE', *, *, #5610, .F. ) ;
#19560=ORIENTED_EDGE ( 'NONE', *, *, #10108, .F. ) ;
#19562=EDGE_CURVE ( 'NONE', #40105, #31103, #39744, .T. ) ;
#19564=DIRECTION ( 'NONE',  ( 1.000000000000000000, 0.000000000000000000, 0.000000000000000000 ) ) ;
#19566=ORIENTED_EDGE ( 'NONE', *, *, #3867, .T. ) ;
#19568=CARTESIAN_POINT ( 'NONE',  ( 16.38619327006176363, 7.072988944186805682, 11.00000000000000000 ) ) ;
#19571=DIRECTION ( 'NONE',  ( -0.000000000000000000, -0.000000000000000000, -1.000000000000000000 ) ) ;
#19574=AXIS2_PLACEMENT_3D ( 'NONE', #38344, #29604, #26149 ) ;
#19575=VERTEX_POINT ( 'NONE', #21654 ) ;
#19578=CARTESIAN_POINT ( 'NONE',  ( 10.06946225350410806, 32.23940090176269990, 9.500000000000000000 ) ) ;
#19582=PLANE ( 'NONE',  #5067 ) ;
#19583=CARTESIAN_POINT ( 'NONE',  ( 8.401171878996485987, 21.11424711454080594, 9.000000000000001776 ) ) ;
#19585=ADVANCED_FACE ( 'NONE', ( #12515 ), #15963, .F. ) ;
#19587=EDGE_CURVE ( 'NONE', #7787, #33406, #25490, .T. ) ;
#19590=ORIENTED_EDGE ( 'NONE', *, *, #6198, .F. ) ;
#19593=CARTESIAN_POINT ( 'NONE',  ( -12.30736835487442704, 14.81698729810789672, 7.000000000000000000 ) ) ;
#19594=LINE ( 'NONE', #32407, #33017 ) ;
#19597=DIRECTION ( 'NONE',  ( 1.000000000000000000, 0.000000000000000000, 0.000000000000000000 ) ) ;
#19599=AXIS2_PLACEMENT_3D ( 'NONE', #4114, #37841, #22396 ) ;
#19600=EDGE_CURVE ( 'NONE', #12521, #6531, #34361, .T. ) ;
#19601=CARTESIAN_POINT ( 'NONE',  ( 13.19371393710734708, 15.45995597598971116, 10.76099332938163933 ) ) ;
#19602=ORIENTED_EDGE ( 'NONE', *, *, #33203, .F. ) ;
#19603=DIRECTION ( 'NONE',  ( 0.000000000000000000, 0.000000000000000000, 1.000000000000000000 ) ) ;
#19604=B_SPLINE_CURVE_WITH_KNOTS ( 'NONE', 3,
 ( #32425, #12920, #26109, #16374 ),
 .UNSPECIFIED., .F., .F.,
 ( 4, 4 ),
 ( 0.000000000000000000, 1.000000000000000000 ),
 .UNSPECIFIED. ) ;
#19608=DIRECTION ( 'NONE',  ( 0.9945218953682746221, 0.1045284632676415221, -0.000000000000000000 ) ) ;
#19613=PLANE ( 'NONE',  #12095 ) ;
#19615=DIRECTION ( 'NONE',  ( -0.000000000000000000, -0.000000000000000000, -1.000000000000000000 ) ) ;
#19617=EDGE_LOOP ( 'NONE', ( #31995, #15692, #5433, #27563 ) ) ;
#19621=CARTESIAN_POINT ( 'NONE',  ( 3.607749162633204332, 7.931741834401770497, 10.49999999999999822 ) ) ;
#19624=VECTOR ( 'NONE', #3936, 1000.000000000000227 ) ;
#19628=ORIENTED_EDGE ( 'NONE', *, *, #27929, .T. ) ;
#19631=CARTESIAN_POINT ( 'NONE',  ( 2.525645716490518389, 8.212903943950921715, 11.00000000000000000 ) ) ;
#19636=EDGE_LOOP ( 'NONE', ( #24710, #18065, #31927 ) ) ;
#19638=CARTESIAN_POINT ( 'NONE',  ( 14.57736017774144877, 22.47612012567140383, 7.000000000000000000 ) ) ;
#19639=EDGE_CURVE ( 'NONE', #10420, #1897, #38241, .T. ) ;
#19646=CARTESIAN_POINT ( 'NONE',  ( -7.766013557953293400, 28.81973365084998306, 10.50000000000000000 ) ) ;
#19647=CIRCLE ( 'NONE', #16406, 0.5000000000000004441 ) ;
#19651=DIRECTION ( 'NONE',  ( -0.2079116908177663092, -0.9781476007338041345, 0.000000000000000000 ) ) ;
#19652=CARTESIAN_POINT ( 'NONE',  ( 12.30736835487432579, 14.81698729810772619, 11.00000000000000000 ) ) ;
#19654=DIRECTION ( 'NONE',  ( -0.000000000000000000, -0.000000000000000000, -1.000000000000000000 ) ) ;
#19655=CIRCLE ( 'NONE', #35236, 0.4999999999999999445 ) ;
#19656=DIRECTION ( 'NONE',  ( -0.7431448254773846962, 0.6691306063588690067, 0.000000000000000000 ) ) ;
#19658=CARTESIAN_POINT ( 'NONE',  ( -13.22516817658055288, 40.70288237343638826, 11.00000000000000000 ) ) ;
#19661=DIRECTION ( 'NONE',  ( -0.9135454576426004225, 0.4067366430758009854, -0.000000000000000000 ) ) ;
#19662=CLOSED_SHELL ( 'NONE', ( #34324, #26074, #17585, #35242, #3646, #12487, #38404, #29093, #30501, #9135, #30156, #1374, #14698, #15598, #8791, #5293, #17721, #6340, #20987, #18609, #20668, #5894, #35743, #32393, #5448, #28887, #10653, #9179, #38543, #20466, #17964, #29973, #1976, #10262, #12615, #6390, #12497, #13012, #29243, #31357, #19277, #20106, #9366, #36626, #2446, #15099, #22761, #30891, #2920, #26304, #29883, #25510, #36528, #10513, #28229, #4638, #30002, #27379, #31040, #1993, #38439, #39694, #23699, #18240, #13852, #25983, #31110, #10043, #36650, #6112, #28024, #14077, #28342, #2735, #16823, #37101, #16697, #9243, #30026, #23662, #27727, #17746, #17700, #20942, #6298, #10124, #10909, #16766, #29751, #24944, #17462, #33733, #6959, #1169, #33634, #7116, #12370, #33922, #15064, #31098, #19482, #18204, #17889, #38846, #29672, #37403, #30140, #7660, #16203, #27401, #12142, #17050, #1474, #22688, #23171, #15942, #34150, #8015, #34694, #19921, #38741, #22893, #30514, #23780, #2765, #7100, #9394, #20721, #10663, #25724, #6148, #40076, #29250, #23829, #39123, #18581, #24544, #19538, #38547, #5714, #21312, #19814, #30404, #2817, #2074, #38967, #39501, #30191, #21583, #19324, #13856, #21307, #14494, #1820, #34941, #3312, #38100, #22996, #10404, #37051, #29496, #39781, #38719, #34627, #5342, #9912, #3298, #40096, #4145, #10749, #32668, #36582, #1539, #3410, #24044, #28255, #26920, #20545, #30742, #34691, #37731, #4421, #38830, #23693, #28027, #22379, #29878, #30142, #7581, #30207, #1819, #4782, #16753, #39137, #15853, #13643, #6363, #16301, #12890, #563, #17574, #30715, #7767, #3774, #21944, #15523, #21359, #38323, #5661, #24208, #12762, #39349, #32617, #24057, #29039, #23128, #11288, #17488, #12093, #32593, #7148, #7797, #39195, #6837, #19585, #25271, #5849, #37311, #3920, #39645, #39656, #32492, #13243, #36579, #3798, #28687, #8066, #34127, #36226, #27043, #6867, #5270, #29139, #10992, #38610, #33152, #8656, #25996, #25643, #4657, #13135, #1923, #22808, #23206, #37759, #13053, #13089, #36700, #6909, #26409, #27548, #5193, #12263, #5065, #8907, #11409, #32900, #14756, #25152, #28608, #18538, #16074, #26163, #30240, #31223, #25044, #35867, #9521, #38644, #27121, #36446, #6273, #29019, #24812, #596, #13324, #5164, #27635, #39970, #24664, #7527, #26815, #22283, #136, #19792, #18038, #38695, #30847, #11212, #29395, #23963, #32174, #31986, #24446, #10651, #36953, #23640, #35644, #8788, #4914, #9107, #11388, #10239, #16353, #9668, #30740, #3848, #16668, #11713, #27858, #11841, #7765, #36898, #16102, #33889, #27823, #3150, #33126, #11635, #34201, #35721, #39219, #28747, #23331, #31789, #13342, #26454, #35839, #33857, #26491, #36693, #39469, #25672, #517, #34219, #19303, #24209, #28696, #25792, #29381, #35846, #20841, #16445, #18940, #18808, #15568, #30710, #24786, #11371, #15901, #2470, #36398, #4581, #33711, #14711, #5420, #25198, #38441, #8327, #23897, #7011, #38208, #25927, #38409, #26645, #12842, #7394, #1845, #16211, #17917, #33329, #15096, #21240, #14029, #14342, #21754, #9895, #37929, #5146, #13750, #39141, #9337, #35110, #37172, #5167, #3049, #7242, #12722, #18611, #8307, #16432, #9546, #34706, #27272, #3194, #2967, #17097, #27772, #24422, #5563, #28986, #26808, #40130, #28078, #5597, #14298, #25264, #15199, #4430, #23944, #18088, #15208, #12013, #5408, #37678, #15268, #37608, #12245, #12845, #35059, #36125, #19742, #35698, #28890, #18844, #27225, #1322, #34019, #19930, #6621, #34835, #7376, #17989, #5302, #33207, #38102, #39872, #31143, #6442, #26382, #19290, #31665, #6518, #38317, #31437, #23808, #18330, #22254, #18857, #18586, #2937, #17126, #39203, #26098, #32856, #8255, #34591, #1974, #22539, #32967, #2558, #29780, #2373, #35447, #12602, #39676, #10667, #6809, #1473, #2296, #23989, #4201, #30367, #34338, #15850, #21781, #6744, #35864, #9586, #31213, #21036, #32134, #32356, #5967, #6661, #22790, #25753, #16101, #9666, #6759, #36495, #17024, #28231, #40050, #8189, #23177, #30452, #24767, #5287, #3685, #19057, #27390, #36998, #2941, #31557, #9157, #15828, #7346, #10248, #19969, #39077, #28450, #29467, #33411, #4285, #18488, #20563, #25623, #13573, #28904, #10461, #34831, #14566, #28748, #26184, #1400, #31070, #2187, #18213, #12617, #18801, #37131, #62, #30808, #15254, #12642, #13986, #15368, #13216, #36795, #392, #31410, #23502, #8052, #39414, #9378, #37098, #27006, #4375, #40079, #26949, #15696, #28047, #30851, #24315, #35443, #8614, #20005, #2444, #23561, #24841, #38971, #27154 ) ) ;
#19663=DIRECTION ( 'NONE',  ( -0.000000000000000000, -0.000000000000000000, -1.000000000000000000 ) ) ;
#19664=EDGE_CURVE ( 'NONE', #21646, #27087, #33737, .T. ) ;
#19666=DIRECTION ( 'NONE',  ( 0.5000000000000041078, 0.8660254037844362651, 0.000000000000000000 ) ) ;
#19669=DIRECTION ( 'NONE',  ( -0.6123724356957950254, 0.3535533905932778387, -0.7071067811865450192 ) ) ;
#19670=VECTOR ( 'NONE', #5277, 1000.000000000000114 ) ;
#19680=CONICAL_SURFACE ( 'NONE', #23576, 1.000000000000004441, 0.7853981633974583820 ) ;
#19681=FACE_OUTER_BOUND ( 'NONE', #32077, .T. ) ;
#19682=ORIENTED_EDGE ( 'NONE', *, *, #2689, .F. ) ;
#19684=FACE_OUTER_BOUND ( 'NONE', #6857, .T. ) ;
#19687=ORIENTED_EDGE ( 'NONE', *, *, #31611, .T. ) ;
#19689=EDGE_CURVE ( 'NONE', #4287, #6957, #5158, .T. ) ;
#19691=ORIENTED_EDGE ( 'NONE', *, *, #23257, .T. ) ;
#19693=VECTOR ( 'NONE', #16967, 999.9999999999998863 ) ;
#19694=EDGE_CURVE ( 'NONE', #35769, #10247, #6216, .T. ) ;
#19695=EDGE_CURVE ( 'NONE', #24976, #16279, #34453, .T. ) ;
#19696=ORIENTED_EDGE ( 'NONE', *, *, #6052, .F. ) ;
#19701=LINE ( 'NONE', #32094, #5286 ) ;
#19704=AXIS2_PLACEMENT_3D ( 'NONE', #11727, #8679, #30814 ) ;
#19706=EDGE_LOOP ( 'NONE', ( #3258, #1141, #33591 ) ) ;
#19708=DIRECTION ( 'NONE',  ( 0.2185080122244179301, 0.6724985119639563802, 0.7071067811865462405 ) ) ;
#19712=VECTOR ( 'NONE', #10105, 1000.000000000000114 ) ;
#19713=ORIENTED_EDGE ( 'NONE', *, *, #37200, .T. ) ;
#19714=DIRECTION ( 'NONE',  ( 1.000000000000000000, 0.000000000000000000, 0.000000000000000000 ) ) ;
#19716=DIRECTION ( 'NONE',  ( 1.000000000000000000, 0.000000000000000000, 0.000000000000000000 ) ) ;
#19717=EDGE_CURVE ( 'NONE', #31091, #1084, #3961, .T. ) ;
#19718=EDGE_CURVE ( 'NONE', #29442, #22687, #31008, .T. ) ;
#19720=CARTESIAN_POINT ( 'NONE',  ( 13.05736835487433289, 16.11602540378438420, 7.499999999999997335 ) ) ;
#19721=CARTESIAN_POINT ( 'NONE',  ( 2.036571916123615100, 8.108948098542045457, 11.00000000000000000 ) ) ;
#19722=ORIENTED_EDGE ( 'NONE', *, *, #25769, .T. ) ;
#19727=FACE_OUTER_BOUND ( 'NONE', #22138, .T. ) ;
#19729=VERTEX_POINT ( 'NONE', #18621 ) ;
#19735=DIRECTION ( 'NONE',  ( -0.000000000000000000, -0.000000000000000000, -1.000000000000000000 ) ) ;
#19739=CARTESIAN_POINT ( 'NONE',  ( 14.81329996725644271, 19.93755115561686964, 10.49999999999999822 ) ) ;
#19740=ORIENTED_EDGE ( 'NONE', *, *, #4039, .F. ) ;
#19742=ADVANCED_FACE ( 'NONE', ( #125 ), #26585, .T. ) ;
#19743=CARTESIAN_POINT ( 'NONE',  ( -5.132330917503045598, 36.34800796123247579, 10.49999999999999822 ) ) ;
#19746=VECTOR ( 'NONE', #33858, 1000.000000000000000 ) ;
#19754=FACE_OUTER_BOUND ( 'NONE', #29884, .T. ) ;
#19755=B_SPLINE_SURFACE_WITH_KNOTS ( 'NONE', 1, 3, ( 
 ( #7137, #32344, #31926, #13642, #13436, #19743, #3159, #29288, #29084, #27937 ),
 ( #24689, #26030, #21639, #15550, #12496, #9459, #5305, #23596, #11408, #35992 ) ),
 .UNSPECIFIED., .F., .F., .F.,
 ( 2, 2 ),
 ( 4, 2, 2, 2, 4 ),
 ( 0.000000000000000000, 1.000000000000000000 ),
 ( 1.265795420569479912, 1.658494502268205162, 2.051193583966930412, 2.443892665665655439, 2.836591747364380467 ),
 .UNSPECIFIED. ) ;
#19756=AXIS2_PLACEMENT_3D ( 'NONE', #26211, #23573, #27019 ) ;
#19768=VECTOR ( 'NONE', #23152, 1000.000000000000000 ) ;
#19773=ORIENTED_EDGE ( 'NONE', *, *, #15585, .F. ) ;
#19776=ORIENTED_EDGE ( 'NONE', *, *, #34447, .F. ) ;
#19778=CARTESIAN_POINT ( 'NONE',  ( -22.37674264578614469, 24.85189042352228839, 11.00000000000000000 ) ) ;
#19781=ORIENTED_EDGE ( 'NONE', *, *, #22669, .T. ) ;
#19788=DIRECTION ( 'NONE',  ( 0.6123724356957886972, -0.3535533905932740639, -0.7071067811865525687 ) ) ;
#19792=ADVANCED_FACE ( 'NONE', ( #8016 ), #35454, .F. ) ;
#19801=CARTESIAN_POINT ( 'NONE',  ( 9.736411649803228485, 11.65093146000192625, 7.000000000000000000 ) ) ;
#19803=EDGE_CURVE ( 'NONE', #35819, #4586, #20219, .T. ) ;
#19804=AXIS2_PLACEMENT_3D ( 'NONE', #1908, #36031, #1294 ) ;
#19807=CARTESIAN_POINT ( 'NONE',  ( -11.25022250131745771, 31.95692947463384925, 10.96580508970282963 ) ) ;
#19808=CARTESIAN_POINT ( 'NONE',  ( -8.238488885696254371, 24.65111619403957022, 9.000000000000001776 ) ) ;
#19814=ADVANCED_FACE ( 'NONE', ( #7203 ), #29155, .T. ) ;
#19815=EDGE_CURVE ( 'NONE', #18376, #30328, #37607, .T. ) ;
#19817=DIRECTION ( 'NONE',  ( 1.000000000000000000, 0.000000000000000000, 0.000000000000000000 ) ) ;
#19818=EDGE_CURVE ( 'NONE', #13994, #31871, #1325, .T. ) ;
#19819=CIRCLE ( 'NONE', #16571, 0.5000000000000004441 ) ;
#19824=FACE_OUTER_BOUND ( 'NONE', #34891, .T. ) ;
#19832=DIRECTION ( 'NONE',  ( -1.000000000000000000, 0.000000000000000000, 0.000000000000000000 ) ) ;
#19840=ORIENTED_EDGE ( 'NONE', *, *, #8773, .F. ) ;
#19842=CARTESIAN_POINT ( 'NONE',  ( 0.000000000000000000, 22.50000000000000355, 7.000000000000000000 ) ) ;
#19848=PLANE ( 'NONE',  #6612 ) ;
#19849=VERTEX_POINT ( 'NONE', #4571 ) ;
#19851=CYLINDRICAL_SURFACE ( 'NONE', #40035, 0.5000000000000004441 ) ;
#19852=CARTESIAN_POINT ( 'NONE',  ( -3.607749162633400619, 7.931741834401826452, 10.50000000000000000 ) ) ;
#19853=B_SPLINE_CURVE_WITH_KNOTS ( 'NONE', 3,
 ( #15272, #18133, #36808, #27263 ),
 .UNSPECIFIED., .F., .F.,
 ( 4, 4 ),
 ( 0.000000000000000000, 1.000000000000000000 ),
 .UNSPECIFIED. ) ;
#19856=ORIENTED_EDGE ( 'NONE', *, *, #28150, .F. ) ;
#19857=CARTESIAN_POINT ( 'NONE',  ( 13.63581098909226519, 27.45627467658428600, 11.00000000000000000 ) ) ;
#19859=CARTESIAN_POINT ( 'NONE',  ( 0.000000000000000000, 22.50000000000000355, 7.000000000000000000 ) ) ;
#19861=VECTOR ( 'NONE', #8124, 999.9999999999998863 ) ;
#19862=DIRECTION ( 'NONE',  ( 0.000000000000000000, -0.000000000000000000, -1.000000000000000000 ) ) ;
#19865=CARTESIAN_POINT ( 'NONE',  ( -13.81813021740780201, 28.33725983961547001, 7.102474990965858659 ) ) ;
#19868=FACE_OUTER_BOUND ( 'NONE', #20410, .T. ) ;
#19869=CARTESIAN_POINT ( 'NONE',  ( 10.33795143809920170, 20.40792924032133016, 11.00000000000000000 ) ) ;
#19870=CARTESIAN_POINT ( 'NONE',  ( 9.337241587065685522, 10.76617146908747991, 10.49999999999999467 ) ) ;
#19873=ORIENTED_EDGE ( 'NONE', *, *, #33108, .T. ) ;
#19875=DIRECTION ( 'NONE',  ( 0.1470157664652038954, 0.6916548014802263999, -0.7071067811865456854 ) ) ;
#19876=CARTESIAN_POINT ( 'NONE',  ( -12.80736835487442349, 15.68301270189233954, 11.00000000000000000 ) ) ;
#19878=CARTESIAN_POINT ( 'NONE',  ( -13.63581098909220302, 27.45627467658446719, 11.00000000000000000 ) ) ;
#19886=DIRECTION ( 'NONE',  ( -0.2079116908177664480, -0.9781476007338042455, 0.000000000000000000 ) ) ;
#19887=CARTESIAN_POINT ( 'NONE',  ( 1.000000000000000000, 37.00000000000000711, 7.500000000000000888 ) ) ;
#19890=ORIENTED_EDGE ( 'NONE', *, *, #15000, .T. ) ;
#19894=VERTEX_POINT ( 'NONE', #4773 ) ;
#19896=DIRECTION ( 'NONE',  ( -1.000000000000000000, 0.000000000000000000, 0.000000000000000000 ) ) ;
#19900=ORIENTED_EDGE ( 'NONE', *, *, #39075, .T. ) ;
#19902=EDGE_LOOP ( 'NONE', ( #27584, #3047, #3871, #6186 ) ) ;
#19905=CARTESIAN_POINT ( 'NONE',  ( 6.354454053420414361, 35.54304081427980577, 7.500000000000000888 ) ) ;
#19906=CARTESIAN_POINT ( 'NONE',  ( -9.892954722048926897, 20.95745441963942568, 10.50000000000000000 ) ) ;
#19908=CARTESIAN_POINT ( 'NONE',  ( 9.126760388790467360, 17.80801270189218144, 10.74999999999999467 ) ) ;
#19909=EDGE_LOOP ( 'NONE', ( #24046, #413, #38974, #38716 ) ) ;
#19910=FILL_AREA_STYLE_COLOUR ( '', #31358 ) ;
#19911=LINE ( 'NONE', #32307, #36628 ) ;
#19912=DIRECTION ( 'NONE',  ( -0.4731467892558146038, -0.5254827454987658353, -0.7071067811865425767 ) ) ;
#19917=VECTOR ( 'NONE', #29024, 1000.000000000000227 ) ;
#19920=LINE ( 'NONE', #12663, #28540 ) ;
#19921=ADVANCED_FACE ( 'NONE', ( #7407 ), #20017, .T. ) ;
#19923=DIRECTION ( 'NONE',  ( -0.000000000000000000, -0.000000000000000000, -1.000000000000000000 ) ) ;
#19925=ORIENTED_EDGE ( 'NONE', *, *, #35228, .F. ) ;
#19926=CONICAL_SURFACE ( 'NONE', #9576, 1.000000000000000444, 0.7853981633974482790 ) ;
#19930=ADVANCED_FACE ( 'NONE', ( #4975 ), #19441, .T. ) ;
#19931=DIRECTION ( 'NONE',  ( -0.9510565162951503115, 0.3090169943749572767, 0.000000000000000000 ) ) ;
#19932=EDGE_CURVE ( 'NONE', #34769, #11836, #1805, .T. ) ;
#19937=CARTESIAN_POINT ( 'NONE',  ( -12.47058434440077512, 14.72275450261881602, 10.96580508970281187 ) ) ;
#19939=PLANE ( 'NONE',  #31254 ) ;
#19940=ORIENTED_EDGE ( 'NONE', *, *, #40176, .F. ) ;
#19942=DIRECTION ( 'NONE',  ( -1.000000000000000000, 0.000000000000000000, 0.000000000000000000 ) ) ;
#19946=CARTESIAN_POINT ( 'NONE',  ( -5.198706521309195416, 29.65540566576573767, 9.000000000000001776 ) ) ;
#19949=VECTOR ( 'NONE', #33986, 1000.000000000000000 ) ;
#19950=VECTOR ( 'NONE', #21682, 1000.000000000000114 ) ;
#19951=DIRECTION ( 'NONE',  ( -0.000000000000000000, -0.000000000000000000, -1.000000000000000000 ) ) ;
#19954=VERTEX_POINT ( 'NONE', #10875 ) ;
#19961=DIRECTION ( 'NONE',  ( 0.000000000000000000, 0.000000000000000000, 1.000000000000000000 ) ) ;
#19962=CARTESIAN_POINT ( 'NONE',  ( -8.189058612310551766, 9.932416477787068487, 7.455686640544901600 ) ) ;
#19968=FACE_OUTER_BOUND ( 'NONE', #5472, .T. ) ;
#19969=ADVANCED_FACE ( 'NONE', ( #13914 ), #26308, .T. ) ;
#19970=ORIENTED_EDGE ( 'NONE', *, *, #39168, .T. ) ;
#19973=VERTEX_POINT ( 'NONE', #9025 ) ;
#19975=CIRCLE ( 'NONE', #21282, 0.4999999999999997224 ) ;
#19977=CARTESIAN_POINT ( 'NONE',  ( -14.39395135575592377, 26.65114718998442811, 10.68306085400104699 ) ) ;
#19979=ORIENTED_EDGE ( 'NONE', *, *, #14965, .T. ) ;
#19981=DIRECTION ( 'NONE',  ( 0.9510565162951497564, -0.3090169943749591086, 0.000000000000000000 ) ) ;
#19983=CIRCLE ( 'NONE', #1836, 0.5000000000000001110 ) ;
#19985=DIRECTION ( 'NONE',  ( 0.000000000000000000, 0.000000000000000000, -1.000000000000000000 ) ) ;
#19987=DIRECTION ( 'NONE',  ( 0.000000000000000000, 0.000000000000000000, 1.000000000000000000 ) ) ;
#19989=ORIENTED_EDGE ( 'NONE', *, *, #30204, .F. ) ;
#19992=DIRECTION ( 'NONE',  ( 1.000000000000000000, 0.000000000000000000, 0.000000000000000000 ) ) ;
#20003=ORIENTED_EDGE ( 'NONE', *, *, #14773, .T. ) ;
#20005=ADVANCED_FACE ( 'NONE', ( #20626 ), #30567, .F. ) ;
#20007=CARTESIAN_POINT ( 'NONE',  ( -8.816778784387198087, 10.36474508437586195, 7.000000000000000000 ) ) ;
#20010=AXIS2_PLACEMENT_3D ( 'NONE', #30654, #11959, #37541 ) ;
#20011=AXIS2_PLACEMENT_3D ( 'NONE', #34933, #22522, #10957 ) ;
#20012=CARTESIAN_POINT ( 'NONE',  ( -7.014595103779441843, 35.79644522156330311, 10.50000000000000000 ) ) ;
#20015=ORIENTED_EDGE ( 'NONE', *, *, #36732, .F. ) ;
#20016=CYLINDRICAL_SURFACE ( 'NONE', #37683, 0.4999999999999997780 ) ;
#20017=PLANE ( 'NONE',  #29161 ) ;
#20019=CARTESIAN_POINT ( 'NONE',  ( 14.86556419889027048, 20.43481210330100240, 10.49999999999999822 ) ) ;
#20020=CARTESIAN_POINT ( 'NONE',  ( 10.47804177580207607, 33.28010392086025604, 11.00000000000000000 ) ) ;
#20023=LINE ( 'NONE', #13511, #36014 ) ;
#20024=ORIENTED_EDGE ( 'NONE', *, *, #10761, .T. ) ;
#20029=DIRECTION ( 'NONE',  ( 0.6916548014802259559, -0.1470157664652035345, -0.7071067811865460184 ) ) ;
#20031=ORIENTED_EDGE ( 'NONE', *, *, #10527, .T. ) ;
#20033=ORIENTED_EDGE ( 'NONE', *, *, #7160, .T. ) ;
#20035=CARTESIAN_POINT ( 'NONE',  ( 14.09933648065468503, 26.02968990214155198, 10.49999999999999822 ) ) ;
#20038=AXIS2_PLACEMENT_3D ( 'NONE', #26134, #23495, #26948 ) ;
#20039=AXIS2_PLACEMENT_3D ( 'NONE', #38555, #7261, #10729 ) ;
#20043=ORIENTED_EDGE ( 'NONE', *, *, #23125, .F. ) ;
#20047=DIRECTION ( 'NONE',  ( 0.000000000000000000, 0.000000000000000000, -1.000000000000000000 ) ) ;
#20052=VERTEX_POINT ( 'NONE', #8428 ) ;
#20055=EDGE_CURVE ( 'NONE', #13272, #21146, #12946, .T. ) ;
#20056=LINE ( 'NONE', #17423, #30703 ) ;
#20060=ORIENTED_EDGE ( 'NONE', *, *, #24188, .T. ) ;
#20061=FACE_OUTER_BOUND ( 'NONE', #21219, .T. ) ;
#20063=AXIS2_PLACEMENT_3D ( 'NONE', #28757, #13110, #16173 ) ;
#20064=VECTOR ( 'NONE', #8270, 1000.000000000000114 ) ;
#20066=ORIENTED_EDGE ( 'NONE', *, *, #24764, .F. ) ;
#20068=CARTESIAN_POINT ( 'NONE',  ( -14.98531754163844276, 21.83276651127755486, 7.381627713044571770 ) ) ;
#20069=CARTESIAN_POINT ( 'NONE',  ( 13.88403039571024244, 27.53692605078171241, 10.94611345180490503 ) ) ;
#20070=PLANE ( 'NONE',  #7196 ) ;
#20071=DIRECTION ( 'NONE',  ( -0.7071067811865479058, 0.000000000000000000, -0.7071067811865472397 ) ) ;
#20072=EDGE_CURVE ( 'NONE', #15678, #21190, #27110, .T. ) ;
#20073=CARTESIAN_POINT ( 'NONE',  ( 2.629601561899396422, 7.723830143584012653, 10.50000000000000000 ) ) ;
#20075=CARTESIAN_POINT ( 'NONE',  ( -12.74038105676665289, 14.56698729810790027, 10.63089969389957368 ) ) ;
#20076=ORIENTED_EDGE ( 'NONE', *, *, #18697, .F. ) ;
#20079=CARTESIAN_POINT ( 'NONE',  ( -0.8726219062944396976, 37.33905845026552583, 10.49999999999999822 ) ) ;
#20082=DIRECTION ( 'NONE',  ( 0.6459741880212489518, 0.2876062384759403012, -0.7071067811865537900 ) ) ;
#20086=EDGE_CURVE ( 'NONE', #22029, #12954, #29801, .T. ) ;
#20091=DIRECTION ( 'NONE',  ( 0.000000000000000000, 0.000000000000000000, 1.000000000000000000 ) ) ;
#20092=ORIENTED_EDGE ( 'NONE', *, *, #18115, .T. ) ;
#20097=ORIENTED_EDGE ( 'NONE', *, *, #21664, .T. ) ;
#20098=DIRECTION ( 'NONE',  ( -0.000000000000000000, 0.000000000000000000, 1.000000000000000000 ) ) ;
#20099=CARTESIAN_POINT ( 'NONE',  ( 9.296885549838558305, 10.71356306745936138, 10.49999999999999822 ) ) ;
#20100=AXIS2_PLACEMENT_3D ( 'NONE', #11167, #35754, #20722 ) ;
#20104=VERTEX_POINT ( 'NONE', #2133 ) ;
#20106=ADVANCED_FACE ( 'NONE', ( #5569 ), #14517, .T. ) ;
#20112=FACE_OUTER_BOUND ( 'NONE', #34146, .T. ) ;
#20114=DIRECTION ( 'NONE',  ( -0.6691306063588671194, -0.7431448254773863615, 0.000000000000000000 ) ) ;
#20117=PLANE ( 'NONE',  #5500 ) ;
#20119=LINE ( 'NONE', #32520, #22115 ) ;
#20123=EDGE_LOOP ( 'NONE', ( #39563, #13679, #8465 ) ) ;
#20125=CARTESIAN_POINT ( 'NONE',  ( -3.813962023474482876, 32.29559562678526419, 10.50000000000000000 ) ) ;
#20128=DIRECTION ( 'NONE',  ( 0.2185080122244175416, 0.6724985119639551590, -0.7071067811865474617 ) ) ;
#20129=CIRCLE ( 'NONE', #9105, 0.5000000000000004441 ) ;
#20130=DIRECTION ( 'NONE',  ( -1.224646799147351235E-16, 1.000000000000000000, 0.000000000000000000 ) ) ;
#20131=VERTEX_POINT ( 'NONE', #2534 ) ;
#20135=DIRECTION ( 'NONE',  ( 0.9510565162951544194, 0.3090169943749449533, -0.000000000000000000 ) ) ;
#20136=ORIENTED_EDGE ( 'NONE', *, *, #5319, .T. ) ;
#20137=ORIENTED_EDGE ( 'NONE', *, *, #3640, .F. ) ;
#20139=CARTESIAN_POINT ( 'NONE',  ( 8.410254037844358876, 17.06698729810774395, 10.50000000000000000 ) ) ;
#20143=DIRECTION ( 'NONE',  ( 1.000000000000000000, 0.000000000000000000, -0.000000000000000000 ) ) ;
#20144=VERTEX_POINT ( 'NONE', #5965 ) ;
#20146=CARTESIAN_POINT ( 'NONE',  ( -13.63581098909220479, 27.45627467658446008, 7.000000000000000000 ) ) ;
#20147=DIRECTION ( 'NONE',  ( 0.000000000000000000, 0.000000000000000000, -1.000000000000000000 ) ) ;
#20148=CARTESIAN_POINT ( 'NONE',  ( -2.525645716490712012, 8.212903943950955465, 7.000000000000000000 ) ) ;
#20149=ORIENTED_EDGE ( 'NONE', *, *, #4610, .F. ) ;
#20151=PLANE ( 'NONE',  #6014 ) ;
#20152=ORIENTED_EDGE ( 'NONE', *, *, #31119, .F. ) ;
#20155=VERTEX_POINT ( 'NONE', #33224 ) ;
#20158=CIRCLE ( 'NONE', #29255, 0.5000000000000004441 ) ;
#20160=FACE_OUTER_BOUND ( 'NONE', #603, .T. ) ;
#20162=DIRECTION ( 'NONE',  ( -0.07391278520356001080, 0.7032331762534130837, -0.7071067811865392461 ) ) ;
#20164=CARTESIAN_POINT ( 'NONE',  ( 0.5000000000000001110, 37.00000000000000711, 7.000000000000000000 ) ) ;
#20167=VECTOR ( 'NONE', #33811, 1000.000000000000000 ) ;
#20168=CARTESIAN_POINT ( 'NONE',  ( 0.4999999999999995559, 37.00000000000000711, 11.00000000000000000 ) ) ;
#20172=PLANE ( 'NONE',  #28683 ) ;
#20176=ORIENTED_EDGE ( 'NONE', *, *, #26288, .F. ) ;
#20179=EDGE_CURVE ( 'NONE', #31776, #21244, #35024, .T. ) ;
#20182=ORIENTED_EDGE ( 'NONE', *, *, #33614, .T. ) ;
#20190=VERTEX_POINT ( 'NONE', #7310 ) ;
#20195=VERTEX_POINT ( 'NONE', #12270 ) ;
#20198=DIRECTION ( 'NONE',  ( -0.4067366430757888285, 0.9135454576426059736, -0.000000000000000000 ) ) ;
#20202=VECTOR ( 'NONE', #40034, 1000.000000000000000 ) ;
#20204=CIRCLE ( 'NONE', #35096, 6.000000000000003553 ) ;
#20205=EDGE_CURVE ( 'NONE', #26597, #20501, #24657, .T. ) ;
#20209=CARTESIAN_POINT ( 'NONE',  ( -5.440908595777638190, 35.94977745735568675, 11.00000000000000000 ) ) ;
#20210=DIRECTION ( 'NONE',  ( 0.8090169943749426773, -0.5877852522924796874, -0.000000000000000000 ) ) ;
#20212=EDGE_CURVE ( 'NONE', #39810, #23537, #1235, .T. ) ;
#20214=CARTESIAN_POINT ( 'NONE',  ( -8.315274455032216849, 10.01576150750520888, 7.000000000000000000 ) ) ;
#20215=CARTESIAN_POINT ( 'NONE',  ( 5.440908595777817602, 35.94977745735560859, 7.000000000000000000 ) ) ;
#20218=DIRECTION ( 'NONE',  ( 0.4067366430757984874, 0.9135454576426016438, -2.081668171172158416E-14 ) ) ;
#20219=LINE ( 'NONE', #29351, #27856 ) ;
#20221=FACE_OUTER_BOUND ( 'NONE', #20123, .T. ) ;
#20222=CARTESIAN_POINT ( 'NONE',  ( -14.41430201638242714, 20.48224166989796302, 11.00000000000000355 ) ) ;
#20225=ORIENTED_EDGE ( 'NONE', *, *, #37697, .F. ) ;
#20226=AXIS2_PLACEMENT_3D ( 'NONE', #24155, #39197, #20914 ) ;
#20229=AXIS2_PLACEMENT_3D ( 'NONE', #40186, #6260, #3018 ) ;
#20232=EDGE_CURVE ( 'NONE', #30940, #24654, #31139, .T. ) ;
#20235=ORIENTED_EDGE ( 'NONE', *, *, #892, .F. ) ;
#20237=ORIENTED_EDGE ( 'NONE', *, *, #5391, .T. ) ;
#20248=AXIS2_PLACEMENT_3D ( 'NONE', #12389, #2457, #14844 ) ;
#20250=PLANE ( 'NONE',  #5679 ) ;
#20251=ORIENTED_EDGE ( 'NONE', *, *, #14856, .T. ) ;
#20255=CARTESIAN_POINT ( 'NONE',  ( 6.282361020112160688, 14.70372268239673197, 10.50000000000000000 ) ) ;
#20257=DIRECTION ( 'NONE',  ( -0.9781476007338069101, -0.2079116908177532363, 0.000000000000000000 ) ) ;
#20259=DIRECTION ( 'NONE',  ( -1.000000000000000000, 0.000000000000000000, 0.000000000000000000 ) ) ;
#20260=ORIENTED_EDGE ( 'NONE', *, *, #5443, .T. ) ;
#20261=CARTESIAN_POINT ( 'NONE',  ( -3.000488737322915878, 30.46850471150003159, 7.000000000000000000 ) ) ;
#20262=DIRECTION ( 'NONE',  ( 0.000000000000000000, 0.7071067811865500152, -0.7071067811865451302 ) ) ;
#20263=CARTESIAN_POINT ( 'NONE',  ( 6.557822374958315770, 35.99981354310111215, 10.50000000000000000 ) ) ;
#20266=CARTESIAN_POINT ( 'NONE',  ( -14.96930490892015797, 21.54088032874991399, 7.500000000000004441 ) ) ;
#20267=FACE_OUTER_BOUND ( 'NONE', #1574, .T. ) ;
#20268=AXIS2_PLACEMENT_3D ( 'NONE', #39926, #2168, #8252 ) ;
#20273=DIRECTION ( 'NONE',  ( -0.3090169943749560000, -0.9510565162951507556, 0.000000000000000000 ) ) ;
#20275=VECTOR ( 'NONE', #9446, 1000.000000000000000 ) ;
#20278=CARTESIAN_POINT ( 'NONE',  ( -0.4999999999999964473, 37.50000000000000711, 10.49999999999999822 ) ) ;
#20280=DIRECTION ( 'NONE',  ( 0.7071067811865499042, 0.000000000000000000, 0.7071067811865451302 ) ) ;
#20283=CARTESIAN_POINT ( 'NONE',  ( 12.41947502333593967, 43.35441443594645250, 7.000000000000000000 ) ) ;
#20290=CARTESIAN_POINT ( 'NONE',  ( -5.440908595777636414, 35.94977745735568675, 9.000000000000001776 ) ) ;
#20297=DIRECTION ( 'NONE',  ( -0.2079116908177664202, -0.9781476007338041345, 0.000000000000000000 ) ) ;
#20299=LINE ( 'NONE', #36140, #29748 ) ;
#20300=ORIENTED_EDGE ( 'NONE', *, *, #10007, .F. ) ;
#20303=ORIENTED_EDGE ( 'NONE', *, *, #32474, .T. ) ;
#20306=EDGE_CURVE ( 'NONE', #9166, #11008, #21804, .T. ) ;
#20307=ORIENTED_EDGE ( 'NONE', *, *, #31638, .F. ) ;
#20308=CARTESIAN_POINT ( 'NONE',  ( 13.97943872024082346, 27.84235072122924137, 10.49999999999999467 ) ) ;
#20309=EDGE_LOOP ( 'NONE', ( #9877, #32732, #8161, #15482 ) ) ;
#20311=DIRECTION ( 'NONE',  ( -0.000000000000000000, -0.000000000000000000, -1.000000000000000000 ) ) ;
#20314=EDGE_CURVE ( 'NONE', #8575, #36455, #4541, .T. ) ;
#20315=DIRECTION ( 'NONE',  ( 0.4067366430758010409, 0.9135454576426005335, -0.000000000000000000 ) ) ;
#20316=ORIENTED_EDGE ( 'NONE', *, *, #15575, .F. ) ;
#20318=FACE_OUTER_BOUND ( 'NONE', #3949, .T. ) ;
#20321=AXIS2_PLACEMENT_3D ( 'NONE', #23899, #35493, #20665 ) ;
#20323=ORIENTED_EDGE ( 'NONE', *, *, #15204, .T. ) ;
#20325=PLANE ( 'NONE',  #20769 ) ;
#20326=VECTOR ( 'NONE', #3926, 1000.000000000000000 ) ;
#20329=EDGE_CURVE ( 'NONE', #2112, #28965, #33764, .T. ) ;
#20331=DIRECTION ( 'NONE',  ( -0.9945218953682742891, -0.1045284632676437564, 0.000000000000000000 ) ) ;
#20332=EDGE_CURVE ( 'NONE', #34846, #26679, #19920, .T. ) ;
#20333=ORIENTED_EDGE ( 'NONE', *, *, #6989, .F. ) ;
#20335=CIRCLE ( 'NONE', #15767, 1.000000000000007772 ) ;
#20338=DIRECTION ( 'NONE',  ( 0.2079116908177533474, -0.9781476007338067991, 0.000000000000000000 ) ) ;
#20342=CARTESIAN_POINT ( 'NONE',  ( 14.97009266215792778, 21.42933399866928568, 11.00000000000000000 ) ) ;
#20343=CIRCLE ( 'NONE', #16449, 0.9999999999999995559 ) ;
#20346=CARTESIAN_POINT ( 'NONE',  ( -14.97283171447380390, 21.48159823030330884, 11.00000000000000000 ) ) ;
#20349=DIRECTION ( 'NONE',  ( 0.8090169943749504489, 0.5877852522924689183, 0.000000000000000000 ) ) ;
#20351=CARTESIAN_POINT ( 'NONE',  ( -2.141014423450144033, 7.887532638883575586, 10.49999999999999822 ) ) ;
#20352=ORIENTED_EDGE ( 'NONE', *, *, #19600, .T. ) ;
#20354=DIRECTION ( 'NONE',  ( 0.1045284632676436315, -0.9945218953682742891, 0.000000000000000000 ) ) ;
#20355=EDGE_CURVE ( 'NONE', #35442, #29211, #15558, .T. ) ;
#20358=VECTOR ( 'NONE', #28347, 1000.000000000000114 ) ;
#20360=EDGE_CURVE ( 'NONE', #4426, #12819, #6169, .T. ) ;
#20364=B_SPLINE_CURVE_WITH_KNOTS ( 'NONE', 3,
 ( #22314, #25560, #37362, #34714 ),
 .UNSPECIFIED., .F., .F.,
 ( 4, 4 ),
 ( 0.000000000000000000, 0.3999999999265801964 ),
 .UNSPECIFIED. ) ;
#20368=AXIS2_PLACEMENT_3D ( 'NONE', #26394, #23553, #38188 ) ;
#20370=EDGE_LOOP ( 'NONE', ( #29629, #4669, #29153 ) ) ;
#20371=DIRECTION ( 'NONE',  ( -0.9510565162951504226, 0.3090169943749573322, 0.000000000000000000 ) ) ;
#20373=LINE ( 'NONE', #4925, #25572 ) ;
#20374=AXIS2_PLACEMENT_3D ( 'NONE', #39693, #36453, #31152 ) ;
#20378=PLANE ( 'NONE',  #38433 ) ;
#20380=ORIENTED_EDGE ( 'NONE', *, *, #23289, .T. ) ;
#20382=ORIENTED_EDGE ( 'NONE', *, *, #27929, .F. ) ;
#20385=CARTESIAN_POINT ( 'NONE',  ( -14.17145697063249088, 26.57885438195673444, 10.94387467463493735 ) ) ;
#20389=EDGE_CURVE ( 'NONE', #21146, #2261, #32107, .T. ) ;
#20395=CIRCLE ( 'NONE', #28180, 0.4999999999999986122 ) ;
#20401=ORIENTED_EDGE ( 'NONE', *, *, #10628, .F. ) ;
#20403=CARTESIAN_POINT ( 'NONE',  ( -8.412270287199723029, 10.07085245822962349, 10.49999999999999112 ) ) ;
#20405=ORIENTED_EDGE ( 'NONE', *, *, #10877, .F. ) ;
#20408=VECTOR ( 'NONE', #15063, 1000.000000000000000 ) ;
#20410=EDGE_LOOP ( 'NONE', ( #32444, #20260, #11998, #10700 ) ) ;
#20413=VECTOR ( 'NONE', #30273, 1000.000000000000114 ) ;
#20414=CARTESIAN_POINT ( 'NONE',  ( 14.70623423376107475, 19.54590544129782614, 7.000000000000000000 ) ) ;
#20417=CARTESIAN_POINT ( 'NONE',  ( -8.505700342264141511, 22.10876900990917804, 9.000000000000001776 ) ) ;
#20418=DIRECTION ( 'NONE',  ( 0.000000000000000000, 0.000000000000000000, 1.000000000000000000 ) ) ;
#20420=EDGE_LOOP ( 'NONE', ( #27913, #24348, #33180, #8639 ) ) ;
#20423=DIRECTION ( 'NONE',  ( 0.000000000000000000, 0.000000000000000000, 1.000000000000000000 ) ) ;
#20426=DIRECTION ( 'NONE',  ( 0.7032331762534049791, 0.07391278520355976100, -0.7071067811865475727 ) ) ;
#20428=DIRECTION ( 'NONE',  ( 0.1564344650402246795, -0.9876883405951386585, 0.000000000000000000 ) ) ;
#20429=ORIENTED_EDGE ( 'NONE', *, *, #29925, .T. ) ;
#20432=EDGE_CURVE ( 'NONE', #23885, #1824, #24371, .T. ) ;
#20434=CARTESIAN_POINT ( 'NONE',  ( -13.30736835487442349, 15.68301270189233954, 11.00000000000000000 ) ) ;
#20436=ORIENTED_EDGE ( 'NONE', *, *, #7533, .F. ) ;
#20437=CARTESIAN_POINT ( 'NONE',  ( -13.95683075005230123, 28.08631143191951551, 10.49999999999999822 ) ) ;
#20438=ORIENTED_EDGE ( 'NONE', *, *, #5751, .F. ) ;
#20440=DIRECTION ( 'NONE',  ( -0.000000000000000000, -0.000000000000000000, -1.000000000000000000 ) ) ;
#20443=AXIS2_PLACEMENT_3D ( 'NONE', #37958, #32680, #20280 ) ;
#20447=EDGE_CURVE ( 'NONE', #34816, #1059, #11282, .T. ) ;
#20448=ORIENTED_EDGE ( 'NONE', *, *, #25241, .F. ) ;
#20450=DIRECTION ( 'NONE',  ( 1.000000000000000000, 0.000000000000000000, 0.000000000000000000 ) ) ;
#20452=EDGE_CURVE ( 'NONE', #9748, #25178, #35764, .T. ) ;
#20453=DIRECTION ( 'NONE',  ( -0.000000000000000000, -0.000000000000000000, -1.000000000000000000 ) ) ;
#20454=AXIS2_PLACEMENT_3D ( 'NONE', #17186, #38500, #16777 ) ;
#20455=VERTEX_POINT ( 'NONE', #8527 ) ;
#20457=AXIS2_PLACEMENT_3D ( 'NONE', #7251, #29602, #35298 ) ;
#20461=DIRECTION ( 'NONE',  ( 0.000000000000000000, -0.5906904945688817854, 0.8068982213550663918 ) ) ;
#20465=ORIENTED_EDGE ( 'NONE', *, *, #32081, .T. ) ;
#20466=ADVANCED_FACE ( 'NONE', ( #4477, #20527 ), #20325, .T. ) ;
#20468=VECTOR ( 'NONE', #23176, 1000.000000000000227 ) ;
#20469=DIRECTION ( 'NONE',  ( 0.7431448254773863615, -0.6691306063588671194, 0.000000000000000000 ) ) ;
#20473=CARTESIAN_POINT ( 'NONE',  ( 0.5000000000000005551, 33.00000000000000000, 10.50000000000000000 ) ) ;
#20475=CARTESIAN_POINT ( 'NONE',  ( 1.000000000000000666, 32.50000000000000000, 10.50000000000000178 ) ) ;
#20477=CARTESIAN_POINT ( 'NONE',  ( 6.354454053420411697, 35.54304081427980577, 9.000000000000001776 ) ) ;
#20479=DIRECTION ( 'NONE',  ( -0.9510565162951507556, 0.3090169943749560000, 0.000000000000000000 ) ) ;
#20480=VECTOR ( 'NONE', #21406, 1000.000000000000114 ) ;
#20481=EDGE_LOOP ( 'NONE', ( #23990, #30826, #32496 ) ) ;
#20484=DIRECTION ( 'NONE',  ( 0.2185080122244080769, -0.6724985119639556030, -0.7071067811865499042 ) ) ;
#20485=CARTESIAN_POINT ( 'NONE',  ( -0.8223886111233146279, 37.39061994947693535, 10.49999999999999822 ) ) ;
#20487=DIRECTION ( 'NONE',  ( -0.000000000000000000, -0.000000000000000000, -1.000000000000000000 ) ) ;
#20489=CARTESIAN_POINT ( 'NONE',  ( -14.97277451176450924, 21.48159783397892397, 10.49999999999999822 ) ) ;
#20491=CARTESIAN_POINT ( 'NONE',  ( -13.53057405073934838, 22.08338764125509002, 10.50000000000000000 ) ) ;
#20497=ORIENTED_EDGE ( 'NONE', *, *, #31463, .T. ) ;
#20499=ORIENTED_EDGE ( 'NONE', *, *, #25393, .T. ) ;
#20500=CYLINDRICAL_SURFACE ( 'NONE', #28032, 0.4999999999999997780 ) ;
#20501=VERTEX_POINT ( 'NONE', #16882 ) ;
#20504=ORIENTED_EDGE ( 'NONE', *, *, #8115, .F. ) ;
#20505=AXIS2_PLACEMENT_3D ( 'NONE', #836, #10183, #31715 ) ;
#20507=ORIENTED_EDGE ( 'NONE', *, *, #33558, .T. ) ;
#20509=VECTOR ( 'NONE', #37950, 1000.000000000000000 ) ;
#20512=ORIENTED_EDGE ( 'NONE', *, *, #21052, .F. ) ;
#20515=EDGE_CURVE ( 'NONE', #39304, #2159, #23370, .T. ) ;
#20516=DIRECTION ( 'NONE',  ( 0.000000000000000000, 0.000000000000000000, 1.000000000000000000 ) ) ;
#20518=CARTESIAN_POINT ( 'NONE',  ( -5.440908595777636414, 35.94977745735568675, 9.000000000000001776 ) ) ;
#20519=VERTEX_POINT ( 'NONE', #5278 ) ;
#20527=FACE_BOUND ( 'NONE', #39172, .T. ) ;
#20530=AXIS2_PLACEMENT_3D ( 'NONE', #7528, #10993, #23579 ) ;
#20532=EDGE_CURVE ( 'NONE', #28626, #33852, #2042, .T. ) ;
#20537=EDGE_CURVE ( 'NONE', #19050, #10078, #35560, .T. ) ;
#20539=CARTESIAN_POINT ( 'NONE',  ( 14.09933648065468503, 26.02968990214155198, 9.500000000000000000 ) ) ;
#20540=ORIENTED_EDGE ( 'NONE', *, *, #34226, .T. ) ;
#20541=ORIENTED_EDGE ( 'NONE', *, *, #35490, .T. ) ;
#20543=DIRECTION ( 'NONE',  ( 0.8090169943749426773, -0.5877852522924797984, 0.000000000000000000 ) ) ;
#20544=LINE ( 'NONE', #18295, #5560 ) ;
#20545=ADVANCED_FACE ( 'NONE', ( #5081 ), #14018, .T. ) ;
#20547=CARTESIAN_POINT ( 'NONE',  ( -12.80736835487442349, 15.68301270189233954, 7.000000000000000000 ) ) ;
#20548=ORIENTED_EDGE ( 'NONE', *, *, #4738, .T. ) ;
#20550=FACE_OUTER_BOUND ( 'NONE', #24885, .T. ) ;
#20552=DIRECTION ( 'NONE',  ( 0.000000000000000000, 0.000000000000000000, 1.000000000000000000 ) ) ;
#20553=ORIENTED_EDGE ( 'NONE', *, *, #9753, .T. ) ;
#20555=PLANE ( 'NONE',  #17054 ) ;
#20556=ORIENTED_EDGE ( 'NONE', *, *, #36254, .T. ) ;
#20559=ORIENTED_EDGE ( 'NONE', *, *, #14664, .T. ) ;
#20563=ADVANCED_FACE ( 'NONE', ( #1843 ), #38940, .T. ) ;
#20564=DIRECTION ( 'NONE',  ( -0.6691306063588653430, -0.7431448254773878048, 0.000000000000000000 ) ) ;
#20565=EDGE_CURVE ( 'NONE', #31137, #21311, #32453, .T. ) ;
#20569=CARTESIAN_POINT ( 'NONE',  ( -3.607749162633401951, 7.931741834401822899, 10.63089969389957190 ) ) ;
#20572=CARTESIAN_POINT ( 'NONE',  ( -4.625823320348136036, 31.66047261929882950, 10.75000000000000888 ) ) ;
#20574=CARTESIAN_POINT ( 'NONE',  ( 8.118377661053324701, 10.47536095541698486, 7.000000000000000000 ) ) ;
#20577=LINE ( 'NONE', #32973, #4806 ) ;
#20578=CARTESIAN_POINT ( 'NONE',  ( -13.14565529531520127, 15.48770264576553402, 10.82238833324609750 ) ) ;
#20580=VERTEX_POINT ( 'NONE', #11179 ) ;
#20581=EDGE_CURVE ( 'NONE', #10337, #33798, #5181, .T. ) ;
#20583=EDGE_CURVE ( 'NONE', #37593, #10104, #35965, .T. ) ;
#20590=ORIENTED_EDGE ( 'NONE', *, *, #36600, .F. ) ;
#20592=ORIENTED_EDGE ( 'NONE', *, *, #25093, .T. ) ;
#20597=CONICAL_SURFACE ( 'NONE', #38082, 0.5000000000000002220, 0.7853981633974517207 ) ;
#20602=ORIENTED_EDGE ( 'NONE', *, *, #37982, .T. ) ;
#20604=CARTESIAN_POINT ( 'NONE',  ( -12.68475447279705115, 27.14725768220950286, 7.000000000000000000 ) ) ;
#20605=CARTESIAN_POINT ( 'NONE',  ( 6.557822374958316658, 35.99981354310111215, 7.000000000000000000 ) ) ;
#20606=CONICAL_SURFACE ( 'NONE', #25772, 0.4999999999999961142, 0.7853981633974463916 ) ;
#20610=AXIS2_PLACEMENT_3D ( 'NONE', #18028, #38952, #1990 ) ;
#20612=ORIENTED_EDGE ( 'NONE', *, *, #30393, .F. ) ;
#20615=EDGE_CURVE ( 'NONE', #36809, #22772, #15159, .T. ) ;
#20616=CARTESIAN_POINT ( 'NONE',  ( 14.78558495942256990, 19.97203773654679537, 7.338691926023217071 ) ) ;
#20619=AXIS2_PLACEMENT_3D ( 'NONE', #28127, #2751, #21830 ) ;
#20620=CARTESIAN_POINT ( 'NONE',  ( -1.974612014229268020, 7.629979921222117767, 7.203056206335834766 ) ) ;
#20621=DIRECTION ( 'NONE',  ( 0.000000000000000000, 0.000000000000000000, 1.000000000000000000 ) ) ;
#20622=CARTESIAN_POINT ( 'NONE',  ( 3.357189294653307954, 32.49896394832310165, 10.49999999999999467 ) ) ;
#20623=ORIENTED_EDGE ( 'NONE', *, *, #28381, .F. ) ;
#20625=FACE_OUTER_BOUND ( 'NONE', #23580, .T. ) ;
#20626=FACE_OUTER_BOUND ( 'NONE', #12962, .T. ) ;
#20629=CARTESIAN_POINT ( 'NONE',  ( -14.86556419889029890, 20.43481210330121556, 10.50000000000000000 ) ) ;
#20631=AXIS2_PLACEMENT_3D ( 'NONE', #22033, #28326, #22421 ) ;
#20637=CARTESIAN_POINT ( 'NONE',  ( 13.97557076678965693, 21.53386246193694475, 7.000000000000000000 ) ) ;
#20639=ORIENTED_EDGE ( 'NONE', *, *, #15796, .F. ) ;
#20640=FACE_OUTER_BOUND ( 'NONE', #11643, .T. ) ;
#20648=CARTESIAN_POINT ( 'NONE',  ( 5.305271391459043251, 36.43775379931900460, 10.49999999999999822 ) ) ;
#20650=ORIENTED_EDGE ( 'NONE', *, *, #5317, .F. ) ;
#20652=DIRECTION ( 'NONE',  ( -1.000000000000000000, 0.000000000000000000, 0.000000000000000000 ) ) ;
#20654=DIRECTION ( 'NONE',  ( 0.7275037805841029215, 0.3706816908109982767, 0.5773502691896289507 ) ) ;
#20655=VECTOR ( 'NONE', #34559, 1000.000000000000227 ) ;
#20656=ORIENTED_EDGE ( 'NONE', *, *, #15801, .T. ) ;
#20658=AXIS2_PLACEMENT_3D ( 'NONE', #25529, #37733, #37928 ) ;
#20660=VECTOR ( 'NONE', #12838, 1000.000000000000114 ) ;
#20661=DIRECTION ( 'NONE',  ( 1.000000000000000000, 0.000000000000000000, -0.000000000000000000 ) ) ;
#20664=AXIS2_PLACEMENT_3D ( 'NONE', #36447, #8005, #8613 ) ;
#20665=DIRECTION ( 'NONE',  ( 0.000000000000000000, -0.5778781230734075791, -0.8161230758121935658 ) ) ;
#20666=LINE ( 'NONE', #35897, #31695 ) ;
#20668=ADVANCED_FACE ( 'NONE', ( #39799 ), #5674, .T. ) ;
#20669=VERTEX_POINT ( 'NONE', #36560 ) ;
#20671=DIRECTION ( 'NONE',  ( -0.000000000000000000, 0.000000000000000000, 1.000000000000000000 ) ) ;
#20674=LINE ( 'NONE', #27159, #23695 ) ;
#20675=DIRECTION ( 'NONE',  ( 0.9781476007338070211, 0.2079116908177534029, -0.000000000000000000 ) ) ;
#20678=CARTESIAN_POINT ( 'NONE',  ( 5.440908595777819379, 35.94977745735560859, 11.00000000000000000 ) ) ;
#20679=CARTESIAN_POINT ( 'NONE',  ( -7.929471891321301591, 25.60217271033470610, 7.000000000000000000 ) ) ;
#20681=VECTOR ( 'NONE', #31465, 999.9999999999998863 ) ;
#20683=DIRECTION ( 'NONE',  ( -0.000000000000000000, -0.000000000000000000, -1.000000000000000000 ) ) ;
#20684=VECTOR ( 'NONE', #4631, 999.9999999999998863 ) ;
#20685=ORIENTED_EDGE ( 'NONE', *, *, #1717, .T. ) ;
#20688=CARTESIAN_POINT ( 'NONE',  ( -14.08246327825354349, 27.69965426814084353, 10.49999999999999822 ) ) ;
#20692=DIRECTION ( 'NONE',  ( -0.3090169943749448977, 0.9510565162951543083, 0.000000000000000000 ) ) ;
#20693=CARTESIAN_POINT ( 'NONE',  ( 5.440908595777814050, 35.94977745735560859, 7.000000000000000000 ) ) ;
#20700=EDGE_CURVE ( 'NONE', #38335, #26227, #8731, .T. ) ;
#20704=CARTESIAN_POINT ( 'NONE',  ( 5.267154670482129930, 36.54499619867781490, 7.382773698552470343 ) ) ;
#20705=ORIENTED_EDGE ( 'NONE', *, *, #9512, .F. ) ;
#20708=ORIENTED_EDGE ( 'NONE', *, *, #19233, .F. ) ;
#20710=EDGE_LOOP ( 'NONE', ( #35167, #22812, #13547, #30525 ) ) ;
#20712=CIRCLE ( 'NONE', #20063, 6.000000000000005329 ) ;
#20716=CARTESIAN_POINT ( 'NONE',  ( 13.60579549876902483, 27.97225316470530387, 10.49999999999999645 ) ) ;
#20717=ORIENTED_EDGE ( 'NONE', *, *, #29090, .T. ) ;
#20718=CIRCLE ( 'NONE', #31718, 0.4999999999999989453 ) ;
#20719=DIRECTION ( 'NONE',  ( 1.000000000000000000, 0.000000000000000000, 0.000000000000000000 ) ) ;
#20721=ADVANCED_FACE ( 'NONE', ( #30868 ), #27611, .T. ) ;
#20722=DIRECTION ( 'NONE',  ( 1.000000000000000000, 0.000000000000000000, 0.000000000000000000 ) ) ;
#20725=DIRECTION ( 'NONE',  ( 0.000000000000000000, 0.000000000000000000, 1.000000000000000000 ) ) ;
#20726=CARTESIAN_POINT ( 'NONE',  ( -8.927394655428429360, 11.06314620770957013, 7.000000000000000000 ) ) ;
#20728=LINE ( 'NONE', #30263, #5906 ) ;
#20733=CARTESIAN_POINT ( 'NONE',  ( 8.238488885696289898, 24.65111619403943877, 9.000000000000001776 ) ) ;
#20734=DIRECTION ( 'NONE',  ( -0.000000000000000000, -0.000000000000000000, -1.000000000000000000 ) ) ;
#20737=DIRECTION ( 'NONE',  ( -0.9510565162951543083, -0.3090169943749450088, -0.000000000000000000 ) ) ;
#20742=EDGE_CURVE ( 'NONE', #15678, #27267, #13355, .T. ) ;
#20743=CARTESIAN_POINT ( 'NONE',  ( 13.32679399471731685, 28.40733119287944319, 7.000000000000000000 ) ) ;
#20745=EDGE_LOOP ( 'NONE', ( #25782, #3656, #10894, #12274 ) ) ;
#20749=DIRECTION ( 'NONE',  ( 0.8090169943749426773, -0.5877852522924797984, 0.000000000000000000 ) ) ;
#20750=CARTESIAN_POINT ( 'NONE',  ( 9.892954722048896699, 20.95745441963929423, 10.50000000000000533 ) ) ;
#20752=EDGE_LOOP ( 'NONE', ( #16748, #12382, #5523, #36005 ) ) ;
#20755=CARTESIAN_POINT ( 'NONE',  ( -6.778507894852238813, 14.44616049828245785, 10.75000000000001066 ) ) ;
#20757=ORIENTED_EDGE ( 'NONE', *, *, #22458, .T. ) ;
#20759=CARTESIAN_POINT ( 'NONE',  ( 11.11016527260166420, 31.83082137946473367, 11.00000000000000000 ) ) ;
#20763=VERTEX_POINT ( 'NONE', #34912 ) ;
#20766=DIRECTION ( 'NONE',  ( 0.4067366430757889395, -0.9135454576426059736, 0.000000000000000000 ) ) ;
#20769=AXIS2_PLACEMENT_3D ( 'NONE', #26408, #4873, #29457 ) ;
#20771=ORIENTED_EDGE ( 'NONE', *, *, #31988, .F. ) ;
#20772=CARTESIAN_POINT ( 'NONE',  ( 14.70623423376107475, 19.54590544129782614, 7.000000000000000000 ) ) ;
#20773=CYLINDRICAL_SURFACE ( 'NONE', #32531, 0.5000000000000007772 ) ;
#20775=DIRECTION ( 'NONE',  ( -0.000000000000000000, -0.000000000000000000, 1.000000000000000000 ) ) ;
#20778=CARTESIAN_POINT ( 'NONE',  ( -4.524139159579191549, 31.43208625488816566, 10.50000000000000000 ) ) ;
#20779=DIRECTION ( 'NONE',  ( -0.9781476007338072431, -0.2079116908177518208, 0.000000000000000000 ) ) ;
#20780=LINE ( 'NONE', #2881, #1239 ) ;
#20783=ORIENTED_EDGE ( 'NONE', *, *, #34421, .F. ) ;
#20786=CARTESIAN_POINT ( 'NONE',  ( -14.26801110064877776, 26.12045026487111343, 10.49999999999999822 ) ) ;
#20788=ORIENTED_EDGE ( 'NONE', *, *, #28504, .F. ) ;
#20790=ORIENTED_EDGE ( 'NONE', *, *, #3908, .F. ) ;
#20792=CARTESIAN_POINT ( 'NONE',  ( -13.24038105676664401, 15.43301270189234486, 7.000000000000000000 ) ) ;
#20796=ORIENTED_EDGE ( 'NONE', *, *, #7684, .T. ) ;
#20800=EDGE_LOOP ( 'NONE', ( #39169, #11238, #10595 ) ) ;
#20802=DIRECTION ( 'NONE',  ( 1.000000000000000000, 0.000000000000000000, 0.000000000000000000 ) ) ;
#20804=ORIENTED_EDGE ( 'NONE', *, *, #19251, .F. ) ;
#20806=ORIENTED_EDGE ( 'NONE', *, *, #15873, .T. ) ;
#20809=ORIENTED_EDGE ( 'NONE', *, *, #3564, .T. ) ;
#20812=EDGE_CURVE ( 'NONE', #16261, #26640, #39325, .T. ) ;
#20813=CARTESIAN_POINT ( 'NONE',  ( -13.24038105676664401, 15.43301270189234486, 10.49999999999999822 ) ) ;
#20814=CIRCLE ( 'NONE', #21443, 0.5000000000000004441 ) ;
#20815=LINE ( 'NONE', #2126, #36258 ) ;
#20816=EDGE_CURVE ( 'NONE', #39980, #12345, #19461, .T. ) ;
#20819=CYLINDRICAL_SURFACE ( 'NONE', #32703, 0.5000000000000004441 ) ;
#20820=LINE ( 'NONE', #11672, #20480 ) ;
#20821=ORIENTED_EDGE ( 'NONE', *, *, #21798, .F. ) ;
#20824=DIRECTION ( 'NONE',  ( -0.8660254037844364872, 0.5000000000000038858, -0.000000000000000000 ) ) ;
#20826=AXIS2_PLACEMENT_3D ( 'NONE', #18273, #27208, #2233 ) ;
#20828=CARTESIAN_POINT ( 'NONE',  ( -14.55573640795744872, 20.46737631633130405, 10.96580508970282253 ) ) ;
#20831=ORIENTED_EDGE ( 'NONE', *, *, #33414, .F. ) ;
#20834=DIRECTION ( 'NONE',  ( -0.000000000000000000, -0.000000000000000000, -1.000000000000000000 ) ) ;
#20836=EDGE_LOOP ( 'NONE', ( #7694, #15032, #511, #25592 ) ) ;
#20837=CARTESIAN_POINT ( 'NONE',  ( -14.81003276707474292, 21.44615697153889755, 10.87262190629285108 ) ) ;
#20838=ORIENTED_EDGE ( 'NONE', *, *, #1445, .F. ) ;
#20841=ADVANCED_FACE ( 'NONE', ( #3825 ), #36746, .T. ) ;
#20844=EDGE_CURVE ( 'NONE', #26114, #7930, #22308, .T. ) ;
#20845=CIRCLE ( 'NONE', #23410, 1.000000000000002665 ) ;
#20848=DIRECTION ( 'NONE',  ( 1.000000000000000000, 0.000000000000000000, 0.000000000000000000 ) ) ;
#20850=EDGE_LOOP ( 'NONE', ( #10710, #39661, #26128, #38273 ) ) ;
#20853=CARTESIAN_POINT ( 'NONE',  ( -5.198706521309195416, 29.65540566576573767, 7.000000000000000000 ) ) ;
#20856=ORIENTED_EDGE ( 'NONE', *, *, #1717, .F. ) ;
#20859=DIRECTION ( 'NONE',  ( 0.000000000000000000, 0.000000000000000000, -1.000000000000000000 ) ) ;
#20863=EDGE_CURVE ( 'NONE', #5593, #12092, #5595, .T. ) ;
#20864=DIRECTION ( 'NONE',  ( -0.000000000000000000, -0.000000000000000000, -1.000000000000000000 ) ) ;
#20865=EDGE_CURVE ( 'NONE', #32523, #31286, #34766, .T. ) ;
#20873=FACE_OUTER_BOUND ( 'NONE', #38253, .T. ) ;
#20875=CARTESIAN_POINT ( 'NONE',  ( -13.32151712420406220, 20.09434385051854122, 10.50000000000000000 ) ) ;
#20876=LINE ( 'NONE', #26564, #26152 ) ;
#20877=CYLINDRICAL_SURFACE ( 'NONE', #19704, 0.5000000000000004441 ) ;
#20879=CARTESIAN_POINT ( 'NONE',  ( 9.421923923747751672, 10.82814555784876731, 7.455686640544903376 ) ) ;
#20882=DIRECTION ( 'NONE',  ( -0.3090169943749450643, 0.9510565162951544194, 0.000000000000000000 ) ) ;
#20883=LINE ( 'NONE', #30225, #8853 ) ;
#20884=AXIS2_PLACEMENT_3D ( 'NONE', #11400, #1861, #39221 ) ;
#20888=CARTESIAN_POINT ( 'NONE',  ( -14.97191702109866718, 21.44669161452688044, 10.49999999999999822 ) ) ;
#20894=CARTESIAN_POINT ( 'NONE',  ( 9.427394962683440127, 11.06314620782477753, 10.49999999999999822 ) ) ;
#20899=ORIENTED_EDGE ( 'NONE', *, *, #23335, .T. ) ;
#20900=FACE_OUTER_BOUND ( 'NONE', #23950, .T. ) ;
#20901=CARTESIAN_POINT ( 'NONE',  ( 9.359089477944728230, 11.31962006718884162, 10.49999999999999822 ) ) ;
#20905=CIRCLE ( 'NONE', #3378, 0.5000000000000024425 ) ;
#20906=CARTESIAN_POINT ( 'NONE',  ( 10.24940219216491677, 33.45281357907897046, 7.102637441331450141 ) ) ;
#20908=CARTESIAN_POINT ( 'NONE',  ( -8.007761790012255076, 9.776959832083379709, 10.50000000000000711 ) ) ;
#20909=CARTESIAN_POINT ( 'NONE',  ( 6.811226782241714517, 35.33967249274190436, 10.49999999999999822 ) ) ;
#20911=CARTESIAN_POINT ( 'NONE',  ( -4.003810537522578983, 8.420815593655365916, 10.49999999999999822 ) ) ;
#20913=CARTESIAN_POINT ( 'NONE',  ( -5.644276917315534270, 36.40655018617698602, 10.63089969389957190 ) ) ;
#20914=DIRECTION ( 'NONE',  ( 1.224646799147351235E-16, -1.000000000000000000, 0.000000000000000000 ) ) ;
#20916=CARTESIAN_POINT ( 'NONE',  ( -13.37378135583788463, 20.59160479820268108, 9.500000000000000000 ) ) ;
#20921=CARTESIAN_POINT ( 'NONE',  ( 10.81260707898150386, 32.90853150812154837, 10.63089969389957190 ) ) ;
#20922=VECTOR ( 'NONE', #16314, 1000.000000000000114 ) ;
#20931=VECTOR ( 'NONE', #209, 1000.000000000000114 ) ;
#20932=CARTESIAN_POINT ( 'NONE',  ( 11.11016527260166242, 31.83082137946473367, 10.99999999999999645 ) ) ;
#20933=ORIENTED_EDGE ( 'NONE', *, *, #10569, .F. ) ;
#20934=ORIENTED_EDGE ( 'NONE', *, *, #1413, .F. ) ;
#20936=CARTESIAN_POINT ( 'NONE',  ( -12.80736835487442349, 15.68301270189233954, 9.500000000000000000 ) ) ;
#20937=CARTESIAN_POINT ( 'NONE',  ( 10.36702044712426840, 31.16169077310587809, 10.50000000000000000 ) ) ;
#20938=AXIS2_PLACEMENT_3D ( 'NONE', #31526, #7130, #22771 ) ;
#20939=DIRECTION ( 'NONE',  ( -0.000000000000000000, -0.000000000000000000, -1.000000000000000000 ) ) ;
#20940=ORIENTED_EDGE ( 'NONE', *, *, #8002, .T. ) ;
#20942=ADVANCED_FACE ( 'NONE', ( #7677 ), #15846, .T. ) ;
#20943=DIRECTION ( 'NONE',  ( -0.9945218953682730678, 0.1045284632676569819, -0.000000000000000000 ) ) ;
#20944=CARTESIAN_POINT ( 'NONE',  ( -2.575189371470781197, 7.979819372998155913, 10.94387467463494090 ) ) ;
#20952=ORIENTED_EDGE ( 'NONE', *, *, #992, .F. ) ;
#20955=CARTESIAN_POINT ( 'NONE',  ( 15.00000000000000000, 22.50000000000000711, 7.000000000000000000 ) ) ;
#20957=AXIS2_PLACEMENT_3D ( 'NONE', #14315, #24063, #39698 ) ;
#20963=DIRECTION ( 'NONE',  ( 0.1045284632676570929, 0.9945218953682729568, 0.000000000000000000 ) ) ;
#20966=AXIS2_PLACEMENT_3D ( 'NONE', #19905, #17476, #32509 ) ;
#20973=VERTEX_POINT ( 'NONE', #17241 ) ;
#20974=AXIS2_PLACEMENT_3D ( 'NONE', #27558, #19011, #11924 ) ;
#20979=CARTESIAN_POINT ( 'NONE',  ( -3.998603647808162798, 8.333314792924266357, 10.49999999999999822 ) ) ;
#20981=VERTEX_POINT ( 'NONE', #5032 ) ;
#20987=ADVANCED_FACE ( 'NONE', ( #4832 ), #26765, .T. ) ;
#20988=LINE ( 'NONE', #9190, #25081 ) ;
#20989=AXIS2_PLACEMENT_3D ( 'NONE', #32051, #773, #31258 ) ;
#20990=ORIENTED_EDGE ( 'NONE', *, *, #10758, .F. ) ;
#20996=DIRECTION ( 'NONE',  ( -0.9510565162951503115, 0.3090169943749573322, 0.000000000000000000 ) ) ;
#21001=ORIENTED_EDGE ( 'NONE', *, *, #15553, .F. ) ;
#21003=AXIS2_PLACEMENT_3D ( 'NONE', #32659, #1167, #13954 ) ;
#21007=CARTESIAN_POINT ( 'NONE',  ( 11.11016527260166420, 31.83082137946473367, 7.000000000000000000 ) ) ;
#21015=DIRECTION ( 'NONE',  ( -0.8090169943749430104, 0.5877852522924791323, 0.000000000000000000 ) ) ;
#21016=ORIENTED_EDGE ( 'NONE', *, *, #39040, .F. ) ;
#21021=DIRECTION ( 'NONE',  ( 1.000000000000000000, 0.000000000000000000, 0.000000000000000000 ) ) ;
#21024=ORIENTED_EDGE ( 'NONE', *, *, #39842, .F. ) ;
#21025=VECTOR ( 'NONE', #12699, 1000.000000000000000 ) ;
#21028=CARTESIAN_POINT ( 'NONE',  ( 0.5000000000000002220, 36.50000000000000711, 9.500000000000000000 ) ) ;
#21031=CARTESIAN_POINT ( 'NONE',  ( -14.61656768153253694, 21.96308928146571660, 10.49999999999999822 ) ) ;
#21036=ADVANCED_FACE ( 'NONE', ( #23325 ), #608, .T. ) ;
#21037=CARTESIAN_POINT ( 'NONE',  ( 1.000000000000000000, 37.50000000000000711, 10.49999999999999822 ) ) ;
#21045=CARTESIAN_POINT ( 'NONE',  ( 9.665073660139013256, 25.11464168560187460, 10.50000000000000533 ) ) ;
#21046=DIRECTION ( 'NONE',  ( 0.000000000000000000, 0.000000000000000000, 1.000000000000000000 ) ) ;
#21047=DIRECTION ( 'NONE',  ( 0.000000000000000000, 0.000000000000000000, -1.000000000000000000 ) ) ;
#21052=EDGE_CURVE ( 'NONE', #18778, #25278, #2593, .T. ) ;
#21053=PLANE ( 'NONE',  #9214 ) ;
#21055=DIRECTION ( 'NONE',  ( 1.000000000000000000, 0.000000000000000000, 0.000000000000000000 ) ) ;
#21058=ORIENTED_EDGE ( 'NONE', *, *, #23443, .F. ) ;
#21059=EDGE_CURVE ( 'NONE', #38584, #19377, #21078, .T. ) ;
#21061=EDGE_CURVE ( 'NONE', #26362, #11564, #5437, .T. ) ;
#21063=DIRECTION ( 'NONE',  ( 0.2876062384759507928, 0.6459741880212497289, -0.7071067811865487940 ) ) ;
#21064=VERTEX_POINT ( 'NONE', #39952 ) ;
#21067=CARTESIAN_POINT ( 'NONE',  ( 19.73557158514996246, 33.31698729810761250, 11.00000000000000000 ) ) ;
#21069=CARTESIAN_POINT ( 'NONE',  ( 14.52509594610761923, 21.97885917798724975, 10.50000000000000355 ) ) ;
#21071=CARTESIAN_POINT ( 'NONE',  ( 14.22382948751891441, 26.07014013211499659, 10.49999999999999822 ) ) ;
#21077=DIRECTION ( 'NONE',  ( -0.2079116908177663647, -0.9781476007338042455, 0.000000000000000000 ) ) ;
#21078=LINE ( 'NONE', #24119, #7526 ) ;
#21086=AXIS2_PLACEMENT_3D ( 'NONE', #4622, #17020, #22695 ) ;
#21090=EDGE_CURVE ( 'NONE', #26812, #24016, #39754, .T. ) ;
#21092=DIRECTION ( 'NONE',  ( 1.000000000000000000, 0.000000000000000000, 0.000000000000000000 ) ) ;
#21097=DIRECTION ( 'NONE',  ( -0.9781476007338069101, -0.2079116908177532363, 0.000000000000000000 ) ) ;
#21102=ORIENTED_EDGE ( 'NONE', *, *, #16751, .T. ) ;
#21104=CARTESIAN_POINT ( 'NONE',  ( 10.16122020288883299, 33.53402030034401804, 7.000000000000000000 ) ) ;
#21106=CARTESIAN_POINT ( 'NONE',  ( -3.503793317224518145, 8.420815634768723967, 7.000000000000000000 ) ) ;
#21107=AXIS2_PLACEMENT_3D ( 'NONE', #32630, #38712, #23273 ) ;
#21109=CONICAL_SURFACE ( 'NONE', #10085, 1.000000000000002665, 0.7853981633974548293 ) ;
#21110=VECTOR ( 'NONE', #15237, 1000.000000000000000 ) ;
#21111=CARTESIAN_POINT ( 'NONE',  ( -3.718716484603639572, 7.955328666817546690, 10.49999999999999645 ) ) ;
#21114=CARTESIAN_POINT ( 'NONE',  ( 3.357189294653307954, 32.49896394832310165, 10.49999999999999645 ) ) ;
#21115=DIRECTION ( 'NONE',  ( 1.000000000000000000, 0.000000000000000000, 0.000000000000000000 ) ) ;
#21119=ORIENTED_EDGE ( 'NONE', *, *, #28494, .T. ) ;
#21122=DIRECTION ( 'NONE',  ( -0.5877852522924797984, -0.8090169943749426773, 0.000000000000000000 ) ) ;
#21124=DIRECTION ( 'NONE',  ( 0.000000000000000000, 0.000000000000000000, 1.000000000000000000 ) ) ;
#21130=VERTEX_POINT ( 'NONE', #6227 ) ;
#21131=ORIENTED_EDGE ( 'NONE', *, *, #37609, .F. ) ;
#21135=CARTESIAN_POINT ( 'NONE',  ( 12.80736835487433289, 15.68301270189216545, 7.499999999999997335 ) ) ;
#21136=VECTOR ( 'NONE', #4568, 999.9999999999998863 ) ;
#21137=AXIS2_PLACEMENT_3D ( 'NONE', #2598, #36124, #33087 ) ;
#21138=CARTESIAN_POINT ( 'NONE',  ( -12.99377146717201192, 26.19620116591435277, 10.00000000000000000 ) ) ;
#21142=CARTESIAN_POINT ( 'NONE',  ( -2.596139932171949383, 7.881254734312912902, 10.87262190629277292 ) ) ;
#21143=VERTEX_POINT ( 'NONE', #31019 ) ;
#21145=CYLINDRICAL_SURFACE ( 'NONE', #39743, 0.5000000000000004441 ) ;
#21146=VERTEX_POINT ( 'NONE', #37113 ) ;
#21149=ORIENTED_EDGE ( 'NONE', *, *, #5808, .T. ) ;
#21155=ORIENTED_EDGE ( 'NONE', *, *, #40024, .F. ) ;
#21157=CARTESIAN_POINT ( 'NONE',  ( 10.72501808743029095, 33.00580893829960161, 10.49999999999999822 ) ) ;
#21158=DIRECTION ( 'NONE',  ( 0.000000000000000000, 0.000000000000000000, -1.000000000000000000 ) ) ;
#21159=VECTOR ( 'NONE', #17699, 1000.000000000000227 ) ;
#21165=AXIS2_PLACEMENT_3D ( 'NONE', #27172, #6025, #33286 ) ;
#21168=CARTESIAN_POINT ( 'NONE',  ( 8.843266739736572291, 16.81698729810774395, 10.50000000000000000 ) ) ;
#21169=DIRECTION ( 'NONE',  ( -0.9510565162951504226, 0.3090169943749573322, 0.000000000000000000 ) ) ;
#21170=LINE ( 'NONE', #2288, #21996 ) ;
#21173=ORIENTED_EDGE ( 'NONE', *, *, #17972, .T. ) ;
#21177=CARTESIAN_POINT ( 'NONE',  ( 3.963760424820348405, 8.194319839800193961, 10.49999999999999822 ) ) ;
#21179=VERTEX_POINT ( 'NONE', #12326 ) ;
#21181=VERTEX_POINT ( 'NONE', #9281 ) ;
#21183=CARTESIAN_POINT ( 'NONE',  ( -6.774334011769939323, 35.84443018111166879, 10.49999999999999467 ) ) ;
#21185=CARTESIAN_POINT ( 'NONE',  ( -13.30736835487441638, 16.54903810567678235, 7.000000000000000000 ) ) ;
#21189=CARTESIAN_POINT ( 'NONE',  ( 14.52509594610761923, 21.97885917798724975, 7.000000000000000000 ) ) ;
#21190=VERTEX_POINT ( 'NONE', #23923 ) ;
#21192=CARTESIAN_POINT ( 'NONE',  ( 9.197066986886593298, 11.25907462514027202, 10.66666666666666430 ) ) ;
#21193=EDGE_CURVE ( 'NONE', #30652, #12596, #12720, .T. ) ;
#21195=EDGE_CURVE ( 'NONE', #31103, #22349, #1721, .T. ) ;
#21198=ORIENTED_EDGE ( 'NONE', *, *, #26662, .T. ) ;
#21201=ORIENTED_EDGE ( 'NONE', *, *, #14822, .T. ) ;
#21203=DIRECTION ( 'NONE',  ( -2.168404344971006896E-16, 1.000000000000000000, 0.000000000000000000 ) ) ;
#21205=PLANE ( 'NONE',  #38187 ) ;
#21206=DIRECTION ( 'NONE',  ( 0.4156269377774484686, -0.5720614028176835841, -0.7071067811865511255 ) ) ;
#21207=EDGE_CURVE ( 'NONE', #12323, #2692, #20883, .T. ) ;
#21209=DIRECTION ( 'NONE',  ( 0.4731467892558125499, -0.5254827454987578417, -0.7071067811865499042 ) ) ;
#21210=ORIENTED_EDGE ( 'NONE', *, *, #18987, .F. ) ;
#21212=LINE ( 'NONE', #4772, #15101 ) ;
#21215=DIRECTION ( 'NONE',  ( -1.000000000000000000, 0.000000000000000000, 0.000000000000000000 ) ) ;
#21217=VECTOR ( 'NONE', #34328, 1000.000000000000000 ) ;
#21219=EDGE_LOOP ( 'NONE', ( #2310, #26884, #8201 ) ) ;
#21221=CIRCLE ( 'NONE', #25735, 15.00000000000000000 ) ;
#21223=CARTESIAN_POINT ( 'NONE',  ( -6.354454053420243831, 35.54304081427989814, 11.00000000000000000 ) ) ;
#21226=CARTESIAN_POINT ( 'NONE',  ( -14.70981814587872094, 21.45668995266216683, 10.94387467463488051 ) ) ;
#21227=ORIENTED_EDGE ( 'NONE', *, *, #905, .T. ) ;
#21229=DIRECTION ( 'NONE',  ( 0.6691306063588571273, -0.7431448254773952433, 0.000000000000000000 ) ) ;
#21235=DIRECTION ( 'NONE',  ( -1.000000000000000000, 0.000000000000000000, 0.000000000000000000 ) ) ;
#21239=CARTESIAN_POINT ( 'NONE',  ( -5.237540274239744775, 35.49300472853438038, 7.500000000000000888 ) ) ;
#21240=ADVANCED_FACE ( 'NONE', ( #33486 ), #18435, .T. ) ;
#21242=EDGE_CURVE ( 'NONE', #16160, #21540, #22253, .T. ) ;
#21243=LINE ( 'NONE', #34236, #11553 ) ;
#21244=VERTEX_POINT ( 'NONE', #31409 ) ;
#21250=CYLINDRICAL_SURFACE ( 'NONE', #13471, 0.5000000000000004441 ) ;
#21252=AXIS2_PLACEMENT_3D ( 'NONE', #32487, #16434, #22922 ) ;
#21254=CARTESIAN_POINT ( 'NONE',  ( 14.97837590057439527, 21.69185896976586037, 7.455686640544910482 ) ) ;
#21255=CIRCLE ( 'NONE', #3725, 0.5000000000000001110 ) ;
#21257=AXIS2_PLACEMENT_3D ( 'NONE', #14751, #10698, #4602 ) ;
#21258=FACE_OUTER_BOUND ( 'NONE', #12679, .T. ) ;
#21259=CARTESIAN_POINT ( 'NONE',  ( 1.000000000000000666, 33.00000000000000000, 11.00000000000000000 ) ) ;
#21261=DIRECTION ( 'NONE',  ( 0.2079116908177533751, -0.9781476007338067991, 0.000000000000000000 ) ) ;
#21263=LINE ( 'NONE', #12120, #21997 ) ;
#21264=LINE ( 'NONE', #32416, #5016 ) ;
#21265=FACE_OUTER_BOUND ( 'NONE', #3350, .T. ) ;
#21268=CARTESIAN_POINT ( 'NONE',  ( 9.729305141884044161, 11.08259174741900033, 7.203056206335836542 ) ) ;
#21269=ORIENTED_EDGE ( 'NONE', *, *, #8283, .T. ) ;
#21272=CARTESIAN_POINT ( 'NONE',  ( 9.356056665764066693, 26.06569820189703179, 10.49999999999999645 ) ) ;
#21277=VECTOR ( 'NONE', #34365, 1000.000000000000000 ) ;
#21279=PLANE ( 'NONE',  #21137 ) ;
#21282=AXIS2_PLACEMENT_3D ( 'NONE', #17613, #11307, #5800 ) ;
#21289=VECTOR ( 'NONE', #18756, 1000.000000000000000 ) ;
#21290=EDGE_CURVE ( 'NONE', #13694, #3751, #3577, .T. ) ;
#21293=EDGE_CURVE ( 'NONE', #13267, #16446, #32584, .T. ) ;
#21297=CARTESIAN_POINT ( 'NONE',  ( 12.62435565298211593, 16.36602540378438420, 9.500000000000000000 ) ) ;
#21298=DIRECTION ( 'NONE',  ( 0.9945218953682729568, -0.1045284632676570929, -0.000000000000000000 ) ) ;
#21302=DIRECTION ( 'NONE',  ( -0.1045284632676437564, 0.9945218953682744001, 0.000000000000000000 ) ) ;
#21303=ORIENTED_EDGE ( 'NONE', *, *, #14228, .F. ) ;
#21305=DIRECTION ( 'NONE',  ( 0.3090169943749448977, -0.9510565162951543083, 0.000000000000000000 ) ) ;
#21307=ADVANCED_FACE ( 'NONE', ( #38099 ), #19613, .F. ) ;
#21309=VECTOR ( 'NONE', #7591, 999.9999999999998863 ) ;
#21311=VERTEX_POINT ( 'NONE', #15973 ) ;
#21312=ADVANCED_FACE ( 'NONE', ( #9484 ), #6421, .F. ) ;
#21314=CARTESIAN_POINT ( 'NONE',  ( -5.622359283595719681, 36.35732237484531026, 10.76099332938163755 ) ) ;
#21315=DIRECTION ( 'NONE',  ( 0.3090169943749450643, -0.9510565162951544194, 0.000000000000000000 ) ) ;
#21316=CIRCLE ( 'NONE', #14178, 0.4999999999999997780 ) ;
#21324=DIRECTION ( 'NONE',  ( -1.000000000000000000, 0.000000000000000000, 0.000000000000000000 ) ) ;
#21326=LINE ( 'NONE', #5878, #310 ) ;
#21331=CARTESIAN_POINT ( 'NONE',  ( 11.14453731054108765, 31.86177010143591204, 10.99999999999999645 ) ) ;
#21332=ORIENTED_EDGE ( 'NONE', *, *, #20863, .F. ) ;
#21333=ORIENTED_EDGE ( 'NONE', *, *, #11260, .F. ) ;
#21335=EDGE_CURVE ( 'NONE', #35565, #23735, #15770, .T. ) ;
#21336=CARTESIAN_POINT ( 'NONE',  ( -14.31603901957233660, 19.98981538725089990, 10.49999999999999467 ) ) ;
#21340=CIRCLE ( 'NONE', #37547, 0.4999999999999997780 ) ;
#21341=CARTESIAN_POINT ( 'NONE',  ( 10.49474413300069386, 21.89971208337373909, 10.50000000000000000 ) ) ;
#21342=EDGE_LOOP ( 'NONE', ( #13622, #8988, #24537, #11856 ) ) ;
#21344=LINE ( 'NONE', #5492, #39471 ) ;
#21347=ORIENTED_EDGE ( 'NONE', *, *, #14771, .F. ) ;
#21352=ORIENTED_EDGE ( 'NONE', *, *, #10340, .T. ) ;
#21355=CARTESIAN_POINT ( 'NONE',  ( 9.331903152615748098, 11.35703883385568780, 10.49999999999999822 ) ) ;
#21357=CARTESIAN_POINT ( 'NONE',  ( -3.558056881628413937, 8.165525635826545781, 10.94611345180491035 ) ) ;
#21358=ORIENTED_EDGE ( 'NONE', *, *, #32736, .T. ) ;
#21359=ADVANCED_FACE ( 'NONE', ( #19824 ), #32423, .T. ) ;
#21360=CARTESIAN_POINT ( 'NONE',  ( 10.33648234394583376, 33.08013173297155873, 10.49999999999999822 ) ) ;
#21361=DIRECTION ( 'NONE',  ( -0.3090169943749573878, -0.9510565162951503115, 0.000000000000000000 ) ) ;
#21364=CIRCLE ( 'NONE', #9683, 1.000000000000000888 ) ;
#21365=FACE_OUTER_BOUND ( 'NONE', #4195, .T. ) ;
#21367=CARTESIAN_POINT ( 'NONE',  ( -9.844611323930809732, 11.18224604797046773, 7.076227724509050354 ) ) ;
#21368=VECTOR ( 'NONE', #34545, 1000.000000000000000 ) ;
#21369=DIRECTION ( 'NONE',  ( 0.000000000000000000, 0.000000000000000000, 1.000000000000000000 ) ) ;
#21371=VERTEX_POINT ( 'NONE', #7414 ) ;
#21375=CARTESIAN_POINT ( 'NONE',  ( 1.525645716490520387, 8.212903943950921715, 7.000000000000000000 ) ) ;
#21376=ORIENTED_EDGE ( 'NONE', *, *, #19085, .F. ) ;
#21381=CARTESIAN_POINT ( 'NONE',  ( 14.58123527826104215, 20.01612550765316101, 10.49999999999999467 ) ) ;
#21382=VERTEX_POINT ( 'NONE', #17395 ) ;
#21388=DIRECTION ( 'NONE',  ( 0.000000000000000000, 0.000000000000000000, -1.000000000000000000 ) ) ;
#21389=LINE ( 'NONE', #24634, #21878 ) ;
#21391=ORIENTED_EDGE ( 'NONE', *, *, #14263, .T. ) ;
#21393=ORIENTED_EDGE ( 'NONE', *, *, #29900, .T. ) ;
#21396=CARTESIAN_POINT ( 'NONE',  ( -1.590043107810763079, 12.61456814725308107, 10.50000000000000000 ) ) ;
#21398=EDGE_LOOP ( 'NONE', ( #18072, #3016, #38510 ) ) ;
#21400=CIRCLE ( 'NONE', #39581, 15.00000000000000000 ) ;
#21401=LINE ( 'NONE', #36840, #14201 ) ;
#21404=DIRECTION ( 'NONE',  ( 0.000000000000000000, 0.000000000000000000, 1.000000000000000000 ) ) ;
#21406=DIRECTION ( 'NONE',  ( 0.3090169943749448977, -0.9510565162951543083, 0.000000000000000000 ) ) ;
#21407=ORIENTED_EDGE ( 'NONE', *, *, #14496, .F. ) ;
#21409=CARTESIAN_POINT ( 'NONE',  ( 0.000000000000000000, 22.50000000000000355, 7.000000000000000000 ) ) ;
#21413=DIRECTION ( 'NONE',  ( -0.9781476007338041345, 0.2079116908177663092, 0.000000000000000000 ) ) ;
#21416=ORIENTED_EDGE ( 'NONE', *, *, #25775, .T. ) ;
#21419=CARTESIAN_POINT ( 'NONE',  ( -7.014595103779441843, 35.79644522156330311, 7.000000000000000000 ) ) ;
#21421=VERTEX_POINT ( 'NONE', #30586 ) ;
#21426=CARTESIAN_POINT ( 'NONE',  ( -1.838889047819898037, 31.15129278236396360, 9.000000000000001776 ) ) ;
#21428=DIRECTION ( 'NONE',  ( 0.4067366430757888840, -0.9135454576426058626, 0.000000000000000000 ) ) ;
#21431=CARTESIAN_POINT ( 'NONE',  ( 1.449462053036050024, 12.07351642418171167, 10.74999999999999112 ) ) ;
#21433=VERTEX_POINT ( 'NONE', #11495 ) ;
#21436=DIRECTION ( 'NONE',  ( 1.000000000000000000, 0.000000000000000000, 0.000000000000000000 ) ) ;
#21437=DIRECTION ( 'NONE',  ( 0.000000000000000000, 0.000000000000000000, 1.000000000000000000 ) ) ;
#21443=AXIS2_PLACEMENT_3D ( 'NONE', #30950, #30154, #21599 ) ;
#21444=EDGE_CURVE ( 'NONE', #29636, #31286, #18194, .T. ) ;
#21446=VERTEX_POINT ( 'NONE', #27327 ) ;
#21447=EDGE_CURVE ( 'NONE', #1824, #26924, #5392, .T. ) ;
#21450=ORIENTED_EDGE ( 'NONE', *, *, #28531, .F. ) ;
#21453=CARTESIAN_POINT ( 'NONE',  ( 12.89070168820767037, 15.82735026918957111, 10.83333333333333037 ) ) ;
#21455=CARTESIAN_POINT ( 'NONE',  ( -5.362728154696096539, 13.41753630677062148, 10.50000000000000711 ) ) ;
#21456=EDGE_CURVE ( 'NONE', #31127, #15571, #19467, .T. ) ;
#21457=CARTESIAN_POINT ( 'NONE',  ( 14.36830325120613061, 20.48707633493483371, 10.99999999999999289 ) ) ;
#21459=DIRECTION ( 'NONE',  ( 0.000000000000000000, 0.000000000000000000, -1.000000000000000000 ) ) ;
#21460=DIRECTION ( 'NONE',  ( 0.9135454576425988682, -0.4067366430758048157, 0.000000000000000000 ) ) ;
#21461=DIRECTION ( 'NONE',  ( -0.4999999999999920619, 0.8660254037844432595, 0.000000000000000000 ) ) ;
#21464=LINE ( 'NONE', #27362, #22425 ) ;
#21467=DIRECTION ( 'NONE',  ( -0.000000000000000000, -0.000000000000000000, -1.000000000000000000 ) ) ;
#21469=AXIS2_PLACEMENT_3D ( 'NONE', #8065, #36111, #8269 ) ;
#21474=ORIENTED_EDGE ( 'NONE', *, *, #2099, .T. ) ;
#21475=CARTESIAN_POINT ( 'NONE',  ( -2.525645716490710679, 8.212903943950959018, 9.000000000000001776 ) ) ;
#21482=DIRECTION ( 'NONE',  ( 0.8660254037844363761, -0.5000000000000039968, 0.000000000000000000 ) ) ;
#21483=AXIS2_PLACEMENT_3D ( 'NONE', #36552, #8114, #5272 ) ;
#21487=EDGE_CURVE ( 'NONE', #20155, #26406, #5869, .T. ) ;
#21489=ORIENTED_EDGE ( 'NONE', *, *, #9769, .T. ) ;
#21490=PLANE ( 'NONE',  #1874 ) ;
#21495=VECTOR ( 'NONE', #16507, 1000.000000000000227 ) ;
#21496=ORIENTED_EDGE ( 'NONE', *, *, #35310, .F. ) ;
#21497=DIRECTION ( 'NONE',  ( -1.000000000000000000, 0.000000000000000000, 0.000000000000000000 ) ) ;
#21498=VERTEX_POINT ( 'NONE', #12285 ) ;
#21501=CYLINDRICAL_SURFACE ( 'NONE', #13618, 0.4999999999999997780 ) ;
#21502=ORIENTED_EDGE ( 'NONE', *, *, #38386, .F. ) ;
#21504=FACE_OUTER_BOUND ( 'NONE', #10744, .T. ) ;
#21505=DIRECTION ( 'NONE',  ( -1.000000000000000000, 0.000000000000000000, 0.000000000000000000 ) ) ;
#21506=CIRCLE ( 'NONE', #24752, 1.000000000000000222 ) ;
#21507=EDGE_CURVE ( 'NONE', #21421, #14341, #14740, .T. ) ;
#21508=PLANE ( 'NONE',  #37689 ) ;
#21510=EDGE_CURVE ( 'NONE', #13434, #3501, #37402, .T. ) ;
#21517=DIRECTION ( 'NONE',  ( 0.9135454576426059736, 0.4067366430757888285, 0.000000000000000000 ) ) ;
#21520=VECTOR ( 'NONE', #6652, 1000.000000000000000 ) ;
#21524=DIRECTION ( 'NONE',  ( -0.000000000000000000, -0.000000000000000000, -1.000000000000000000 ) ) ;
#21525=ORIENTED_EDGE ( 'NONE', *, *, #23711, .F. ) ;
#21527=CARTESIAN_POINT ( 'NONE',  ( 0.5000000000000000000, 37.50000000000000711, 10.49999999999999822 ) ) ;
#21529=DIRECTION ( 'NONE',  ( -1.000000000000000000, 0.000000000000000000, 0.000000000000000000 ) ) ;
#21530=CARTESIAN_POINT ( 'NONE',  ( 13.63581098909226874, 27.45627467658428955, 7.000000000000000000 ) ) ;
#21531=VERTEX_POINT ( 'NONE', #24475 ) ;
#21533=EDGE_CURVE ( 'NONE', #13142, #32713, #36872, .T. ) ;
#21534=DIRECTION ( 'NONE',  ( 0.000000000000000000, 0.000000000000000000, 1.000000000000000000 ) ) ;
#21535=AXIS2_PLACEMENT_3D ( 'NONE', #8460, #24296, #12104 ) ;
#21536=CARTESIAN_POINT ( 'NONE',  ( 15.02235689379175732, 21.92659494635341844, 11.00000000000000000 ) ) ;
#21539=CARTESIAN_POINT ( 'NONE',  ( 9.677076426724161351, 26.69573495723207301, 10.50000000000000355 ) ) ;
#21540=VERTEX_POINT ( 'NONE', #5982 ) ;
#21542=EDGE_CURVE ( 'NONE', #39554, #2993, #24675, .T. ) ;
#21543=ORIENTED_EDGE ( 'NONE', *, *, #30399, .F. ) ;
#21546=CARTESIAN_POINT ( 'NONE',  ( -1.281338032051963616, 37.44565299484865051, 7.102637441331450141 ) ) ;
#21548=CARTESIAN_POINT ( 'NONE',  ( -11.81630298851966288, 31.79381426990562787, 7.000000000000000000 ) ) ;
#21549=ORIENTED_EDGE ( 'NONE', *, *, #38895, .F. ) ;
#21551=DIRECTION ( 'NONE',  ( 0.000000000000000000, 0.000000000000000000, 1.000000000000000000 ) ) ;
#21552=CARTESIAN_POINT ( 'NONE',  ( -10.32951289851619592, 32.69782367585516170, 10.83333333333333037 ) ) ;
#21553=LINE ( 'NONE', #17924, #2025 ) ;
#21555=EDGE_CURVE ( 'NONE', #11050, #39108, #37068, .T. ) ;
#21556=DIRECTION ( 'NONE',  ( 0.5000000000000039968, 0.8660254037844363761, 0.000000000000000000 ) ) ;
#21559=CARTESIAN_POINT ( 'NONE',  ( 8.401171878996485987, 21.11424711454080594, 7.000000000000000000 ) ) ;
#21560=VECTOR ( 'NONE', #12795, 1000.000000000000114 ) ;
#21563=CARTESIAN_POINT ( 'NONE',  ( -8.505700342264141511, 22.10876900990917804, 9.000000000000001776 ) ) ;
#21564=PLANE ( 'NONE',  #29135 ) ;
#21565=ORIENTED_EDGE ( 'NONE', *, *, #12037, .T. ) ;
#21567=CIRCLE ( 'NONE', #5997, 0.5000000000000004441 ) ;
#21570=CARTESIAN_POINT ( 'NONE',  ( -14.36910708881314669, 26.64307479831630587, 10.76099332938163577 ) ) ;
#21572=ORIENTED_EDGE ( 'NONE', *, *, #28354, .T. ) ;
#21577=ORIENTED_EDGE ( 'NONE', *, *, #26621, .F. ) ;
#21580=CARTESIAN_POINT ( 'NONE',  ( 0.5000000000000000000, 37.50000000000000711, 10.63089969389957190 ) ) ;
#21583=ADVANCED_FACE ( 'NONE', ( #37665 ), #19170, .F. ) ;
#21584=CARTESIAN_POINT ( 'NONE',  ( 8.927394655428267711, 11.06314620770944757, 11.00000000000000000 ) ) ;
#21585=ORIENTED_EDGE ( 'NONE', *, *, #37178, .T. ) ;
#21592=EDGE_LOOP ( 'NONE', ( #1301, #12991, #15993 ) ) ;
#21593=AXIS2_PLACEMENT_3D ( 'NONE', #19568, #13672, #6960 ) ;
#21595=CARTESIAN_POINT ( 'NONE',  ( -11.08846162081388975, 2.083081287325696529, 10.00000000000000000 ) ) ;
#21597=CIRCLE ( 'NONE', #37804, 0.5000000000000004441 ) ;
#21599=DIRECTION ( 'NONE',  ( 1.000000000000000000, 0.000000000000000000, 0.000000000000000000 ) ) ;
#21605=DIRECTION ( 'NONE',  ( 0.1045284632676570929, 0.9945218953682730678, 0.000000000000000000 ) ) ;
#21608=CARTESIAN_POINT ( 'NONE',  ( -13.28401428800407658, 15.85743772853297884, 10.49999999999999822 ) ) ;
#21610=VECTOR ( 'NONE', #13155, 999.9999999999998863 ) ;
#21611=VERTEX_POINT ( 'NONE', #6377 ) ;
#21617=VERTEX_POINT ( 'NONE', #12479 ) ;
#21621=CARTESIAN_POINT ( 'NONE',  ( 9.625795778761983001, 10.95253033666821274, 11.00000000000000000 ) ) ;
#21623=CARTESIAN_POINT ( 'NONE',  ( -14.06524961900331760, 27.71236540882611621, 7.499999999999993783 ) ) ;
#21624=AXIS2_PLACEMENT_3D ( 'NONE', #35856, #2338, #14116 ) ;
#21625=ORIENTED_EDGE ( 'NONE', *, *, #17618, .F. ) ;
#21628=LINE ( 'NONE', #15540, #20275 ) ;
#21630=ORIENTED_EDGE ( 'NONE', *, *, #30691, .T. ) ;
#21634=CARTESIAN_POINT ( 'NONE',  ( -0.5000000000000005551, 32.50000000000000000, 10.49999999999999645 ) ) ;
#21635=ORIENTED_EDGE ( 'NONE', *, *, #37430, .T. ) ;
#21639=CARTESIAN_POINT ( 'NONE',  ( -5.632984386902246676, 36.38118674759818560, 10.68306085400122996 ) ) ;
#21640=CIRCLE ( 'NONE', #26189, 1.000000000000000222 ) ;
#21644=VECTOR ( 'NONE', #5621, 1000.000000000000000 ) ;
#21645=CARTESIAN_POINT ( 'NONE',  ( -1.693998953219649772, 12.12549434688617822, 10.00000000000000000 ) ) ;
#21646=VERTEX_POINT ( 'NONE', #96 ) ;
#21647=CARTESIAN_POINT ( 'NONE',  ( 5.237540274239914417, 35.49300472853430222, 7.000000000000000000 ) ) ;
#21648=CARTESIAN_POINT ( 'NONE',  ( 11.14717238216093520, 32.53695909538286202, 7.000000000000000000 ) ) ;
#21651=CARTESIAN_POINT ( 'NONE',  ( -14.52509594610762456, 21.97885917798744870, 11.00000000000000000 ) ) ;
#21652=EDGE_CURVE ( 'NONE', #18499, #31487, #28323, .T. ) ;
#21653=DIRECTION ( 'NONE',  ( 0.8090169943749426773, -0.5877852522924797984, 0.000000000000000000 ) ) ;
#21654=CARTESIAN_POINT ( 'NONE',  ( 7.530592408760855783, 11.28437794979193498, 10.00000000000000000 ) ) ;
#21655=CARTESIAN_POINT ( 'NONE',  ( 4.481940917958135095, 8.628727325586426744, 7.000000000000000000 ) ) ;
#21656=LINE ( 'NONE', #34059, #39127 ) ;
#21659=DIRECTION ( 'NONE',  ( 0.000000000000000000, 0.000000000000000000, 1.000000000000000000 ) ) ;
#21662=CARTESIAN_POINT ( 'NONE',  ( 12.05736835487432579, 14.38397459621550567, 10.49999999999999822 ) ) ;
#21663=VECTOR ( 'NONE', #11073, 1000.000000000000000 ) ;
#21664=EDGE_CURVE ( 'NONE', #18489, #30503, #10230, .T. ) ;
#21671=B_SPLINE_SURFACE_WITH_KNOTS ( 'NONE', 1, 3, ( 
 ( #33339, #30075, #8740, #39809, #5683, #37168, #30280, #8942, #3041, #5288 ),
 ( #24577, #12184, #9342, #36972, #2248, #33927, #9139, #6082, #21331, #20932 ) ),
 .UNSPECIFIED., .F., .F., .F.,
 ( 2, 2 ),
 ( 4, 2, 2, 2, 4 ),
 ( 0.000000000000000000, 1.000000000000000000 ),
 ( 1.003840680322689360, 1.396539762021415498, 1.789238843720141414, 2.181937925418867330, 2.574637007117593246 ),
 .UNSPECIFIED. ) ;
#21672=ORIENTED_EDGE ( 'NONE', *, *, #23020, .F. ) ;
#21673=CARTESIAN_POINT ( 'NONE',  ( 0.5000000000000005551, 33.00000000000000000, 10.00000000000000000 ) ) ;
#21680=AXIS2_PLACEMENT_3D ( 'NONE', #3122, #18369, #34010 ) ;
#21682=DIRECTION ( 'NONE',  ( -0.6293203910498342823, 0.7771459614569734553, 0.000000000000000000 ) ) ;
#21684=ORIENTED_EDGE ( 'NONE', *, *, #9116, .F. ) ;
#21686=AXIS2_PLACEMENT_3D ( 'NONE', #1571, #4817, #32041 ) ;
#21689=CARTESIAN_POINT ( 'NONE',  ( -3.610593701936585465, 31.83882289796395426, 10.00000000000000000 ) ) ;
#21690=EDGE_CURVE ( 'NONE', #31599, #2452, #4226, .T. ) ;
#21699=DIRECTION ( 'NONE',  ( -1.224646799147351235E-16, 1.000000000000000000, 0.000000000000000000 ) ) ;
#21700=PLANE ( 'NONE',  #25319 ) ;
#21701=AXIS2_PLACEMENT_3D ( 'NONE', #14831, #27218, #39804 ) ;
#21702=FACE_OUTER_BOUND ( 'NONE', #13792, .T. ) ;
#21703=ORIENTED_EDGE ( 'NONE', *, *, #21664, .F. ) ;
#21705=DIRECTION ( 'NONE',  ( 0.9510565162951541973, 0.3090169943749456194, 0.000000000000000000 ) ) ;
#21706=LINE ( 'NONE', #22105, #18901 ) ;
#21711=VECTOR ( 'NONE', #8564, 1000.000000000000114 ) ;
#21712=EDGE_LOOP ( 'NONE', ( #19134, #21816, #225, #10830 ) ) ;
#21716=DIRECTION ( 'NONE',  ( -0.000000000000000000, -0.000000000000000000, -1.000000000000000000 ) ) ;
#21718=CARTESIAN_POINT ( 'NONE',  ( -3.784955426773657816, 9.502919080911416572, 10.00000000000000000 ) ) ;
#21722=PLANE ( 'NONE',  #6250 ) ;
#21725=CARTESIAN_POINT ( 'NONE',  ( 0.5000000000000000000, 37.09261900150649893, 10.99387790580546032 ) ) ;
#21727=CARTESIAN_POINT ( 'NONE',  ( -9.204968164644803608, 10.68109904802236798, 10.68306085400111449 ) ) ;
#21728=EDGE_LOOP ( 'NONE', ( #34868, #14851, #1012, #20097 ) ) ;
#21730=DIRECTION ( 'NONE',  ( -0.5877852522924699175, 0.8090169943749498938, 0.000000000000000000 ) ) ;
#21731=CARTESIAN_POINT ( 'NONE',  ( -10.44103466624267362, 32.57396620494226624, 9.500000000000000000 ) ) ;
#21735=CARTESIAN_POINT ( 'NONE',  ( 6.651296319737278750, 27.81603774131160023, 9.000000000000001776 ) ) ;
#21739=VECTOR ( 'NONE', #21428, 1000.000000000000114 ) ;
#21740=ORIENTED_EDGE ( 'NONE', *, *, #4565, .T. ) ;
#21743=DIRECTION ( 'NONE',  ( 1.000000000000000000, 0.000000000000000000, 0.000000000000000000 ) ) ;
#21745=FACE_OUTER_BOUND ( 'NONE', #377, .T. ) ;
#21747=DIRECTION ( 'NONE',  ( 0.000000000000000000, 0.000000000000000000, 1.000000000000000000 ) ) ;
#21749=CARTESIAN_POINT ( 'NONE',  ( -7.468455364333119739, 29.89744377950679421, 10.00000000000000000 ) ) ;
#21753=EDGE_CURVE ( 'NONE', #38096, #26836, #21829, .T. ) ;
#21754=ADVANCED_FACE ( 'NONE', ( #18978 ), #29173, .T. ) ;
#21756=DIRECTION ( 'NONE',  ( -0.3090169943749574988, -0.9510565162951503115, 0.000000000000000000 ) ) ;
#21757=VECTOR ( 'NONE', #25503, 1000.000000000000000 ) ;
#21758=CARTESIAN_POINT ( 'NONE',  ( 0.9685993473471133930, 37.46883198857096886, 7.338691926023209966 ) ) ;
#21760=AXIS2_PLACEMENT_3D ( 'NONE', #20215, #38491, #26305 ) ;
#21762=EDGE_CURVE ( 'NONE', #36822, #36487, #38266, .T. ) ;
#21763=CIRCLE ( 'NONE', #8139, 0.5000000000000004441 ) ;
#21766=CARTESIAN_POINT ( 'NONE',  ( -3.601976756503266763, 7.958898870085802990, 10.68306085400113048 ) ) ;
#21767=ORIENTED_EDGE ( 'NONE', *, *, #29948, .F. ) ;
#21768=EDGE_LOOP ( 'NONE', ( #11361, #11191, #27997, #15854 ) ) ;
#21772=ORIENTED_EDGE ( 'NONE', *, *, #17641, .T. ) ;
#21775=CARTESIAN_POINT ( 'NONE',  ( 13.93732035918235113, 28.04574148721571092, 7.339470489435498735 ) ) ;
#21780=VERTEX_POINT ( 'NONE', #7375 ) ;
#21781=ADVANCED_FACE ( 'NONE', ( #7785 ), #37321, .T. ) ;
#21783=ORIENTED_EDGE ( 'NONE', *, *, #11385, .F. ) ;
#21784=EDGE_CURVE ( 'NONE', #21382, #17580, #14286, .T. ) ;
#21790=VECTOR ( 'NONE', #5137, 1000.000000000000000 ) ;
#21791=CARTESIAN_POINT ( 'NONE',  ( 24.58993327517434224, 16.11278406388105111, 7.000000000000000000 ) ) ;
#21792=CYLINDRICAL_SURFACE ( 'NONE', #12840, 0.5000000000000001110 ) ;
#21793=VECTOR ( 'NONE', #7060, 1000.000000000000000 ) ;
#21794=CARTESIAN_POINT ( 'NONE',  ( 1.278175571583998194, 14.08178954835375940, 7.000000000000000000 ) ) ;
#21796=DIRECTION ( 'NONE',  ( -1.000000000000000000, 0.000000000000000000, 0.000000000000000000 ) ) ;
#21797=EDGE_CURVE ( 'NONE', #2755, #19049, #26678, .T. ) ;
#21798=EDGE_CURVE ( 'NONE', #3986, #14430, #23774, .T. ) ;
#21799=DIRECTION ( 'NONE',  ( 0.000000000000000000, 0.000000000000000000, 1.000000000000000000 ) ) ;
#21800=EDGE_CURVE ( 'NONE', #11758, #31065, #27657, .T. ) ;
#21803=CARTESIAN_POINT ( 'NONE',  ( 2.672146553953307802, 12.33340603770389876, 11.00000000000000000 ) ) ;
#21804=LINE ( 'NONE', #28100, #27887 ) ;
#21806=DIRECTION ( 'NONE',  ( -0.3706816908110125985, -0.7275037805840900429, 0.5773502691896360561 ) ) ;
#21808=ORIENTED_EDGE ( 'NONE', *, *, #13218, .T. ) ;
#21812=DIRECTION ( 'NONE',  ( 1.000000000000000000, 0.000000000000000000, 0.000000000000000000 ) ) ;
#21814=ORIENTED_EDGE ( 'NONE', *, *, #12137, .T. ) ;
#21815=DIRECTION ( 'NONE',  ( 0.000000000000000000, 0.000000000000000000, 1.000000000000000000 ) ) ;
#21816=ORIENTED_EDGE ( 'NONE', *, *, #16122, .F. ) ;
#21818=DIRECTION ( 'NONE',  ( -0.3090169943749572767, -0.9510565162951503115, 0.000000000000000000 ) ) ;
#21820=CARTESIAN_POINT ( 'NONE',  ( 12.51373512357659123, 14.69784138864569911, 10.94387467463329955 ) ) ;
#21825=DIRECTION ( 'NONE',  ( -0.000000000000000000, -0.000000000000000000, -1.000000000000000000 ) ) ;
#21829=CIRCLE ( 'NONE', #17963, 0.4999999999999995559 ) ;
#21830=DIRECTION ( 'NONE',  ( -1.000000000000000000, 0.000000000000000000, 0.000000000000000000 ) ) ;
#21831=FACE_OUTER_BOUND ( 'NONE', #12647, .T. ) ;
#21841=CARTESIAN_POINT ( 'NONE',  ( 22.37674264578617667, 24.85189042352198641, 11.00000000000000000 ) ) ;
#21843=DIRECTION ( 'NONE',  ( -0.5877852522924797984, -0.8090169943749425663, 0.000000000000000000 ) ) ;
#21844=AXIS2_PLACEMENT_3D ( 'NONE', #12885, #33844, #22222 ) ;
#21847=DIRECTION ( 'NONE',  ( 1.000000000000000000, 0.000000000000000000, 0.000000000000000000 ) ) ;
#21849=EDGE_CURVE ( 'NONE', #19377, #38413, #13475, .T. ) ;
#21850=CARTESIAN_POINT ( 'NONE',  ( 14.97009266215792778, 21.42933399866929634, 10.63089969389956480 ) ) ;
#21851=DIRECTION ( 'NONE',  ( 0.9781476007338072431, 0.2079116908177516265, 0.000000000000000000 ) ) ;
#21854=LINE ( 'NONE', #18818, #24476 ) ;
#21855=CARTESIAN_POINT ( 'NONE',  ( -7.470035553104361625, 44.81454624109330354, 7.000000000000000000 ) ) ;
#21861=DIRECTION ( 'NONE',  ( -0.2588190451025293437, -0.9659258262890660918, 0.000000000000000000 ) ) ;
#21862=CARTESIAN_POINT ( 'NONE',  ( -13.33727129354594609, 15.63559704646376147, 7.470097061328788257 ) ) ;
#21868=DIRECTION ( 'NONE',  ( -0.000000000000000000, -0.000000000000000000, -1.000000000000000000 ) ) ;
#21875=LINE ( 'NONE', #30835, #17353 ) ;
#21878=VECTOR ( 'NONE', #31327, 1000.000000000000000 ) ;
#21879=AXIS2_PLACEMENT_3D ( 'NONE', #5246, #18050, #2208 ) ;
#21881=EDGE_LOOP ( 'NONE', ( #10165, #33282, #23360, #39455, #24824 ) ) ;
#21882=CARTESIAN_POINT ( 'NONE',  ( 2.164762040630750395, 7.656889776559952843, 7.338691926023207301 ) ) ;
#21883=EDGE_CURVE ( 'NONE', #19145, #30411, #35215, .T. ) ;
#21884=FACE_OUTER_BOUND ( 'NONE', #29935, .T. ) ;
#21890=ORIENTED_EDGE ( 'NONE', *, *, #32615, .T. ) ;
#21891=DIRECTION ( 'NONE',  ( -0.9945218953682742891, -0.1045284632676437425, 0.000000000000000000 ) ) ;
#21892=ORIENTED_EDGE ( 'NONE', *, *, #13164, .F. ) ;
#21894=CARTESIAN_POINT ( 'NONE',  ( 8.412270287199559604, 10.07085245822950981, 10.49999999999999822 ) ) ;
#21895=LINE ( 'NONE', #25340, #18288 ) ;
#21899=CARTESIAN_POINT ( 'NONE',  ( 8.380596568873530217, 10.11444759148754535, 10.76099332938164288 ) ) ;
#21900=DIRECTION ( 'NONE',  ( 0.3090169943749450643, -0.9510565162951544194, 0.000000000000000000 ) ) ;
#21901=FACE_OUTER_BOUND ( 'NONE', #14348, .T. ) ;
#21902=DIRECTION ( 'NONE',  ( 0.000000000000000000, 0.000000000000000000, 1.000000000000000000 ) ) ;
#21903=LINE ( 'NONE', #12960, #28139 ) ;
#21905=VECTOR ( 'NONE', #27928, 1000.000000000000000 ) ;
#21909=EDGE_CURVE ( 'NONE', #32296, #29828, #38669, .T. ) ;
#21911=CARTESIAN_POINT ( 'NONE',  ( -14.81329996725647469, 19.93755115561707569, 7.000000000000000000 ) ) ;
#21913=VECTOR ( 'NONE', #17870, 1000.000000000000000 ) ;
#21916=CIRCLE ( 'NONE', #4410, 1.000000000000002665 ) ;
#21922=FACE_OUTER_BOUND ( 'NONE', #12279, .T. ) ;
#21923=ORIENTED_EDGE ( 'NONE', *, *, #35923, .F. ) ;
#21925=CARTESIAN_POINT ( 'NONE',  ( -14.58123527826107590, 20.01612550765336707, 10.49999999999999822 ) ) ;
#21926=DIRECTION ( 'NONE',  ( -0.000000000000000000, -0.000000000000000000, -1.000000000000000000 ) ) ;
#21927=CARTESIAN_POINT ( 'NONE',  ( 14.81329996725643738, 19.93755115561686964, 10.50000000000000533 ) ) ;
#21928=ORIENTED_EDGE ( 'NONE', *, *, #21510, .T. ) ;
#21930=CARTESIAN_POINT ( 'NONE',  ( 14.47283171447379502, 21.48159823030311344, 7.500000000000010658 ) ) ;
#21931=EDGE_CURVE ( 'NONE', #31871, #13187, #29527, .T. ) ;
#21932=DIRECTION ( 'NONE',  ( 0.000000000000000000, -0.000000000000000000, -1.000000000000000000 ) ) ;
#21933=ORIENTED_EDGE ( 'NONE', *, *, #28970, .T. ) ;
#21935=EDGE_CURVE ( 'NONE', #25837, #39356, #9807, .T. ) ;
#21939=AXIS2_PLACEMENT_3D ( 'NONE', #27791, #30648, #24735 ) ;
#21940=AXIS2_PLACEMENT_3D ( 'NONE', #33002, #14699, #20996 ) ;
#21944=ADVANCED_FACE ( 'NONE', ( #12235 ), #11446, .F. ) ;
#21945=CIRCLE ( 'NONE', #30407, 15.00000000000000000 ) ;
#21946=FACE_OUTER_BOUND ( 'NONE', #29108, .T. ) ;
#21947=LINE ( 'NONE', #34349, #6580 ) ;
#21949=AXIS2_PLACEMENT_3D ( 'NONE', #38779, #13387, #16651 ) ;
#21950=FACE_OUTER_BOUND ( 'NONE', #1382, .T. ) ;
#21952=CARTESIAN_POINT ( 'NONE',  ( 3.607749162633208329, 7.931741834401768720, 10.59344459855565468 ) ) ;
#21954=DIRECTION ( 'NONE',  ( -0.000000000000000000, -0.000000000000000000, -1.000000000000000000 ) ) ;
#21955=CARTESIAN_POINT ( 'NONE',  ( 12.17073081513896327, 14.31852474926571972, 10.49999999999999822 ) ) ;
#21958=EDGE_CURVE ( 'NONE', #19274, #35202, #20988, .T. ) ;
#21964=CIRCLE ( 'NONE', #24583, 6.000000000000000888 ) ;
#21967=AXIS2_PLACEMENT_3D ( 'NONE', #6859, #778, #25953 ) ;
#21970=CARTESIAN_POINT ( 'NONE',  ( 6.354454053420411697, 35.54304081427980577, 9.000000000000001776 ) ) ;
#21971=VERTEX_POINT ( 'NONE', #5936 ) ;
#21972=ORIENTED_EDGE ( 'NONE', *, *, #18736, .F. ) ;
#21976=EDGE_LOOP ( 'NONE', ( #11602, #18458, #39876, #13723 ) ) ;
#21979=DIRECTION ( 'NONE',  ( -0.000000000000000000, -0.000000000000000000, 1.000000000000000000 ) ) ;
#21980=ORIENTED_EDGE ( 'NONE', *, *, #37446, .F. ) ;
#21982=DIRECTION ( 'NONE',  ( -0.000000000000000000, -0.000000000000000000, 1.000000000000000000 ) ) ;
#21983=DIRECTION ( 'NONE',  ( -1.000000000000000000, 0.000000000000000000, 0.000000000000000000 ) ) ;
#21987=ORIENTED_EDGE ( 'NONE', *, *, #37902, .F. ) ;
#21991=ORIENTED_EDGE ( 'NONE', *, *, #31621, .T. ) ;
#21994=CARTESIAN_POINT ( 'NONE',  ( -14.54089481611321055, 26.18321485943229376, 7.323837789871779691 ) ) ;
#21996=VECTOR ( 'NONE', #39451, 1000.000000000000000 ) ;
#21997=VECTOR ( 'NONE', #36312, 1000.000000000000000 ) ;
#21999=FACE_OUTER_BOUND ( 'NONE', #4245, .T. ) ;
#22005=LINE ( 'NONE', #25054, #35216 ) ;
#22009=EDGE_CURVE ( 'NONE', #4170, #18302, #12028, .T. ) ;
#22011=ORIENTED_EDGE ( 'NONE', *, *, #3954, .F. ) ;
#22018=ORIENTED_EDGE ( 'NONE', *, *, #23183, .F. ) ;
#22022=CARTESIAN_POINT ( 'NONE',  ( 12.14063985594365924, 14.34296697341676641, 10.49999999999999822 ) ) ;
#22023=AXIS2_PLACEMENT_3D ( 'NONE', #17180, #38088, #32204 ) ;
#22024=ORIENTED_EDGE ( 'NONE', *, *, #18311, .T. ) ;
#22027=DIRECTION ( 'NONE',  ( -1.000000000000000000, 0.000000000000000000, 0.000000000000000000 ) ) ;
#22029=VERTEX_POINT ( 'NONE', #21185 ) ;
#22031=DIRECTION ( 'NONE',  ( -1.000000000000000000, 0.000000000000000000, 0.000000000000000000 ) ) ;
#22033=CARTESIAN_POINT ( 'NONE',  ( -0.5000000000000004441, 37.00000000000000711, 7.000000000000000000 ) ) ;
#22034=VECTOR ( 'NONE', #3613, 1000.000000000000114 ) ;
#22035=ORIENTED_EDGE ( 'NONE', *, *, #3242, .F. ) ;
#22037=EDGE_CURVE ( 'NONE', #31380, #8749, #17039, .T. ) ;
#22039=EDGE_CURVE ( 'NONE', #5579, #28502, #39289, .T. ) ;
#22041=VERTEX_POINT ( 'NONE', #39470 ) ;
#22043=CARTESIAN_POINT ( 'NONE',  ( 4.577399223880713741, 35.23960032125091146, 9.500000000000000000 ) ) ;
#22044=EDGE_CURVE ( 'NONE', #24787, #24416, #4255, .T. ) ;
#22045=VERTEX_POINT ( 'NONE', #27473 ) ;
#22046=DIRECTION ( 'NONE',  ( 0.8090169943749421222, -0.5877852522924804646, 0.000000000000000000 ) ) ;
#22047=CARTESIAN_POINT ( 'NONE',  ( -0.5000000000000004441, 37.00000000000000711, 7.000000000000000000 ) ) ;
#22048=CARTESIAN_POINT ( 'NONE',  ( -14.86556419889029534, 20.43481210330121556, 7.000000000000000000 ) ) ;
#22050=DIRECTION ( 'NONE',  ( 0.6459741880212479526, 0.2876062384759398016, 0.7071067811865549002 ) ) ;
#22051=DIRECTION ( 'NONE',  ( 0.4067366430758010409, 0.9135454576426005335, -0.000000000000000000 ) ) ;
#22053=AXIS2_PLACEMENT_3D ( 'NONE', #171, #24951, #34500 ) ;
#22055=PLANE ( 'NONE',  #2417 ) ;
#22056=DIRECTION ( 'NONE',  ( 0.7431448254773953543, 0.6691306063588570163, 0.000000000000000000 ) ) ;
#22057=DIRECTION ( 'NONE',  ( -0.000000000000000000, -0.000000000000000000, -1.000000000000000000 ) ) ;
#22058=EDGE_CURVE ( 'NONE', #6246, #16446, #2505, .T. ) ;
#22060=CARTESIAN_POINT ( 'NONE',  ( -2.036571916123810055, 8.108948098542073879, 10.50000000000000355 ) ) ;
#22061=ORIENTED_EDGE ( 'NONE', *, *, #14052, .T. ) ;
#22064=CARTESIAN_POINT ( 'NONE',  ( -13.28503138821885798, 15.53523575316151195, 7.499999999999993783 ) ) ;
#22077=ORIENTED_EDGE ( 'NONE', *, *, #24968, .F. ) ;
#22079=DIRECTION ( 'NONE',  ( 0.5877852522924689183, -0.8090169943749505599, -0.000000000000000000 ) ) ;
#22081=B_SPLINE_CURVE_WITH_KNOTS ( 'NONE', 3,
 ( #39959, #12135, #24523, #34074 ),
 .UNSPECIFIED., .F., .F.,
 ( 4, 4 ),
 ( 0.8666666404939821211, 1.000000000000000000 ),
 .UNSPECIFIED. ) ;
#22084=EDGE_CURVE ( 'NONE', #17936, #1570, #17756, .T. ) ;
#22086=VERTEX_POINT ( 'NONE', #11649 ) ;
#22088=CARTESIAN_POINT ( 'NONE',  ( 8.368303251206119953, 20.48707633493483371, 9.000000000000001776 ) ) ;
#22089=FACE_OUTER_BOUND ( 'NONE', #444, .T. ) ;
#22090=AXIS2_PLACEMENT_3D ( 'NONE', #30608, #18616, #39738 ) ;
#22094=ORIENTED_EDGE ( 'NONE', *, *, #24508, .F. ) ;
#22095=CARTESIAN_POINT ( 'NONE',  ( -12.23327497914565853, 13.81973598992469121, 7.000000000000000000 ) ) ;
#22097=DIRECTION ( 'NONE',  ( -0.5877852522924797984, -0.8090169943749426773, 0.000000000000000000 ) ) ;
#22099=CARTESIAN_POINT ( 'NONE',  ( -19.48557158514982390, 33.75000000000009948, 7.000000000000000000 ) ) ;
#22100=EDGE_LOOP ( 'NONE', ( #27869, #33789, #33267, #4713 ) ) ;
#22103=DIRECTION ( 'NONE',  ( -0.6691306063588678965, -0.7431448254773855844, 0.000000000000000000 ) ) ;
#22104=CARTESIAN_POINT ( 'NONE',  ( -0.5000000000000026645, 32.50000000000000000, 10.50000000000000000 ) ) ;
#22105=CARTESIAN_POINT ( 'NONE',  ( -7.096882951594427169, 29.56287847632736288, 10.00000000000000000 ) ) ;
#22106=FACE_OUTER_BOUND ( 'NONE', #29488, .T. ) ;
#22107=CARTESIAN_POINT ( 'NONE',  ( -10.81260707898136531, 32.90853150812170469, 10.63089969389957901 ) ) ;
#22115=VECTOR ( 'NONE', #32716, 1000.000000000000000 ) ;
#22123=CARTESIAN_POINT ( 'NONE',  ( 13.63581098909226519, 27.45627467658428600, 10.99999999999999289 ) ) ;
#22124=CARTESIAN_POINT ( 'NONE',  ( 5.644276917315718123, 36.40655018617690786, 10.49999999999999822 ) ) ;
#22125=EDGE_LOOP ( 'NONE', ( #7732, #4033, #22398, #21198 ) ) ;
#22127=DIRECTION ( 'NONE',  ( 0.7032331762534027586, -0.07391278520357077997, -0.7071067811865484609 ) ) ;
#22128=CIRCLE ( 'NONE', #37042, 15.00000000000000000 ) ;
#22129=DIRECTION ( 'NONE',  ( 0.9945218953682730678, -0.1045284632676569819, 0.000000000000000000 ) ) ;
#22130=ORIENTED_EDGE ( 'NONE', *, *, #23363, .T. ) ;
#22132=LINE ( 'NONE', #25376, #38802 ) ;
#22133=PLANE ( 'NONE',  #17416 ) ;
#22134=B_SPLINE_CURVE_WITH_KNOTS ( 'NONE', 3,
 ( #14770, #34451, #9268, #40139 ),
 .UNSPECIFIED., .F., .F.,
 ( 4, 4 ),
 ( 0.000000000000000000, 1.000000000000000000 ),
 .UNSPECIFIED. ) ;
#22138=EDGE_LOOP ( 'NONE', ( #33255, #22623, #38414, #36629 ) ) ;
#22142=PLANE ( 'NONE',  #35258 ) ;
#22145=CARTESIAN_POINT ( 'NONE',  ( -13.28503138821885798, 15.53523575316151195, 7.499999999999993783 ) ) ;
#22147=CARTESIAN_POINT ( 'NONE',  ( -10.72918489117944674, 32.98258515686310943, 7.500000000000004441 ) ) ;
#22149=CARTESIAN_POINT ( 'NONE',  ( -14.36830325120615903, 20.48707633493503621, 7.500000000000004441 ) ) ;
#22150=CARTESIAN_POINT ( 'NONE',  ( -13.05736835487441994, 16.11602540378456183, 9.500000000000000000 ) ) ;
#22153=CIRCLE ( 'NONE', #28624, 0.5000000000000004441 ) ;
#22155=EDGE_CURVE ( 'NONE', #24567, #747, #24761, .T. ) ;
#22164=CONICAL_SURFACE ( 'NONE', #11135, 1.000000000000000888, 0.7853981633974548293 ) ;
#22165=DIRECTION ( 'NONE',  ( 1.000000000000000000, 0.000000000000000000, 0.000000000000000000 ) ) ;
#22167=EDGE_LOOP ( 'NONE', ( #34587, #23151, #11750 ) ) ;
#22170=CARTESIAN_POINT ( 'NONE',  ( -6.460609604078108248, 35.78147008481153080, 10.94611345180489970 ) ) ;
#22174=DIRECTION ( 'NONE',  ( 1.000000000000000000, 0.000000000000000000, 0.000000000000000000 ) ) ;
#22175=ORIENTED_EDGE ( 'NONE', *, *, #22710, .F. ) ;
#22179=VERTEX_POINT ( 'NONE', #17303 ) ;
#22181=VERTEX_POINT ( 'NONE', #13427 ) ;
#22188=DIRECTION ( 'NONE',  ( 0.000000000000000000, 0.000000000000000000, 1.000000000000000000 ) ) ;
#22190=CARTESIAN_POINT ( 'NONE',  ( 10.44103466624280685, 32.57396620494213124, 9.000000000000001776 ) ) ;
#22192=AXIS2_PLACEMENT_3D ( 'NONE', #30590, #15936, #18393 ) ;
#22193=LINE ( 'NONE', #18957, #6088 ) ;
#22198=EDGE_CURVE ( 'NONE', #22676, #11758, #10086, .T. ) ;
#22200=ORIENTED_EDGE ( 'NONE', *, *, #24420, .F. ) ;
#22202=AXIS2_PLACEMENT_3D ( 'NONE', #13456, #16520, #19357 ) ;
#22204=DIRECTION ( 'NONE',  ( 0.2926062055178220711, -0.7622652262560022374, 0.5773502691896384986 ) ) ;
#22206=VERTEX_POINT ( 'NONE', #38820 ) ;
#22208=ORIENTED_EDGE ( 'NONE', *, *, #29999, .T. ) ;
#22210=DIRECTION ( 'NONE',  ( -1.000000000000000000, 0.000000000000000000, 0.000000000000000000 ) ) ;
#22213=ORIENTED_EDGE ( 'NONE', *, *, #12994, .T. ) ;
#22216=LINE ( 'NONE', #22824, #19624 ) ;
#22220=CYLINDRICAL_SURFACE ( 'NONE', #38148, 0.5000000000000004441 ) ;
#22221=CIRCLE ( 'NONE', #23543, 0.5000000000000004441 ) ;
#22222=DIRECTION ( 'NONE',  ( 0.9510565162951543083, 0.3090169943749450088, 0.000000000000000000 ) ) ;
#22223=CARTESIAN_POINT ( 'NONE',  ( -13.22516817658055288, 40.70288237343638826, 7.000000000000000000 ) ) ;
#22224=ORIENTED_EDGE ( 'NONE', *, *, #34171, .T. ) ;
#22227=AXIS2_PLACEMENT_3D ( 'NONE', #27034, #1655, #38622 ) ;
#22230=EDGE_CURVE ( 'NONE', #15233, #5452, #27600, .T. ) ;
#22232=PLANE ( 'NONE',  #5048 ) ;
#22233=AXIS2_PLACEMENT_3D ( 'NONE', #5521, #17934, #2880 ) ;
#22235=LINE ( 'NONE', #21647, #26206 ) ;
#22236=AXIS2_PLACEMENT_3D ( 'NONE', #14017, #26407, #32722 ) ;
#22237=LINE ( 'NONE', #16561, #33769 ) ;
#22238=DIRECTION ( 'NONE',  ( -1.000000000000000000, 0.000000000000000000, 0.000000000000000000 ) ) ;
#22240=CARTESIAN_POINT ( 'NONE',  ( 14.97009266215792778, 21.42933399866928568, 10.49999999999999822 ) ) ;
#22241=CARTESIAN_POINT ( 'NONE',  ( -3.610593701936590794, 31.83882289796395426, 10.50000000000000533 ) ) ;
#22243=CARTESIAN_POINT ( 'NONE',  ( -1.693998953219646664, 12.12549434688617644, 10.50000000000000000 ) ) ;
#22245=DIRECTION ( 'NONE',  ( 1.000000000000000000, 0.000000000000000000, 0.000000000000000000 ) ) ;
#22248=DIRECTION ( 'NONE',  ( -0.4156269377774519658, 0.5720614028176885801, 0.7071067811865450192 ) ) ;
#22250=CIRCLE ( 'NONE', #33308, 0.4999999999999997780 ) ;
#22253=LINE ( 'NONE', #34463, #39953 ) ;
#22254=ADVANCED_FACE ( 'NONE', ( #4494 ), #24921, .T. ) ;
#22256=DIRECTION ( 'NONE',  ( 0.9510565162951541973, 0.3090169943749456194, 1.040834085586083783E-14 ) ) ;
#22258=ORIENTED_EDGE ( 'NONE', *, *, #34421, .T. ) ;
#22260=VERTEX_POINT ( 'NONE', #26829 ) ;
#22264=EDGE_CURVE ( 'NONE', #445, #8575, #20544, .T. ) ;
#22268=EDGE_LOOP ( 'NONE', ( #39053, #25479, #2956, #11091 ) ) ;
#22270=FACE_OUTER_BOUND ( 'NONE', #24733, .T. ) ;
#22272=VECTOR ( 'NONE', #18166, 1000.000000000000000 ) ;
#22273=ORIENTED_EDGE ( 'NONE', *, *, #32223, .T. ) ;
#22275=VECTOR ( 'NONE', #24314, 1000.000000000000000 ) ;
#22277=ORIENTED_EDGE ( 'NONE', *, *, #23307, .T. ) ;
#22281=EDGE_CURVE ( 'NONE', #26114, #12596, #2326, .T. ) ;
#22283=ADVANCED_FACE ( 'NONE', ( #8746 ), #15911, .T. ) ;
#22285=EDGE_CURVE ( 'NONE', #13694, #18489, #5488, .T. ) ;
#22297=CARTESIAN_POINT ( 'NONE',  ( 5.644276917315719899, 36.40655018617690786, 10.49999999999999822 ) ) ;
#22298=FACE_OUTER_BOUND ( 'NONE', #1484, .T. ) ;
#22304=CARTESIAN_POINT ( 'NONE',  ( 2.501562340374731352, 7.696614566897833853, 10.50000000000000000 ) ) ;
#22305=ORIENTED_EDGE ( 'NONE', *, *, #25010, .T. ) ;
#22308=LINE ( 'NONE', #779, #3648 ) ;
#22309=EDGE_CURVE ( 'NONE', #10247, #22086, #30286, .T. ) ;
#22314=CARTESIAN_POINT ( 'NONE',  ( 9.331903152615748098, 11.35703883385568780, 10.49999999999999645 ) ) ;
#22315=VECTOR ( 'NONE', #2177, 999.9999999999998863 ) ;
#22320=CARTESIAN_POINT ( 'NONE',  ( 14.11133924723984201, 27.61078317377173619, 10.59344459855563514 ) ) ;
#22321=DIRECTION ( 'NONE',  ( -0.4999999999999919509, 0.8660254037844432595, 0.000000000000000000 ) ) ;
#22324=CARTESIAN_POINT ( 'NONE',  ( 14.86131180699620735, 21.44076732726258072, 10.82238861112335471 ) ) ;
#22328=DIRECTION ( 'NONE',  ( 0.3090169943749450643, -0.9510565162951544194, 0.000000000000000000 ) ) ;
#22332=ORIENTED_EDGE ( 'NONE', *, *, #36476, .F. ) ;
#22334=AXIS2_PLACEMENT_3D ( 'NONE', #26257, #37504, #18624 ) ;
#22335=VERTEX_POINT ( 'NONE', #32938 ) ;
#22337=DIRECTION ( 'NONE',  ( -0.6691306063588653430, -0.7431448254773878048, 0.000000000000000000 ) ) ;
#22338=CARTESIAN_POINT ( 'NONE',  ( 6.774334011770120512, 35.84443018111158352, 10.49999999999999822 ) ) ;
#22340=VECTOR ( 'NONE', #25687, 1000.000000000000114 ) ;
#22342=ORIENTED_EDGE ( 'NONE', *, *, #29798, .F. ) ;
#22343=CARTESIAN_POINT ( 'NONE',  ( 3.607749162633205220, 7.931741834401766944, 10.50000000000000178 ) ) ;
#22345=CARTESIAN_POINT ( 'NONE',  ( 0.000000000000000000, 22.50000000000000355, 7.000000000000000000 ) ) ;
#22349=VERTEX_POINT ( 'NONE', #2456 ) ;
#22352=DIRECTION ( 'NONE',  ( -0.000000000000000000, -0.000000000000000000, 1.000000000000000000 ) ) ;
#22353=VECTOR ( 'NONE', #38001, 1000.000000000000114 ) ;
#22354=ORIENTED_EDGE ( 'NONE', *, *, #28655, .T. ) ;
#22358=LINE ( 'NONE', #16481, #18555 ) ;
#22359=ORIENTED_EDGE ( 'NONE', *, *, #15873, .F. ) ;
#22360=ORIENTED_EDGE ( 'NONE', *, *, #6509, .F. ) ;
#22368=DIRECTION ( 'NONE',  ( -0.000000000000000000, 0.000000000000000000, -1.000000000000000000 ) ) ;
#22369=ORIENTED_EDGE ( 'NONE', *, *, #30723, .T. ) ;
#22371=CARTESIAN_POINT ( 'NONE',  ( 13.94482798346721175, 26.50521816028912525, 11.00000000000000000 ) ) ;
#22372=LINE ( 'NONE', #34778, #35548 ) ;
#22379=ADVANCED_FACE ( 'NONE', ( #23781 ), #32154, .T. ) ;
#22382=CARTESIAN_POINT ( 'NONE',  ( -1.693998953219642223, 12.12549434688618888, 11.00000000000000000 ) ) ;
#22383=AXIS2_PLACEMENT_3D ( 'NONE', #33085, #20487, #23327 ) ;
#22385=DIRECTION ( 'NONE',  ( 0.3090169943749574988, 0.9510565162951503115, 0.000000000000000000 ) ) ;
#22386=EDGE_CURVE ( 'NONE', #37263, #1779, #27231, .T. ) ;
#22387=DIRECTION ( 'NONE',  ( 0.000000000000000000, 0.000000000000000000, 1.000000000000000000 ) ) ;
#22388=EDGE_CURVE ( 'NONE', #39356, #14996, #6201, .T. ) ;
#22389=VECTOR ( 'NONE', #33826, 1000.000000000000000 ) ;
#22396=DIRECTION ( 'NONE',  ( 1.000000000000000000, 0.000000000000000000, 0.000000000000000000 ) ) ;
#22398=ORIENTED_EDGE ( 'NONE', *, *, #3274, .T. ) ;
#22406=CYLINDRICAL_SURFACE ( 'NONE', #38476, 0.5000000000000007772 ) ;
#22407=ORIENTED_EDGE ( 'NONE', *, *, #37188, .T. ) ;
#22409=CARTESIAN_POINT ( 'NONE',  ( -12.80736835487442349, 15.68301270189233954, 11.00000000000000000 ) ) ;
#22411=CARTESIAN_POINT ( 'NONE',  ( 12.23768179954923419, 14.31935546172391760, 10.49999999999999822 ) ) ;
#22412=ORIENTED_EDGE ( 'NONE', *, *, #34397, .T. ) ;
#22415=DIRECTION ( 'NONE',  ( 1.000000000000000000, 0.000000000000000000, 0.000000000000000000 ) ) ;
#22419=FACE_OUTER_BOUND ( 'NONE', #22609, .T. ) ;
#22421=DIRECTION ( 'NONE',  ( 1.000000000000000000, 0.000000000000000000, 0.000000000000000000 ) ) ;
#22422=ORIENTED_EDGE ( 'NONE', *, *, #37609, .T. ) ;
#22425=VECTOR ( 'NONE', #39355, 1000.000000000000000 ) ;
#22428=VECTOR ( 'NONE', #39359, 1000.000000000000000 ) ;
#22429=ORIENTED_EDGE ( 'NONE', *, *, #2844, .F. ) ;
#22432=FACE_OUTER_BOUND ( 'NONE', #32501, .T. ) ;
#22433=ORIENTED_EDGE ( 'NONE', *, *, #17566, .F. ) ;
#22435=CARTESIAN_POINT ( 'NONE',  ( -11.44473057578096942, 31.45924896672619298, 11.00000000000000000 ) ) ;
#22436=CARTESIAN_POINT ( 'NONE',  ( -11.17899463792456771, 31.89279561836819710, 10.99387789255783687 ) ) ;
#22439=CARTESIAN_POINT ( 'NONE',  ( -6.506711629694017063, 35.47525137376727855, 10.83333333333333215 ) ) ;
#22444=AXIS2_PLACEMENT_3D ( 'NONE', #22967, #20135, #26620 ) ;
#22446=DIRECTION ( 'NONE',  ( -0.2079116908177655043, -0.9781476007338044676, -0.000000000000000000 ) ) ;
#22449=DIRECTION ( 'NONE',  ( 0.9781476007338069101, 0.2079116908177532363, 0.000000000000000000 ) ) ;
#22450=VERTEX_POINT ( 'NONE', #8947 ) ;
#22453=CARTESIAN_POINT ( 'NONE',  ( -8.910254037844428154, 17.93301270189230223, 10.00000000000000000 ) ) ;
#22458=EDGE_CURVE ( 'NONE', #4444, #32326, #17238, .T. ) ;
#22459=CARTESIAN_POINT ( 'NONE',  ( 10.14060191828658120, 25.26915018278934255, 10.00000000000000000 ) ) ;
#22463=ORIENTED_EDGE ( 'NONE', *, *, #6911, .T. ) ;
#22464=CARTESIAN_POINT ( 'NONE',  ( 21.24426311945340373, 15.07158936841587860, 11.00000000000000000 ) ) ;
#22470=ORIENTED_EDGE ( 'NONE', *, *, #35598, .F. ) ;
#22472=LINE ( 'NONE', #7433, #23222 ) ;
#22478=FACE_OUTER_BOUND ( 'NONE', #37464, .T. ) ;
#22479=CARTESIAN_POINT ( 'NONE',  ( -3.295881626406750087, 9.398963235502531433, 9.500000000000000000 ) ) ;
#22485=ORIENTED_EDGE ( 'NONE', *, *, #2715, .T. ) ;
#22486=ORIENTED_EDGE ( 'NONE', *, *, #821, .T. ) ;
#22487=LINE ( 'NONE', #37741, #30101 ) ;
#22493=CARTESIAN_POINT ( 'NONE',  ( -10.03245514394471627, 31.53326318584470656, 7.000000000000000000 ) ) ;
#22496=CARTESIAN_POINT ( 'NONE',  ( 2.629601561899394202, 7.723830143584017094, 10.63089969389957545 ) ) ;
#22499=ORIENTED_EDGE ( 'NONE', *, *, #7760, .T. ) ;
#22504=DIRECTION ( 'NONE',  ( 0.8660254037844363761, -0.5000000000000039968, -0.000000000000000000 ) ) ;
#22507=DIRECTION ( 'NONE',  ( 0.9945218953682727347, -0.1045284632676597436, 6.938893903907217334E-15 ) ) ;
#22508=EDGE_CURVE ( 'NONE', #35497, #13010, #12784, .T. ) ;
#22509=AXIS2_PLACEMENT_3D ( 'NONE', #18546, #18347, #3101 ) ;
#22514=CARTESIAN_POINT ( 'NONE',  ( 13.72527515842283741, 27.95206079998155957, 10.49999999999999822 ) ) ;
#22515=FACE_OUTER_BOUND ( 'NONE', #1703, .T. ) ;
#22518=CONICAL_SURFACE ( 'NONE', #12785, 1.000000000000013101, 0.7853981633974582710 ) ;
#22519=DIRECTION ( 'NONE',  ( 0.6691306063588569053, -0.7431448254773954654, 0.000000000000000000 ) ) ;
#22520=ORIENTED_EDGE ( 'NONE', *, *, #17791, .F. ) ;
#22522=DIRECTION ( 'NONE',  ( -0.000000000000000000, -0.000000000000000000, -1.000000000000000000 ) ) ;
#22523=DIRECTION ( 'NONE',  ( -0.000000000000000000, -0.000000000000000000, -1.000000000000000000 ) ) ;
#22524=ORIENTED_EDGE ( 'NONE', *, *, #15585, .T. ) ;
#22527=EDGE_CURVE ( 'NONE', #30503, #4287, #34329, .T. ) ;
#22528=EDGE_LOOP ( 'NONE', ( #23919, #24175, #14542, #35755 ) ) ;
#22530=EDGE_CURVE ( 'NONE', #10650, #1084, #27217, .T. ) ;
#22531=ORIENTED_EDGE ( 'NONE', *, *, #38206, .F. ) ;
#22534=DIRECTION ( 'NONE',  ( -1.000000000000000000, 0.000000000000000000, 0.000000000000000000 ) ) ;
#22535=LINE ( 'NONE', #10562, #4650 ) ;
#22537=AXIS2_PLACEMENT_3D ( 'NONE', #38425, #7744, #7542 ) ;
#22539=ADVANCED_FACE ( 'NONE', ( #25370 ), #37984, .T. ) ;
#22540=DIRECTION ( 'NONE',  ( -0.000000000000000000, 0.000000000000000000, 1.000000000000000000 ) ) ;
#22541=ORIENTED_EDGE ( 'NONE', *, *, #16104, .F. ) ;
#22543=CARTESIAN_POINT ( 'NONE',  ( 3.992867117591230919, 8.524771480177550487, 7.499999999999990230 ) ) ;
#22544=CYLINDRICAL_SURFACE ( 'NONE', #68, 0.4999999999999997780 ) ;
#22545=AXIS2_PLACEMENT_3D ( 'NONE', #24695, #37092, #9259 ) ;
#22546=DIRECTION ( 'NONE',  ( -0.000000000000000000, -0.000000000000000000, -1.000000000000000000 ) ) ;
#22548=AXIS2_PLACEMENT_3D ( 'NONE', #15943, #19381, #31780 ) ;
#22552=DIRECTION ( 'NONE',  ( -0.000000000000000000, -0.000000000000000000, -1.000000000000000000 ) ) ;
#22554=EDGE_CURVE ( 'NONE', #29633, #27849, #6285, .T. ) ;
#22555=DIRECTION ( 'NONE',  ( -0.7431448254773863615, 0.6691306063588670083, 0.000000000000000000 ) ) ;
#22556=EDGE_CURVE ( 'NONE', #4057, #36810, #37850, .T. ) ;
#22557=ORIENTED_EDGE ( 'NONE', *, *, #28240, .F. ) ;
#22563=VERTEX_POINT ( 'NONE', #12189 ) ;
#22564=AXIS2_PLACEMENT_3D ( 'NONE', #25211, #18723, #19313 ) ;
#22566=DIRECTION ( 'NONE',  ( -0.9510565162951503115, 0.3090169943749572767, 0.000000000000000000 ) ) ;
#22568=AXIS2_PLACEMENT_3D ( 'NONE', #2260, #29483, #14650 ) ;
#22571=LINE ( 'NONE', #35173, #36513 ) ;
#22572=ORIENTED_EDGE ( 'NONE', *, *, #8280, .F. ) ;
#22574=CARTESIAN_POINT ( 'NONE',  ( 14.42035624161478857, 26.65972665747660386, 10.63089969389957190 ) ) ;
#22576=CIRCLE ( 'NONE', #20010, 0.5000000000000004441 ) ;
#22577=ORIENTED_EDGE ( 'NONE', *, *, #27197, .T. ) ;
#22580=EDGE_CURVE ( 'NONE', #1489, #4691, #27828, .T. ) ;
#22581=ORIENTED_EDGE ( 'NONE', *, *, #32395, .F. ) ;
#22583=VECTOR ( 'NONE', #22725, 1000.000000000000000 ) ;
#22584=DIRECTION ( 'NONE',  ( 0.9135454576426059736, 0.4067366430757888285, -0.000000000000000000 ) ) ;
#22587=ORIENTED_EDGE ( 'NONE', *, *, #5658, .T. ) ;
#22591=DIRECTION ( 'NONE',  ( -0.4999999999999921729, 0.8660254037844432595, 0.000000000000000000 ) ) ;
#22594=AXIS2_PLACEMENT_3D ( 'NONE', #17510, #17106, #14439 ) ;
#22599=CIRCLE ( 'NONE', #5104, 0.5000000000000004441 ) ;
#22601=ORIENTED_EDGE ( 'NONE', *, *, #26999, .F. ) ;
#22604=ORIENTED_EDGE ( 'NONE', *, *, #7069, .T. ) ;
#22607=FACE_OUTER_BOUND ( 'NONE', #34580, .T. ) ;
#22609=EDGE_LOOP ( 'NONE', ( #8342, #10431, #21358 ) ) ;
#22612=DIRECTION ( 'NONE',  ( -0.8660254037844432595, -0.4999999999999920064, 0.000000000000000000 ) ) ;
#22615=FACE_OUTER_BOUND ( 'NONE', #9435, .T. ) ;
#22617=DIRECTION ( 'NONE',  ( 0.9510565162951507556, -0.3090169943749560000, -2.144236138472114690E-15 ) ) ;
#22621=DIRECTION ( 'NONE',  ( 1.000000000000000000, 0.000000000000000000, 0.000000000000000000 ) ) ;
#22623=ORIENTED_EDGE ( 'NONE', *, *, #15575, .T. ) ;
#22625=DIRECTION ( 'NONE',  ( 1.000000000000000000, 0.000000000000000000, 0.000000000000000000 ) ) ;
#22627=VERTEX_POINT ( 'NONE', #25181 ) ;
#22630=AXIS2_PLACEMENT_3D ( 'NONE', #40151, #33681, #12325 ) ;
#22632=ORIENTED_EDGE ( 'NONE', *, *, #11715, .F. ) ;
#22633=VECTOR ( 'NONE', #25245, 999.9999999999998863 ) ;
#22635=DIRECTION ( 'NONE',  ( 0.000000000000000000, 0.000000000000000000, 1.000000000000000000 ) ) ;
#22638=DIRECTION ( 'NONE',  ( -1.224646799147351235E-16, 1.000000000000000000, 0.000000000000000000 ) ) ;
#22639=LINE ( 'NONE', #19808, #29438 ) ;
#22640=CARTESIAN_POINT ( 'NONE',  ( 14.52509594610761923, 21.97885917798724975, 11.00000000000000000 ) ) ;
#22643=CARTESIAN_POINT ( 'NONE',  ( 3.503793317224320969, 8.420815634768672453, 11.00000000000000000 ) ) ;
#22645=FACE_OUTER_BOUND ( 'NONE', #31629, .T. ) ;
#22646=DIRECTION ( 'NONE',  ( -0.000000000000000000, -0.000000000000000000, -1.000000000000000000 ) ) ;
#22650=ORIENTED_EDGE ( 'NONE', *, *, #36353, .F. ) ;
#22652=DIRECTION ( 'NONE',  ( 0.000000000000000000, -0.000000000000000000, 1.000000000000000000 ) ) ;
#22653=EDGE_CURVE ( 'NONE', #38699, #3260, #21763, .T. ) ;
#22655=CARTESIAN_POINT ( 'NONE',  ( 12.68475447279711510, 27.14725768220934654, 9.500000000000000000 ) ) ;
#22657=VERTEX_POINT ( 'NONE', #28422 ) ;
#22663=CARTESIAN_POINT ( 'NONE',  ( 14.12406941186438125, 26.56345723075634524, 10.96580508970281009 ) ) ;
#22669=EDGE_CURVE ( 'NONE', #10635, #39810, #13325, .T. ) ;
#22670=ORIENTED_EDGE ( 'NONE', *, *, #31912, .T. ) ;
#22674=EDGE_CURVE ( 'NONE', #10078, #3614, #37373, .T. ) ;
#22676=VERTEX_POINT ( 'NONE', #599 ) ;
#22684=EDGE_CURVE ( 'NONE', #6323, #7643, #1809, .T. ) ;
#22685=ORIENTED_EDGE ( 'NONE', *, *, #23538, .F. ) ;
#22687=VERTEX_POINT ( 'NONE', #5403 ) ;
#22688=ADVANCED_FACE ( 'NONE', ( #26738 ), #20250, .T. ) ;
#22689=VECTOR ( 'NONE', #25741, 1000.000000000000000 ) ;
#22695=DIRECTION ( 'NONE',  ( 0.1045284632676437703, -0.9945218953682742891, 0.000000000000000000 ) ) ;
#22696=CARTESIAN_POINT ( 'NONE',  ( 14.11133924723984379, 27.61078317377176106, 10.63089969389956480 ) ) ;
#22697=LINE ( 'NONE', #28599, #2665 ) ;
#22698=DIRECTION ( 'NONE',  ( -0.000000000000000000, 0.000000000000000000, 1.000000000000000000 ) ) ;
#22699=CARTESIAN_POINT ( 'NONE',  ( -10.63499050845675775, 32.74860482968701092, 10.94611345180490680 ) ) ;
#22702=ORIENTED_EDGE ( 'NONE', *, *, #19562, .F. ) ;
#22704=DIRECTION ( 'NONE',  ( -0.6691306063588671194, -0.7431448254773863615, 0.000000000000000000 ) ) ;
#22705=DIRECTION ( 'NONE',  ( 0.000000000000000000, 0.000000000000000000, -1.000000000000000000 ) ) ;
#22707=CARTESIAN_POINT ( 'NONE',  ( -3.784955426773653375, 9.502919080911414795, 10.50000000000000000 ) ) ;
#22710=EDGE_CURVE ( 'NONE', #6233, #31812, #15129, .T. ) ;
#22719=CIRCLE ( 'NONE', #28550, 6.000000000000014211 ) ;
#22721=VERTEX_POINT ( 'NONE', #17002 ) ;
#22722=DIRECTION ( 'NONE',  ( -0.000000000000000000, -0.000000000000000000, -1.000000000000000000 ) ) ;
#22725=DIRECTION ( 'NONE',  ( 0.000000000000000000, 0.000000000000000000, -1.000000000000000000 ) ) ;
#22730=EDGE_LOOP ( 'NONE', ( #11634, #25220, #31391, #13277, #34722 ) ) ;
#22732=VECTOR ( 'NONE', #39938, 1000.000000000000000 ) ;
#22733=ORIENTED_EDGE ( 'NONE', *, *, #10603, .F. ) ;
#22736=EDGE_CURVE ( 'NONE', #30411, #4180, #23293, .T. ) ;
#22737=CARTESIAN_POINT ( 'NONE',  ( 13.94482798346721175, 26.50521816028912525, 11.00000000000000000 ) ) ;
#22738=CARTESIAN_POINT ( 'NONE',  ( 8.401171878996485987, 21.11424711454080594, 9.000000000000001776 ) ) ;
#22742=ORIENTED_EDGE ( 'NONE', *, *, #29113, .F. ) ;
#22745=DIRECTION ( 'NONE',  ( -1.000000000000000000, 0.000000000000000000, 0.000000000000000000 ) ) ;
#22751=CARTESIAN_POINT ( 'NONE',  ( 11.44473057578109199, 31.45924896672603310, 7.499999999999997335 ) ) ;
#22753=CARTESIAN_POINT ( 'NONE',  ( 7.111215932167702647, 17.81698729810774751, 9.000000000000001776 ) ) ;
#22755=EDGE_CURVE ( 'NONE', #26378, #6957, #38730, .T. ) ;
#22761=ADVANCED_FACE ( 'NONE', ( #5002 ), #39124, .F. ) ;
#22762=EDGE_CURVE ( 'NONE', #21433, #8840, #26541, .T. ) ;
#22764=VERTEX_POINT ( 'NONE', #35484 ) ;
#22767=LINE ( 'NONE', #7325, #37302 ) ;
#22771=DIRECTION ( 'NONE',  ( -0.2079116908177688350, -0.9781476007338035794, 0.000000000000000000 ) ) ;
#22772=VERTEX_POINT ( 'NONE', #11309 ) ;
#22775=CARTESIAN_POINT ( 'NONE',  ( 14.97283176289962903, 21.60377111278808471, 10.49999999999999822 ) ) ;
#22776=VECTOR ( 'NONE', #24562, 1000.000000000000000 ) ;
#22779=FACE_OUTER_BOUND ( 'NONE', #3928, .T. ) ;
#22780=EDGE_LOOP ( 'NONE', ( #39294, #19940, #13211 ) ) ;
#22784=ORIENTED_EDGE ( 'NONE', *, *, #34446, .F. ) ;
#22788=EDGE_CURVE ( 'NONE', #4338, #39554, #24499, .T. ) ;
#22789=DIRECTION ( 'NONE',  ( 0.000000000000000000, 0.000000000000000000, -1.000000000000000000 ) ) ;
#22790=ADVANCED_FACE ( 'NONE', ( #14547 ), #23689, .T. ) ;
#22792=AXIS2_PLACEMENT_3D ( 'NONE', #36356, #8519, #24359 ) ;
#22794=VECTOR ( 'NONE', #5064, 1000.000000000000114 ) ;
#22795=CARTESIAN_POINT ( 'NONE',  ( -8.249569378970276645, 9.971997865784310022, 7.485646746502372828 ) ) ;
#22799=AXIS2_PLACEMENT_3D ( 'NONE', #15438, #11991, #30883 ) ;
#22801=FACE_OUTER_BOUND ( 'NONE', #12824, .T. ) ;
#22802=VERTEX_POINT ( 'NONE', #17615 ) ;
#22808=ADVANCED_FACE ( 'NONE', ( #8456 ), #27116, .T. ) ;
#22811=B_SPLINE_CURVE_WITH_KNOTS ( 'NONE', 3,
 ( #2062, #5101, #11200, #29880, #14438, #8751 ),
 .UNSPECIFIED., .F., .F.,
 ( 4, 2, 4 ),
 ( 0.000000000000000000, 0.5000000000000000000, 1.000000000000000000 ),
 .UNSPECIFIED. ) ;
#22812=ORIENTED_EDGE ( 'NONE', *, *, #5484, .F. ) ;
#22815=ORIENTED_EDGE ( 'NONE', *, *, #6787, .F. ) ;
#22817=DIRECTION ( 'NONE',  ( 0.4999999999999920064, -0.8660254037844432595, 0.000000000000000000 ) ) ;
#22819=CARTESIAN_POINT ( 'NONE',  ( -13.87104230352202094, 20.53934056656885687, 7.000000000000000000 ) ) ;
#22824=CARTESIAN_POINT ( 'NONE',  ( 6.354454053420415249, 35.54304081427981288, 11.00000000000000000 ) ) ;
#22828=CARTESIAN_POINT ( 'NONE',  ( -3.503793317224519477, 8.420815634768723967, 11.00000000000000000 ) ) ;
#22830=EDGE_LOOP ( 'NONE', ( #12636, #29844, #8813, #21928 ) ) ;
#22835=CIRCLE ( 'NONE', #33252, 0.4999999999999988898 ) ;
#22837=CARTESIAN_POINT ( 'NONE',  ( 10.44103466624280507, 32.57396620494213124, 7.499999999999997335 ) ) ;
#22838=AXIS2_PLACEMENT_3D ( 'NONE', #15335, #21825, #9048 ) ;
#22840=FACE_OUTER_BOUND ( 'NONE', #37034, .T. ) ;
#22841=CARTESIAN_POINT ( 'NONE',  ( -11.81630298851966288, 31.79381426990562787, 11.00000000000000000 ) ) ;
#22843=TOROIDAL_SURFACE ( 'NONE', #22202, 1.000000000000000000, 0.5000000000000000000 ) ;
#22845=ORIENTED_EDGE ( 'NONE', *, *, #21753, .F. ) ;
#22846=CARTESIAN_POINT ( 'NONE',  ( 8.118377661053324701, 10.47536095541698486, 7.000000000000000000 ) ) ;
#22847=DIRECTION ( 'NONE',  ( 0.2079116908177532641, -0.9781476007338069101, 0.000000000000000000 ) ) ;
#22850=FACE_OUTER_BOUND ( 'NONE', #458, .T. ) ;
#22853=ORIENTED_EDGE ( 'NONE', *, *, #944, .F. ) ;
#22856=VECTOR ( 'NONE', #38178, 1000.000000000000114 ) ;
#22858=DIRECTION ( 'NONE',  ( -0.000000000000000000, -0.000000000000000000, -1.000000000000000000 ) ) ;
#22860=ORIENTED_EDGE ( 'NONE', *, *, #12857, .T. ) ;
#22862=EDGE_LOOP ( 'NONE', ( #13286, #28832, #5786, #914 ) ) ;
#22864=CARTESIAN_POINT ( 'NONE',  ( 3.503793317224327186, 8.420815634768674229, 7.000000000000000000 ) ) ;
#22867=AXIS2_PLACEMENT_3D ( 'NONE', #28276, #10594, #6923 ) ;
#22876=VERTEX_POINT ( 'NONE', #24092 ) ;
#22880=DIRECTION ( 'NONE',  ( -1.000000000000000000, 0.000000000000000000, 0.000000000000000000 ) ) ;
#22881=PLANE ( 'NONE',  #3783 ) ;
#22886=CIRCLE ( 'NONE', #27450, 0.4999999999999995559 ) ;
#22887=ORIENTED_EDGE ( 'NONE', *, *, #9966, .T. ) ;
#22888=FACE_OUTER_BOUND ( 'NONE', #8208, .T. ) ;
#22889=CARTESIAN_POINT ( 'NONE',  ( -6.354454053420248272, 35.54304081427989814, 7.000000000000000000 ) ) ;
#22891=DIRECTION ( 'NONE',  ( 0.8090169943749430104, -0.5877852522924791323, 0.000000000000000000 ) ) ;
#22893=ADVANCED_FACE ( 'NONE', ( #39726 ), #33846, .T. ) ;
#22896=CARTESIAN_POINT ( 'NONE',  ( 5.982165713378432059, 28.55918256678898715, 7.000000000000000000 ) ) ;
#22897=EDGE_CURVE ( 'NONE', #24444, #18426, #34890, .T. ) ;
#22898=DIRECTION ( 'NONE',  ( 0.000000000000000000, -0.000000000000000000, -1.000000000000000000 ) ) ;
#22899=CARTESIAN_POINT ( 'NONE',  ( -7.713869163866016621, 10.18146832927085121, 7.500000000000000888 ) ) ;
#22900=VECTOR ( 'NONE', #26100, 1000.000000000000114 ) ;
#22901=CARTESIAN_POINT ( 'NONE',  ( -8.100578861132728292, 28.44816123811128605, 10.49999999999999822 ) ) ;
#22904=VERTEX_POINT ( 'NONE', #2564 ) ;
#22906=DIRECTION ( 'NONE',  ( 0.8660254037844437036, 0.4999999999999912292, -0.000000000000000000 ) ) ;
#22907=VECTOR ( 'NONE', #37097, 999.9999999999998863 ) ;
#22908=CARTESIAN_POINT ( 'NONE',  ( -0.4999999999999998890, 37.50000000000000711, 10.59344459855561027 ) ) ;
#22910=DIRECTION ( 'NONE',  ( 0.4067366430757888840, -0.9135454576426058626, 0.000000000000000000 ) ) ;
#22912=AXIS2_PLACEMENT_3D ( 'NONE', #27099, #30150, #36645 ) ;
#22915=( GEOMETRIC_REPRESENTATION_CONTEXT ( 3 ) GLOBAL_UNCERTAINTY_ASSIGNED_CONTEXT ( ( #13639 ) ) GLOBAL_UNIT_ASSIGNED_CONTEXT ( ( #26344, #10918, #39132 ) ) REPRESENTATION_CONTEXT ( 'NONE', 'WORKASPACE' ) );
#22920=EDGE_CURVE ( 'NONE', #33392, #27087, #18399, .T. ) ;
#22922=DIRECTION ( 'NONE',  ( -1.000000000000000000, 0.000000000000000000, 0.000000000000000000 ) ) ;
#22925=ORIENTED_EDGE ( 'NONE', *, *, #7603, .F. ) ;
#22927=VERTEX_POINT ( 'NONE', #24884 ) ;
#22930=CARTESIAN_POINT ( 'NONE',  ( -14.31603901957233838, 19.98981538725089990, 10.49999999999999822 ) ) ;
#22931=VERTEX_POINT ( 'NONE', #27732 ) ;
#22933=CARTESIAN_POINT ( 'NONE',  ( 0.000000000000000000, 0.000000000000000000, 7.000000000000000000 ) ) ;
#22935=EDGE_LOOP ( 'NONE', ( #359, #7362, #12024, #17701 ) ) ;
#22937=VERTEX_POINT ( 'NONE', #21634 ) ;
#22944=CARTESIAN_POINT ( 'NONE',  ( 13.84305327410120334, 40.15700533419733631, 10.00000000000000000 ) ) ;
#22947=AXIS2_PLACEMENT_3D ( 'NONE', #14166, #23109, #29407 ) ;
#22948=CARTESIAN_POINT ( 'NONE',  ( -5.440908595777639079, 35.94977745735568675, 9.500000000000000000 ) ) ;
#22949=ORIENTED_EDGE ( 'NONE', *, *, #11500, .T. ) ;
#22951=DIRECTION ( 'NONE',  ( -0.000000000000000000, -0.000000000000000000, -1.000000000000000000 ) ) ;
#22956=VERTEX_POINT ( 'NONE', #2754 ) ;
#22957=DIRECTION ( 'NONE',  ( 0.9510565162951544194, 0.3090169943749450643, 0.000000000000000000 ) ) ;
#22958=CARTESIAN_POINT ( 'NONE',  ( -0.4999999999999998890, 37.50000000000000711, 10.49999999999999822 ) ) ;
#22960=FACE_OUTER_BOUND ( 'NONE', #11691, .T. ) ;
#22961=DIRECTION ( 'NONE',  ( -0.000000000000000000, -0.000000000000000000, -1.000000000000000000 ) ) ;
#22967=CARTESIAN_POINT ( 'NONE',  ( 10.14060191828658120, 25.26915018278934255, 10.50000000000000000 ) ) ;
#22968=EDGE_CURVE ( 'NONE', #34846, #1082, #24290, .T. ) ;
#22969=ORIENTED_EDGE ( 'NONE', *, *, #34928, .T. ) ;
#22970=ORIENTED_EDGE ( 'NONE', *, *, #3771, .T. ) ;
#22973=CARTESIAN_POINT ( 'NONE',  ( 3.503793317224329851, 8.420815634768676006, 9.000000000000001776 ) ) ;
#22976=CARTESIAN_POINT ( 'NONE',  ( 11.11016527260166420, 31.83082137946473367, 7.000000000000000000 ) ) ;
#22977=ORIENTED_EDGE ( 'NONE', *, *, #1631, .T. ) ;
#22980=CARTESIAN_POINT ( 'NONE',  ( -12.80736835487442349, 15.68301270189233954, 7.499999999999993783 ) ) ;
#22984=ORIENTED_EDGE ( 'NONE', *, *, #28544, .T. ) ;
#22986=AXIS2_PLACEMENT_3D ( 'NONE', #23703, #36103, #15355 ) ;
#22987=CARTESIAN_POINT ( 'NONE',  ( 1.872892888448897120, -2.256054360071899634, 7.499999999999997335 ) ) ;
#22992=PLANE ( 'NONE',  #31878 ) ;
#22993=EDGE_CURVE ( 'NONE', #3128, #10038, #21243, .T. ) ;
#22995=CARTESIAN_POINT ( 'NONE',  ( 8.927394655428267711, 11.06314620770944757, 11.00000000000000000 ) ) ;
#22996=ADVANCED_FACE ( 'NONE', ( #33652 ), #36883, .F. ) ;
#22997=CARTESIAN_POINT ( 'NONE',  ( -8.315274455032252376, 10.01576150750523375, 7.500000000000000888 ) ) ;
#22999=EDGE_CURVE ( 'NONE', #6543, #38536, #2477, .T. ) ;
#23000=DIRECTION ( 'NONE',  ( 0.9135454576426059736, 0.4067366430757889395, -0.000000000000000000 ) ) ;
#23005=CARTESIAN_POINT ( 'NONE',  ( -14.57736017774144699, 22.47612012567159567, 7.000000000000000000 ) ) ;
#23009=AXIS2_PLACEMENT_3D ( 'NONE', #16666, #20725, #32714 ) ;
#23012=CARTESIAN_POINT ( 'NONE',  ( -14.42035624161469798, 26.65972665747689163, 10.59344459855566356 ) ) ;
#23014=EDGE_LOOP ( 'NONE', ( #13597, #12899, #877, #20504 ) ) ;
#23017=ORIENTED_EDGE ( 'NONE', *, *, #21784, .T. ) ;
#23019=CARTESIAN_POINT ( 'NONE',  ( -8.118377661053489902, 10.47536095541709322, 7.000000000000000000 ) ) ;
#23020=EDGE_CURVE ( 'NONE', #2159, #18499, #21916, .T. ) ;
#23022=CARTESIAN_POINT ( 'NONE',  ( 13.32168723750162975, 15.60515543615789724, 7.485646746502371940 ) ) ;
#23023=EDGE_CURVE ( 'NONE', #32239, #29026, #18008, .T. ) ;
#23024=VERTEX_POINT ( 'NONE', #3349 ) ;
#23029=ORIENTED_EDGE ( 'NONE', *, *, #16216, .T. ) ;
#23031=DIRECTION ( 'NONE',  ( 0.2876062384759567880, 0.6459741880212539478, -0.7071067811865424657 ) ) ;
#23033=ORIENTED_EDGE ( 'NONE', *, *, #37902, .T. ) ;
#23035=AXIS2_PLACEMENT_3D ( 'NONE', #38220, #1444, #25820 ) ;
#23040=AXIS2_PLACEMENT_3D ( 'NONE', #26318, #5383, #17191 ) ;
#23046=DIRECTION ( 'NONE',  ( -0.000000000000000000, -0.000000000000000000, -1.000000000000000000 ) ) ;
#23048=EDGE_CURVE ( 'NONE', #13187, #14341, #25140, .T. ) ;
#23049=CARTESIAN_POINT ( 'NONE',  ( -11.58359699910274720, 32.01076754692467574, 10.49999999999999822 ) ) ;
#23050=CARTESIAN_POINT ( 'NONE',  ( 14.31603901957230462, 19.98981538725069740, 10.50000000000000533 ) ) ;
#23052=ORIENTED_EDGE ( 'NONE', *, *, #29646, .T. ) ;
#23053=DIRECTION ( 'NONE',  ( 0.000000000000000000, 0.000000000000000000, -1.000000000000000000 ) ) ;
#23057=CARTESIAN_POINT ( 'NONE',  ( 16.72075857324119141, 7.444561356925491147, 11.00000000000000000 ) ) ;
#23064=DIRECTION ( 'NONE',  ( -0.000000000000000000, -0.000000000000000000, -1.000000000000000000 ) ) ;
#23066=VERTEX_POINT ( 'NONE', #34826 ) ;
#23069=CIRCLE ( 'NONE', #10752, 0.5000000000000004441 ) ;
#23072=EDGE_CURVE ( 'NONE', #10321, #14195, #14119, .T. ) ;
#23075=EDGE_CURVE ( 'NONE', #12629, #20052, #32313, .T. ) ;
#23076=VECTOR ( 'NONE', #26958, 999.9999999999998863 ) ;
#23081=EDGE_LOOP ( 'NONE', ( #8649, #19508, #19523, #21672, #4603 ) ) ;
#23083=CARTESIAN_POINT ( 'NONE',  ( 4.440908595777811385, 35.94977745735560859, 7.000000000000000000 ) ) ;
#23084=LINE ( 'NONE', #4601, #29656 ) ;
#23085=ORIENTED_EDGE ( 'NONE', *, *, #39152, .F. ) ;
#23089=ORIENTED_EDGE ( 'NONE', *, *, #27882, .T. ) ;
#23091=CARTESIAN_POINT ( 'NONE',  ( -14.11133924723978161, 27.61078317377194224, 7.000000000000000000 ) ) ;
#23096=DIRECTION ( 'NONE',  ( -0.000000000000000000, -0.000000000000000000, -1.000000000000000000 ) ) ;
#23097=AXIS2_PLACEMENT_3D ( 'NONE', #21970, #25609, #22165 ) ;
#23099=CIRCLE ( 'NONE', #34133, 1.000000000000002665 ) ;
#23100=AXIS2_PLACEMENT_3D ( 'NONE', #29460, #16475, #10579 ) ;
#23104=CARTESIAN_POINT ( 'NONE',  ( -14.97433423632582006, 21.61937474157331351, 7.485699520496981840 ) ) ;
#23109=DIRECTION ( 'NONE',  ( -0.000000000000000000, -0.000000000000000000, -1.000000000000000000 ) ) ;
#23111=CARTESIAN_POINT ( 'NONE',  ( -2.672146553953452575, 12.33340603770394317, 10.00000000000000000 ) ) ;
#23112=ORIENTED_EDGE ( 'NONE', *, *, #6164, .T. ) ;
#23114=DIRECTION ( 'NONE',  ( -0.000000000000000000, -0.000000000000000000, -1.000000000000000000 ) ) ;
#23115=CARTESIAN_POINT ( 'NONE',  ( -0.4999999999999998890, 37.09261900150649893, 10.99387790580546032 ) ) ;
#23117=DIRECTION ( 'NONE',  ( 0.000000000000000000, 0.000000000000000000, 1.000000000000000000 ) ) ;
#23120=PLANE ( 'NONE',  #7703 ) ;
#23125=EDGE_CURVE ( 'NONE', #38914, #35744, #37494, .T. ) ;
#23127=CARTESIAN_POINT ( 'NONE',  ( 5.002948306803792100, 36.19539921059735832, 10.49999999999999822 ) ) ;
#23128=ADVANCED_FACE ( 'NONE', ( #1658 ), #10231, .T. ) ;
#23129=ORIENTED_EDGE ( 'NONE', *, *, #10877, .T. ) ;
#23135=VERTEX_POINT ( 'NONE', #506 ) ;
#23136=CARTESIAN_POINT ( 'NONE',  ( 11.44134295108989363, 15.31698729810773152, 9.500000000000000000 ) ) ;
#23137=AXIS2_PLACEMENT_3D ( 'NONE', #6769, #15729, #13271 ) ;
#23138=CARTESIAN_POINT ( 'NONE',  ( 9.156995300982067931, 10.74712803024074503, 10.82238861112330142 ) ) ;
#23140=ORIENTED_EDGE ( 'NONE', *, *, #36449, .F. ) ;
#23144=ORIENTED_EDGE ( 'NONE', *, *, #20232, .T. ) ;
#23147=CYLINDRICAL_SURFACE ( 'NONE', #24245, 0.5000000000000004441 ) ;
#23148=FACE_OUTER_BOUND ( 'NONE', #18725, .T. ) ;
#23150=CARTESIAN_POINT ( 'NONE',  ( -14.36830325120615548, 20.48707633493503621, 7.000000000000000000 ) ) ;
#23151=ORIENTED_EDGE ( 'NONE', *, *, #15478, .T. ) ;
#23152=DIRECTION ( 'NONE',  ( -0.000000000000000000, -0.000000000000000000, 1.000000000000000000 ) ) ;
#23155=FACE_OUTER_BOUND ( 'NONE', #29230, .T. ) ;
#23157=TOROIDAL_SURFACE ( 'NONE', #10867, 1.000000000000000000, 0.5000000000000000000 ) ;
#23159=VECTOR ( 'NONE', #19985, 1000.000000000000000 ) ;
#23160=ORIENTED_EDGE ( 'NONE', *, *, #6890, .T. ) ;
#23165=CARTESIAN_POINT ( 'NONE',  ( -8.633502029282189127, 11.46765470489704342, 7.499999999999999112 ) ) ;
#23166=ORIENTED_EDGE ( 'NONE', *, *, #21935, .F. ) ;
#23167=AXIS2_PLACEMENT_3D ( 'NONE', #11124, #17229, #2585 ) ;
#23171=ADVANCED_FACE ( 'NONE', ( #37675 ), #13837, .T. ) ;
#23172=PLANE ( 'NONE',  #6876 ) ;
#23174=VERTEX_POINT ( 'NONE', #6779 ) ;
#23176=DIRECTION ( 'NONE',  ( 0.6123724356957913617, -0.3535533905932748411, -0.7071067811865496822 ) ) ;
#23177=ADVANCED_FACE ( 'NONE', ( #19181 ), #4179, .T. ) ;
#23178=CARTESIAN_POINT ( 'NONE',  ( -12.30736835487442882, 14.81698729810789672, 11.00000000000000000 ) ) ;
#23180=CARTESIAN_POINT ( 'NONE',  ( -7.014595103779441843, 35.79644522156330311, 7.000000000000000000 ) ) ;
#23181=ORIENTED_EDGE ( 'NONE', *, *, #4816, .T. ) ;
#23183=EDGE_CURVE ( 'NONE', #2015, #29633, #8301, .T. ) ;
#23184=CARTESIAN_POINT ( 'NONE',  ( -10.81260707898136708, 32.90853150812170469, 10.50000000000000533 ) ) ;
#23185=DIRECTION ( 'NONE',  ( 1.000000000000000000, 0.000000000000000000, 0.000000000000000000 ) ) ;
#23186=DIRECTION ( 'NONE',  ( 0.4999999999999920064, -0.8660254037844432595, -0.000000000000000000 ) ) ;
#23188=ORIENTED_EDGE ( 'NONE', *, *, #25127, .T. ) ;
#23190=CARTESIAN_POINT ( 'NONE',  ( 8.410254037844358876, 17.06698729810774395, 10.49999999999999822 ) ) ;
#23193=CONICAL_SURFACE ( 'NONE', #36846, 0.9999999999999986677, 0.7853981633974501664 ) ;
#23194=AXIS2_PLACEMENT_3D ( 'NONE', #25964, #20091, #10538 ) ;
#23195=LINE ( 'NONE', #31734, #12257 ) ;
#23197=ORIENTED_EDGE ( 'NONE', *, *, #28481, .T. ) ;
#23199=AXIS2_PLACEMENT_3D ( 'NONE', #22837, #22635, #37879 ) ;
#23201=CARTESIAN_POINT ( 'NONE',  ( -12.80736835487442349, 15.68301270189233954, 7.000000000000000000 ) ) ;
#23203=AXIS2_PLACEMENT_3D ( 'NONE', #24485, #30396, #27338 ) ;
#23204=DIRECTION ( 'NONE',  ( -0.8153776007405543202, 0.04273212933195244534, 0.5773502691896267303 ) ) ;
#23205=ORIENTED_EDGE ( 'NONE', *, *, #27931, .T. ) ;
#23206=ADVANCED_FACE ( 'NONE', ( #20550 ), #32943, .T. ) ;
#23207=DIRECTION ( 'NONE',  ( 0.2876062384759450197, -0.6459741880212619414, -0.7071067811865398012 ) ) ;
#23210=CARTESIAN_POINT ( 'NONE',  ( -12.80736835487441816, 15.68301270189233243, 11.00000000000000000 ) ) ;
#23214=LINE ( 'NONE', #26860, #13905 ) ;
#23215=VECTOR ( 'NONE', #30634, 1000.000000000000227 ) ;
#23217=CARTESIAN_POINT ( 'NONE',  ( 2.036571916123607551, 8.108948098542043681, 10.49999999999999822 ) ) ;
#23220=EDGE_LOOP ( 'NONE', ( #4242, #20548, #29523, #20933 ) ) ;
#23222=VECTOR ( 'NONE', #29184, 1000.000000000000000 ) ;
#23224=CARTESIAN_POINT ( 'NONE',  ( -14.12406941186437770, 26.56345723075652998, 10.96580508970279766 ) ) ;
#23231=DIRECTION ( 'NONE',  ( 1.000000000000000000, 1.734723475976809067E-15, 0.000000000000000000 ) ) ;
#23233=EDGE_CURVE ( 'NONE', #2993, #13835, #18054, .T. ) ;
#23235=CONICAL_SURFACE ( 'NONE', #31041, 1.000000000000002665, 0.7853981633974543852 ) ;
#23236=ORIENTED_EDGE ( 'NONE', *, *, #32117, .F. ) ;
#23241=ORIENTED_EDGE ( 'NONE', *, *, #21797, .T. ) ;
#23243=DIRECTION ( 'NONE',  ( -0.000000000000000000, -0.000000000000000000, 1.000000000000000000 ) ) ;
#23245=ORIENTED_EDGE ( 'NONE', *, *, #21447, .T. ) ;
#23249=VERTEX_POINT ( 'NONE', #36185 ) ;
#23252=DIRECTION ( 'NONE',  ( -0.4999999999999919509, 0.8660254037844432595, 0.000000000000000000 ) ) ;
#23253=VECTOR ( 'NONE', #13389, 1000.000000000000000 ) ;
#23254=CIRCLE ( 'NONE', #40086, 0.5000000000000000000 ) ;
#23255=CARTESIAN_POINT ( 'NONE',  ( -12.53024597560957609, 27.62278594035707613, 9.500000000000000000 ) ) ;
#23256=AXIS2_PLACEMENT_3D ( 'NONE', #26700, #23046, #38487 ) ;
#23257=EDGE_CURVE ( 'NONE', #11482, #11960, #19341, .T. ) ;
#23258=CARTESIAN_POINT ( 'NONE',  ( -2.231935796429922902, 7.666817632609298272, 7.382773698552460573 ) ) ;
#23259=LINE ( 'NONE', #23457, #19693 ) ;
#23260=DIRECTION ( 'NONE',  ( 0.5720614028176864707, -0.4156269377774609031, -0.7071067811865414665 ) ) ;
#23261=ORIENTED_EDGE ( 'NONE', *, *, #18199, .F. ) ;
#23263=DIRECTION ( 'NONE',  ( -1.000000000000000000, 0.000000000000000000, 0.000000000000000000 ) ) ;
#23264=CARTESIAN_POINT ( 'NONE',  ( -5.184280209938394002, 31.68549066217158483, 10.50000000000000355 ) ) ;
#23267=CARTESIAN_POINT ( 'NONE',  ( -14.83795255154715598, 20.43771420437966313, 10.68306085400112870 ) ) ;
#23273=DIRECTION ( 'NONE',  ( 0.9945218953682742891, 0.1045284632676437425, 0.000000000000000000 ) ) ;
#23275=ORIENTED_EDGE ( 'NONE', *, *, #32459, .T. ) ;
#23277=ORIENTED_EDGE ( 'NONE', *, *, #34625, .F. ) ;
#23279=CARTESIAN_POINT ( 'NONE',  ( 3.558056881628218981, 8.165525635826492490, 10.94611345180490503 ) ) ;
#23281=EDGE_CURVE ( 'NONE', #37730, #25929, #22811, .T. ) ;
#23283=TOROIDAL_SURFACE ( 'NONE', #9659, 1.000000000000000000, 0.5000000000000000000 ) ;
#23284=CIRCLE ( 'NONE', #21967, 0.5000000000000001110 ) ;
#23289=EDGE_CURVE ( 'NONE', #22335, #18302, #26833, .T. ) ;
#23292=DIRECTION ( 'NONE',  ( 0.07391278520358141035, -0.7032331762534025366, -0.7071067811865476838 ) ) ;
#23293=LINE ( 'NONE', #14143, #7617 ) ;
#23294=ORIENTED_EDGE ( 'NONE', *, *, #27520, .F. ) ;
#23298=EDGE_LOOP ( 'NONE', ( #33595, #21376, #17954, #29119 ) ) ;
#23301=FACE_OUTER_BOUND ( 'NONE', #35939, .T. ) ;
#23305=DIRECTION ( 'NONE',  ( -0.000000000000000000, -0.000000000000000000, -1.000000000000000000 ) ) ;
#23307=EDGE_CURVE ( 'NONE', #30940, #29040, #30291, .T. ) ;
#23308=EDGE_CURVE ( 'NONE', #22563, #11320, #27037, .T. ) ;
#23314=CARTESIAN_POINT ( 'NONE',  ( -13.86495741630578316, 28.22533134718097259, 7.202682876670049694 ) ) ;
#23315=DIRECTION ( 'NONE',  ( 0.7032331762534032027, 0.07391278520355958059, 0.7071067811865493491 ) ) ;
#23317=DIRECTION ( 'NONE',  ( -1.000000000000000000, 0.000000000000000000, 0.000000000000000000 ) ) ;
#23321=CARTESIAN_POINT ( 'NONE',  ( -8.927394655428429360, 11.06314620770957013, 7.000000000000000000 ) ) ;
#23324=DIRECTION ( 'NONE',  ( 0.5778781230734078012, 0.000000000000000000, -0.8161230758121934548 ) ) ;
#23325=FACE_OUTER_BOUND ( 'NONE', #15337, .T. ) ;
#23327=DIRECTION ( 'NONE',  ( 1.000000000000000000, 0.000000000000000000, 0.000000000000000000 ) ) ;
#23331=ADVANCED_FACE ( 'NONE', ( #11995 ), #23235, .T. ) ;
#23335=EDGE_CURVE ( 'NONE', #29633, #35208, #21344, .T. ) ;
#23337=FACE_OUTER_BOUND ( 'NONE', #21342, .T. ) ;
#23338=ORIENTED_EDGE ( 'NONE', *, *, #15074, .T. ) ;
#23340=ORIENTED_EDGE ( 'NONE', *, *, #20389, .T. ) ;
#23341=AXIS2_PLACEMENT_3D ( 'NONE', #23663, #12067, #33428 ) ;
#23345=CARTESIAN_POINT ( 'NONE',  ( 9.221287281574511496, 10.65863771052197428, 10.49999999999999822 ) ) ;
#23346=AXIS2_PLACEMENT_3D ( 'NONE', #8516, #33316, #2426 ) ;
#23347=ORIENTED_EDGE ( 'NONE', *, *, #5416, .T. ) ;
#23351=EDGE_LOOP ( 'NONE', ( #1698, #23629, #5029, #3300 ) ) ;
#23353=CARTESIAN_POINT ( 'NONE',  ( 10.47671942996444905, 33.23510584127189560, 7.339470489435492517 ) ) ;
#23354=VERTEX_POINT ( 'NONE', #2460 ) ;
#23355=B_SPLINE_CURVE_WITH_KNOTS ( 'NONE', 3,
 ( #14772, #39144, #33072, #15165, #11123, #39546 ),
 .UNSPECIFIED., .F., .F.,
 ( 4, 2, 4 ),
 ( 0.000000000000000000, 0.5000000000000000000, 1.000000000000000000 ),
 .UNSPECIFIED. ) ;
#23356=FACE_OUTER_BOUND ( 'NONE', #38022, .T. ) ;
#23359=DIRECTION ( 'NONE',  ( 0.000000000000000000, 0.000000000000000000, 1.000000000000000000 ) ) ;
#23360=ORIENTED_EDGE ( 'NONE', *, *, #1303, .F. ) ;
#23361=LINE ( 'NONE', #7714, #19768 ) ;
#23363=EDGE_CURVE ( 'NONE', #1365, #2652, #18711, .T. ) ;
#23367=AXIS2_PLACEMENT_3D ( 'NONE', #4678, #8334, #23570 ) ;
#23370=LINE ( 'NONE', #14421, #16879 ) ;
#23374=CARTESIAN_POINT ( 'NONE',  ( -6.762317648414995830, 29.93445088906605633, 10.49999999999999822 ) ) ;
#23379=CARTESIAN_POINT ( 'NONE',  ( -9.645751987030186214, 11.01237070952370622, 7.281642668398248475 ) ) ;
#23380=EDGE_LOOP ( 'NONE', ( #32029, #27939, #36794, #27487, #6071 ) ) ;
#23385=AXIS2_PLACEMENT_3D ( 'NONE', #37245, #14915, #72 ) ;
#23388=ORIENTED_EDGE ( 'NONE', *, *, #8815, .F. ) ;
#23390=DIRECTION ( 'NONE',  ( -1.000000000000000000, 0.000000000000000000, 0.000000000000000000 ) ) ;
#23391=DIRECTION ( 'NONE',  ( 0.5906904945688822295, 0.000000000000000000, -0.8068982213550660587 ) ) ;
#23395=CARTESIAN_POINT ( 'NONE',  ( -14.11133924723978161, 27.61078317377194224, 10.49999999999999822 ) ) ;
#23405=DIRECTION ( 'NONE',  ( -1.000000000000000000, 0.000000000000000000, 0.000000000000000000 ) ) ;
#23410=AXIS2_PLACEMENT_3D ( 'NONE', #31502, #25595, #3665 ) ;
#23411=CARTESIAN_POINT ( 'NONE',  ( -3.585575659063838572, 32.39727978755421134, 10.75000000000000888 ) ) ;
#23414=CIRCLE ( 'NONE', #33810, 0.5000000000000004441 ) ;
#23415=EDGE_CURVE ( 'NONE', #39789, #19274, #33628, .T. ) ;
#23417=CARTESIAN_POINT ( 'NONE',  ( 12.30736835487432579, 14.81698729810772619, 7.000000000000000000 ) ) ;
#23418=CARTESIAN_POINT ( 'NONE',  ( -13.09742388243079070, 16.09289933416735963, 10.49999999999999822 ) ) ;
#23421=ORIENTED_EDGE ( 'NONE', *, *, #30913, .F. ) ;
#23428=VECTOR ( 'NONE', #29206, 1000.000000000000000 ) ;
#23429=ORIENTED_EDGE ( 'NONE', *, *, #10603, .T. ) ;
#23433=DIRECTION ( 'NONE',  ( 1.000000000000000000, 0.000000000000000000, 0.000000000000000000 ) ) ;
#23437=CARTESIAN_POINT ( 'NONE',  ( -7.611215932167762155, 18.68301270189229513, 9.000000000000001776 ) ) ;
#23443=EDGE_CURVE ( 'NONE', #257, #4300, #22132, .T. ) ;
#23444=EDGE_LOOP ( 'NONE', ( #14145, #27083, #13669 ) ) ;
#23447=CIRCLE ( 'NONE', #33808, 0.5000000000000004441 ) ;
#23450=ORIENTED_EDGE ( 'NONE', *, *, #4405, .T. ) ;
#23456=FACE_OUTER_BOUND ( 'NONE', #11928, .T. ) ;
#23457=CARTESIAN_POINT ( 'NONE',  ( 7.111215932167702647, 17.81698729810774751, 9.000000000000001776 ) ) ;
#23459=ORIENTED_EDGE ( 'NONE', *, *, #27420, .F. ) ;
#23465=CARTESIAN_POINT ( 'NONE',  ( -6.354454053420248272, 35.54304081427989814, 7.000000000000000000 ) ) ;
#23468=AXIS2_PLACEMENT_3D ( 'NONE', #5072, #21315, #12166 ) ;
#23476=ORIENTED_EDGE ( 'NONE', *, *, #23308, .T. ) ;
#23478=CARTESIAN_POINT ( 'NONE',  ( -0.5000000000000005551, 31.00000000000000355, 9.000000000000001776 ) ) ;
#23484=ORIENTED_EDGE ( 'NONE', *, *, #8409, .T. ) ;
#23486=CARTESIAN_POINT ( 'NONE',  ( 15.00099999999999945, 33.00000000000000000, 10.00000000000000000 ) ) ;
#23487=VECTOR ( 'NONE', #23588, 1000.000000000000000 ) ;
#23489=EDGE_CURVE ( 'NONE', #18534, #490, #28142, .T. ) ;
#23491=ORIENTED_EDGE ( 'NONE', *, *, #20581, .T. ) ;
#23495=DIRECTION ( 'NONE',  ( -0.8090169943749504489, -0.5877852522924690293, 0.000000000000000000 ) ) ;
#23496=FILL_AREA_STYLE_COLOUR ( '', #17757 ) ;
#23499=AXIS2_PLACEMENT_3D ( 'NONE', #26458, #4526, #14270 ) ;
#23501=CARTESIAN_POINT ( 'NONE',  ( -2.421689871081829537, 8.701977744317861863, 7.499999999999997335 ) ) ;
#23502=ADVANCED_FACE ( 'NONE', ( #37774 ), #15242, .F. ) ;
#23503=CARTESIAN_POINT ( 'NONE',  ( 6.492361549287938516, 35.85278612139531162, 10.87262190629436986 ) ) ;
#23504=DIRECTION ( 'NONE',  ( -0.000000000000000000, -0.000000000000000000, -1.000000000000000000 ) ) ;
#23511=CARTESIAN_POINT ( 'NONE',  ( 14.50767453556300701, 21.81310552875920550, 10.66666666666667140 ) ) ;
#23515=CARTESIAN_POINT ( 'NONE',  ( 21.98892638600344895, 13.77082694162504417, 10.00000000000000000 ) ) ;
#23516=ORIENTED_EDGE ( 'NONE', *, *, #20452, .T. ) ;
#23518=AXIS2_PLACEMENT_3D ( 'NONE', #35322, #7275, #16643 ) ;
#23525=DIRECTION ( 'NONE',  ( -0.6691306063588569053, 0.7431448254773954654, 0.000000000000000000 ) ) ;
#23533=EDGE_CURVE ( 'NONE', #24240, #15902, #36983, .T. ) ;
#23534=ORIENTED_EDGE ( 'NONE', *, *, #14923, .T. ) ;
#23537=VERTEX_POINT ( 'NONE', #3253 ) ;
#23538=EDGE_CURVE ( 'NONE', #34288, #14430, #1979, .T. ) ;
#23542=FACE_OUTER_BOUND ( 'NONE', #9398, .T. ) ;
#23543=AXIS2_PLACEMENT_3D ( 'NONE', #9153, #27840, #8756 ) ;
#23547=VERTEX_POINT ( 'NONE', #3845 ) ;
#23552=VERTEX_POINT ( 'NONE', #38376 ) ;
#23553=DIRECTION ( 'NONE',  ( 0.9510565162951544194, 0.3090169943749449533, -0.000000000000000000 ) ) ;
#23554=CARTESIAN_POINT ( 'NONE',  ( -7.354454053420251824, 35.54304081427989814, 7.000000000000000000 ) ) ;
#23555=EDGE_CURVE ( 'NONE', #1674, #959, #29432, .T. ) ;
#23556=CIRCLE ( 'NONE', #33940, 0.4999999999999995559 ) ;
#23558=EDGE_CURVE ( 'NONE', #29828, #19377, #36859, .T. ) ;
#23559=LINE ( 'NONE', #27204, #6452 ) ;
#23561=ADVANCED_FACE ( 'NONE', ( #16246 ), #10149, .F. ) ;
#23562=LINE ( 'NONE', #7507, #13908 ) ;
#23569=DIRECTION ( 'NONE',  ( 0.000000000000000000, 0.000000000000000000, -1.000000000000000000 ) ) ;
#23570=DIRECTION ( 'NONE',  ( 1.000000000000000000, 0.000000000000000000, 0.000000000000000000 ) ) ;
#23573=DIRECTION ( 'NONE',  ( 0.000000000000000000, 0.000000000000000000, 1.000000000000000000 ) ) ;
#23574=DIRECTION ( 'NONE',  ( 0.2079116908177535972, -0.9781476007338069101, 1.734723475976807292E-15 ) ) ;
#23576=AXIS2_PLACEMENT_3D ( 'NONE', #616, #18902, #22534 ) ;
#23579=DIRECTION ( 'NONE',  ( 0.1045284632676422437, -0.9945218953682746221, 0.000000000000000000 ) ) ;
#23580=EDGE_LOOP ( 'NONE', ( #30933, #38657, #39638, #40008 ) ) ;
#23583=DIRECTION ( 'NONE',  ( -0.3090169943749573322, -0.9510565162951504226, 0.000000000000000000 ) ) ;
#23586=EDGE_CURVE ( 'NONE', #20973, #2015, #12209, .T. ) ;
#23588=DIRECTION ( 'NONE',  ( 0.9135454576426059736, 0.4067366430757887730, 0.000000000000000000 ) ) ;
#23589=EDGE_LOOP ( 'NONE', ( #2116, #27883, #15300, #37639 ) ) ;
#23591=DIRECTION ( 'NONE',  ( 0.5720614028176860266, 0.4156269377774551299, -0.7071067811865451302 ) ) ;
#23592=CARTESIAN_POINT ( 'NONE',  ( -14.81329996725647469, 19.93755115561707569, 11.00000000000000000 ) ) ;
#23593=CARTESIAN_POINT ( 'NONE',  ( -2.629601561899601592, 7.723830143584057062, 10.49999999999999822 ) ) ;
#23594=ORIENTED_EDGE ( 'NONE', *, *, #30569, .F. ) ;
#23596=CARTESIAN_POINT ( 'NONE',  ( -5.478580155932212925, 36.03438916679318282, 10.99387789255783154 ) ) ;
#23597=ORIENTED_EDGE ( 'NONE', *, *, #35310, .T. ) ;
#23601=EDGE_LOOP ( 'NONE', ( #20152, #32135, #38606 ) ) ;
#23608=VERTEX_POINT ( 'NONE', #35130 ) ;
#23611=CARTESIAN_POINT ( 'NONE',  ( -8.072173610822130030, 9.857023699286527219, 7.382773698552463237 ) ) ;
#23617=FACE_OUTER_BOUND ( 'NONE', #35019, .T. ) ;
#23618=FACE_OUTER_BOUND ( 'NONE', #22528, .T. ) ;
#23620=ORIENTED_EDGE ( 'NONE', *, *, #10314, .F. ) ;
#23625=CARTESIAN_POINT ( 'NONE',  ( -8.410254037844435260, 17.06698729810786475, 10.50000000000000355 ) ) ;
#23629=ORIENTED_EDGE ( 'NONE', *, *, #24764, .T. ) ;
#23633=CARTESIAN_POINT ( 'NONE',  ( -5.400683141673551901, 15.91724817395922997, 9.000000000000001776 ) ) ;
#23634=AXIS2_PLACEMENT_3D ( 'NONE', #30203, #1984, #30000 ) ;
#23638=ORIENTED_EDGE ( 'NONE', *, *, #35182, .F. ) ;
#23640=ADVANCED_FACE ( 'NONE', ( #19684 ), #798, .T. ) ;
#23641=CARTESIAN_POINT ( 'NONE',  ( -8.118377661053488126, 10.47536095541708967, 10.99999999999999289 ) ) ;
#23647=EDGE_CURVE ( 'NONE', #10152, #4297, #25780, .T. ) ;
#23651=EDGE_CURVE ( 'NONE', #31096, #29068, #7283, .T. ) ;
#23653=CONICAL_SURFACE ( 'NONE', #11331, 1.000000000000005995, 0.7853981633974496113 ) ;
#23654=CARTESIAN_POINT ( 'NONE',  ( 14.84160187385922036, 20.32586711126977619, 7.500000000000010658 ) ) ;
#23658=DIRECTION ( 'NONE',  ( 0.1045284632676437703, -0.9945218953682745111, -0.000000000000000000 ) ) ;
#23661=DIRECTION ( 'NONE',  ( 1.000000000000000000, 0.000000000000000000, 0.000000000000000000 ) ) ;
#23662=ADVANCED_FACE ( 'NONE', ( #4451 ), #7685, .T. ) ;
#23663=CARTESIAN_POINT ( 'NONE',  ( 14.47283171447379502, 21.48159823030311344, 9.000000000000001776 ) ) ;
#23665=DIRECTION ( 'NONE',  ( 0.3535533905932642940, 0.6123724356958055726, -0.7071067811865426878 ) ) ;
#23666=CARTESIAN_POINT ( 'NONE',  ( -14.75678334372862466, 20.44624543189450705, 10.82238861112329609 ) ) ;
#23668=CARTESIAN_POINT ( 'NONE',  ( -5.473344025737330476, 14.11593743010433855, 10.50000000000000000 ) ) ;
#23672=CARTESIAN_POINT ( 'NONE',  ( -11.33320880805449526, 31.58310643763908487, 10.66666666666665897 ) ) ;
#23674=ORIENTED_EDGE ( 'NONE', *, *, #20452, .F. ) ;
#23675=DIRECTION ( 'NONE',  ( 0.000000000000000000, 0.000000000000000000, -1.000000000000000000 ) ) ;
#23685=ORIENTED_EDGE ( 'NONE', *, *, #2172, .T. ) ;
#23689=PLANE ( 'NONE',  #17392 ) ;
#23690=CIRCLE ( 'NONE', #17208, 15.00000000000000000 ) ;
#23693=ADVANCED_FACE ( 'NONE', ( #1608 ), #26381, .T. ) ;
#23695=VECTOR ( 'NONE', #23907, 1000.000000000000227 ) ;
#23698=CARTESIAN_POINT ( 'NONE',  ( -13.47830981910552772, 21.58612669357095015, 9.500000000000000000 ) ) ;
#23699=ADVANCED_FACE ( 'NONE', ( #32079 ), #32290, .T. ) ;
#23700=LINE ( 'NONE', #2171, #6045 ) ;
#23701=LINE ( 'NONE', #5607, #26504 ) ;
#23702=VERTEX_POINT ( 'NONE', #13181 ) ;
#23703=CARTESIAN_POINT ( 'NONE',  ( 13.94482798346721175, 26.50521816028912525, 7.000000000000000000 ) ) ;
#23704=CONICAL_SURFACE ( 'NONE', #6185, 0.4999999999999947264, 0.7853981633974468357 ) ;
#23705=CARTESIAN_POINT ( 'NONE',  ( 6.392125613574994425, 35.62765252371730895, 10.99387789255783687 ) ) ;
#23708=DIRECTION ( 'NONE',  ( -0.9781476007338070211, -0.2079116908177534029, 0.000000000000000000 ) ) ;
#23711=EDGE_CURVE ( 'NONE', #10646, #3986, #25834, .T. ) ;
#23713=CARTESIAN_POINT ( 'NONE',  ( -8.927394655428429360, 11.06314620770957013, 7.000000000000000000 ) ) ;
#23714=CARTESIAN_POINT ( 'NONE',  ( -6.354454053420243831, 35.54304081427989814, 7.000000000000000000 ) ) ;
#23717=FACE_OUTER_BOUND ( 'NONE', #7598, .T. ) ;
#23718=VECTOR ( 'NONE', #24308, 1000.000000000000114 ) ;
#23719=EDGE_LOOP ( 'NONE', ( #20790, #449, #1182, #34687 ) ) ;
#23721=CARTESIAN_POINT ( 'NONE',  ( 6.607858460703812220, 34.88289976392060510, 10.50000000000000000 ) ) ;
#23726=DIRECTION ( 'NONE',  ( -0.000000000000000000, -0.000000000000000000, -1.000000000000000000 ) ) ;
#23727=DIRECTION ( 'NONE',  ( 1.000000000000000000, 6.938893903907210234E-15, 0.000000000000000000 ) ) ;
#23733=ORIENTED_EDGE ( 'NONE', *, *, #24297, .F. ) ;
#23735=VERTEX_POINT ( 'NONE', #13992 ) ;
#23736=EDGE_CURVE ( 'NONE', #34769, #7567, #13789, .T. ) ;
#23737=CYLINDRICAL_SURFACE ( 'NONE', #17673, 15.00000000000000000 ) ;
#23739=LINE ( 'NONE', #14997, #13446 ) ;
#23740=DIRECTION ( 'NONE',  ( -0.9510565162951543083, -0.3090169943749450088, -0.000000000000000000 ) ) ;
#23741=ORIENTED_EDGE ( 'NONE', *, *, #28988, .F. ) ;
#23742=AXIS2_PLACEMENT_3D ( 'NONE', #3880, #1043, #28063 ) ;
#23744=ORIENTED_EDGE ( 'NONE', *, *, #5515, .T. ) ;
#23746=AXIS2_PLACEMENT_3D ( 'NONE', #32053, #37004, #16221 ) ;
#23750=CARTESIAN_POINT ( 'NONE',  ( 10.52439982978253674, 33.18839767067679958, 7.382773698552464126 ) ) ;
#23752=CARTESIAN_POINT ( 'NONE',  ( 14.97277451176449325, 21.48159783397873923, 10.49999999999999822 ) ) ;
#23753=DIRECTION ( 'NONE',  ( 0.2079116908177533474, -0.9781476007338067991, 0.000000000000000000 ) ) ;
#23755=ORIENTED_EDGE ( 'NONE', *, *, #159, .F. ) ;
#23758=CYLINDRICAL_SURFACE ( 'NONE', #22792, 0.4999999999999998335 ) ;
#23759=CARTESIAN_POINT ( 'NONE',  ( 2.629601561899395534, 7.723830143584016206, 7.000000000000000000 ) ) ;
#23760=EDGE_CURVE ( 'NONE', #15678, #2130, #23901, .T. ) ;
#23764=DIRECTION ( 'NONE',  ( 0.000000000000000000, 0.000000000000000000, -1.000000000000000000 ) ) ;
#23765=CARTESIAN_POINT ( 'NONE',  ( -2.501562340374943183, 7.696614566897864940, 10.49999999999999822 ) ) ;
#23768=VECTOR ( 'NONE', #1645, 1000.000000000000000 ) ;
#23769=DIRECTION ( 'NONE',  ( 0.1045284632676436315, -0.9945218953682742891, 0.000000000000000000 ) ) ;
#23771=AXIS2_PLACEMENT_3D ( 'NONE', #36870, #12477, #39906 ) ;
#23774=CIRCLE ( 'NONE', #2294, 15.00000000000000000 ) ;
#23775=CARTESIAN_POINT ( 'NONE',  ( -14.84160187385924523, 20.32586711126994672, 7.000000000000000000 ) ) ;
#23776=ORIENTED_EDGE ( 'NONE', *, *, #18248, .T. ) ;
#23779=CARTESIAN_POINT ( 'NONE',  ( 13.22516817658079802, 40.70288237343621063, 11.00000000000000000 ) ) ;
#23780=ADVANCED_FACE ( 'NONE', ( #36534 ), #29634, .T. ) ;
#23781=FACE_OUTER_BOUND ( 'NONE', #20836, .T. ) ;
#23785=EDGE_CURVE ( 'NONE', #23843, #3978, #11576, .T. ) ;
#23786=DIRECTION ( 'NONE',  ( 0.000000000000000000, 0.000000000000000000, 1.000000000000000000 ) ) ;
#23787=DIRECTION ( 'NONE',  ( -0.9945218953682744001, -0.1045284632676436315, 0.000000000000000000 ) ) ;
#23792=ORIENTED_EDGE ( 'NONE', *, *, #14509, .T. ) ;
#23796=ORIENTED_EDGE ( 'NONE', *, *, #21849, .F. ) ;
#23803=CARTESIAN_POINT ( 'NONE',  ( -10.06946225350398194, 32.23940090176283491, 7.500000000000005329 ) ) ;
#23804=ORIENTED_EDGE ( 'NONE', *, *, #1941, .F. ) ;
#23808=ADVANCED_FACE ( 'NONE', ( #39577 ), #14181, .T. ) ;
#23814=LINE ( 'NONE', #33176, #33266 ) ;
#23816=ORIENTED_EDGE ( 'NONE', *, *, #38451, .F. ) ;
#23818=ORIENTED_EDGE ( 'NONE', *, *, #8407, .F. ) ;
#23821=CYLINDRICAL_SURFACE ( 'NONE', #30213, 0.5000000000000001110 ) ;
#23827=DIRECTION ( 'NONE',  ( -0.000000000000000000, -0.000000000000000000, -1.000000000000000000 ) ) ;
#23829=ADVANCED_FACE ( 'NONE', ( #23542 ), #17666, .T. ) ;
#23830=DIRECTION ( 'NONE',  ( 0.9510565162951538642, 0.3090169943749465631, 0.000000000000000000 ) ) ;
#23831=VECTOR ( 'NONE', #27881, 999.9999999999998863 ) ;
#23832=AXIS2_PLACEMENT_3D ( 'NONE', #749, #36931, #9097 ) ;
#23837=ORIENTED_EDGE ( 'NONE', *, *, #29653, .T. ) ;
#23842=VECTOR ( 'NONE', #10661, 1000.000000000000000 ) ;
#23843=VERTEX_POINT ( 'NONE', #26588 ) ;
#23851=CARTESIAN_POINT ( 'NONE',  ( 8.368303251206119953, 20.48707633493483371, 9.000000000000001776 ) ) ;
#23853=AXIS2_PLACEMENT_3D ( 'NONE', #30087, #14849, #36386 ) ;
#23854=AXIS2_PLACEMENT_3D ( 'NONE', #1967, #14544, #18006 ) ;
#23855=CARTESIAN_POINT ( 'NONE',  ( -2.369380564245688436, 7.688150949816208168, 7.455686640544898935 ) ) ;
#23858=ORIENTED_EDGE ( 'NONE', *, *, #37201, .T. ) ;
#23860=CYLINDRICAL_SURFACE ( 'NONE', #10571, 0.5000000000000002220 ) ;
#23861=DIRECTION ( 'NONE',  ( 1.000000000000000000, 0.000000000000000000, 0.000000000000000000 ) ) ;
#23864=DIRECTION ( 'NONE',  ( 1.000000000000000000, 0.000000000000000000, 0.000000000000000000 ) ) ;
#23865=CARTESIAN_POINT ( 'NONE',  ( -14.36830325120615903, 20.48707633493503621, 11.00000000000000355 ) ) ;
#23869=EDGE_LOOP ( 'NONE', ( #654, #56, #8480, #17540 ) ) ;
#23872=CARTESIAN_POINT ( 'NONE',  ( -9.593266739736645121, 18.11602540378452986, 10.50000000000000000 ) ) ;
#23874=EDGE_LOOP ( 'NONE', ( #20136, #35527, #40126 ) ) ;
#23878=CARTESIAN_POINT ( 'NONE',  ( -6.354454053420243831, 35.54304081427989814, 7.000000000000000000 ) ) ;
#23885=VERTEX_POINT ( 'NONE', #2215 ) ;
#23887=CARTESIAN_POINT ( 'NONE',  ( 8.927394655428274817, 11.06314620770945290, 7.000000000000000000 ) ) ;
#23894=AXIS2_PLACEMENT_3D ( 'NONE', #5749, #30935, #34383 ) ;
#23895=DIRECTION ( 'NONE',  ( 0.8386705679454212747, -0.5446390350150315252, 0.000000000000000000 ) ) ;
#23897=ADVANCED_FACE ( 'NONE', ( #7894 ), #8706, .T. ) ;
#23899=CARTESIAN_POINT ( 'NONE',  ( -8.472151273871419974, 28.78272654129072095, 10.49999999999999822 ) ) ;
#23901=CIRCLE ( 'NONE', #6365, 0.4999999999999997780 ) ;
#23902=ORIENTED_EDGE ( 'NONE', *, *, #14241, .T. ) ;
#23903=CARTESIAN_POINT ( 'NONE',  ( 14.96930490892014554, 21.54088032874971859, 7.500000000000010658 ) ) ;
#23904=CARTESIAN_POINT ( 'NONE',  ( 6.832768599201303417, 35.70122713809256254, 10.49999999999999822 ) ) ;
#23905=CARTESIAN_POINT ( 'NONE',  ( -1.547498115756908321, 8.004992253133190516, 7.000000000000000000 ) ) ;
#23907=DIRECTION ( 'NONE',  ( 0.1045284632676436176, -0.9945218953682742891, -0.000000000000000000 ) ) ;
#23910=DIRECTION ( 'NONE',  ( -0.000000000000000000, -0.000000000000000000, -1.000000000000000000 ) ) ;
#23911=DIRECTION ( 'NONE',  ( 1.000000000000000000, 0.000000000000000000, 0.000000000000000000 ) ) ;
#23912=DIRECTION ( 'NONE',  ( 1.000000000000000000, 0.000000000000000000, 0.000000000000000000 ) ) ;
#23915=VECTOR ( 'NONE', #13646, 1000.000000000000000 ) ;
#23917=DIRECTION ( 'NONE',  ( -0.9945218953682746221, -0.1045284632676422437, -0.000000000000000000 ) ) ;
#23918=CIRCLE ( 'NONE', #13528, 1.000000000000000222 ) ;
#23919=ORIENTED_EDGE ( 'NONE', *, *, #11339, .F. ) ;
#23921=DIRECTION ( 'NONE',  ( -0.000000000000000000, -0.000000000000000000, -1.000000000000000000 ) ) ;
#23922=EDGE_CURVE ( 'NONE', #27126, #12690, #23739, .T. ) ;
#23923=CARTESIAN_POINT ( 'NONE',  ( 8.843266739736574067, 16.81698729810774395, 10.00000000000000000 ) ) ;
#23930=LINE ( 'NONE', #2400, #23215 ) ;
#23938=ORIENTED_EDGE ( 'NONE', *, *, #35340, .F. ) ;
#23940=ORIENTED_EDGE ( 'NONE', *, *, #39678, .T. ) ;
#23942=EDGE_CURVE ( 'NONE', #22931, #16537, #33100, .T. ) ;
#23943=CARTESIAN_POINT ( 'NONE',  ( -3.503793317224517700, 8.420815634768727520, 9.000000000000001776 ) ) ;
#23944=ADVANCED_FACE ( 'NONE', ( #20900 ), #33303, .T. ) ;
#23949=AXIS2_PLACEMENT_3D ( 'NONE', #11534, #23921, #27171 ) ;
#23950=EDGE_LOOP ( 'NONE', ( #29116, #21767, #18842, #34859 ) ) ;
#23955=DIRECTION ( 'NONE',  ( -0.8090169943749426773, 0.5877852522924796874, 0.000000000000000000 ) ) ;
#23956=CARTESIAN_POINT ( 'NONE',  ( -6.654030453887829211, 35.94335816374515247, 7.500000000000000888 ) ) ;
#23957=CARTESIAN_POINT ( 'NONE',  ( 12.05736835487432579, 14.38397459621550567, 11.00000000000000000 ) ) ;
#23958=ORIENTED_EDGE ( 'NONE', *, *, #20844, .F. ) ;
#23960=CARTESIAN_POINT ( 'NONE',  ( 12.80736835487433289, 15.68301270189216545, 7.000000000000000000 ) ) ;
#23963=ADVANCED_FACE ( 'NONE', ( #30243 ), #2412, .T. ) ;
#23966=ORIENTED_EDGE ( 'NONE', *, *, #12614, .T. ) ;
#23969=DIRECTION ( 'NONE',  ( -0.2185080122244173473, -0.6724985119639624864, -0.7071067811865404673 ) ) ;
#23971=CARTESIAN_POINT ( 'NONE',  ( 21.24426311945340373, 15.07158936841588215, 11.00000000000000000 ) ) ;
#23974=VECTOR ( 'NONE', #19204, 999.9999999999998863 ) ;
#23977=CARTESIAN_POINT ( 'NONE',  ( -1.000000000000000000, 37.00000000000000711, 7.000000000000000000 ) ) ;
#23979=EDGE_LOOP ( 'NONE', ( #29031, #16778, #31429, #10071, #3540 ) ) ;
#23980=AXIS2_PLACEMENT_3D ( 'NONE', #20518, #30462, #2229 ) ;
#23982=DIRECTION ( 'NONE',  ( 0.000000000000000000, 0.000000000000000000, 1.000000000000000000 ) ) ;
#23983=CARTESIAN_POINT ( 'NONE',  ( -12.29179778625728403, 14.31343464431660628, 10.49999999999999822 ) ) ;
#23984=CARTESIAN_POINT ( 'NONE',  ( 5.237540274239915306, 35.49300472853430222, 7.500000000000000888 ) ) ;
#23987=CARTESIAN_POINT ( 'NONE',  ( -10.44103466624267540, 32.57396620494226624, 11.00000000000000000 ) ) ;
#23988=PLANE ( 'NONE',  #23853 ) ;
#23989=ADVANCED_FACE ( 'NONE', ( #24734 ), #6443, .T. ) ;
#23990=ORIENTED_EDGE ( 'NONE', *, *, #4044, .F. ) ;
#23992=DIRECTION ( 'NONE',  ( 0.9945218953682730678, -0.1045284632676569819, 0.000000000000000000 ) ) ;
#23993=ORIENTED_EDGE ( 'NONE', *, *, #37086, .T. ) ;
#23998=DIRECTION ( 'NONE',  ( -0.5254827454987676116, -0.4731467892558093857, -0.7071067811865447972 ) ) ;
#24001=AXIS2_PLACEMENT_3D ( 'NONE', #18175, #2727, #30955 ) ;
#24002=CARTESIAN_POINT ( 'NONE',  ( 4.000124606132156480, 8.490627681068716015, 10.49999999999999822 ) ) ;
#24005=DIRECTION ( 'NONE',  ( 0.4446959099295487161, 0.6847716512521470067, 0.5773502691896305050 ) ) ;
#24006=AXIS2_PLACEMENT_3D ( 'NONE', #10509, #4414, #10111 ) ;
#24007=EDGE_CURVE ( 'NONE', #14195, #22764, #14556, .T. ) ;
#24010=EDGE_CURVE ( 'NONE', #2130, #16315, #360, .T. ) ;
#24016=VERTEX_POINT ( 'NONE', #18452 ) ;
#24018=EDGE_LOOP ( 'NONE', ( #21808, #2511, #17354, #31506 ) ) ;
#24020=VECTOR ( 'NONE', #25791, 1000.000000000000000 ) ;
#24023=LINE ( 'NONE', #36417, #2352 ) ;
#24027=ORIENTED_EDGE ( 'NONE', *, *, #7045, .T. ) ;
#24031=CARTESIAN_POINT ( 'NONE',  ( 13.53280532430061989, 27.77329351534933721, 10.66666666666666607 ) ) ;
#24032=ORIENTED_EDGE ( 'NONE', *, *, #32599, .F. ) ;
#24036=LINE ( 'NONE', #33196, #27429 ) ;
#24044=ADVANCED_FACE ( 'NONE', ( #15596 ), #21490, .F. ) ;
#24046=ORIENTED_EDGE ( 'NONE', *, *, #30399, .T. ) ;
#24050=ORIENTED_EDGE ( 'NONE', *, *, #20389, .F. ) ;
#24052=CARTESIAN_POINT ( 'NONE',  ( 4.984135866956514782, 36.15314577889351000, 7.000000000000000000 ) ) ;
#24053=DIRECTION ( 'NONE',  ( -1.224646799147351235E-16, 1.000000000000000000, 0.000000000000000000 ) ) ;
#24054=AXIS2_PLACEMENT_3D ( 'NONE', #37835, #22387, #10008 ) ;
#24055=CARTESIAN_POINT ( 'NONE',  ( 11.48173768534036121, 32.16538668264416145, 10.49999999999999822 ) ) ;
#24056=DIRECTION ( 'NONE',  ( -0.1045284632676422437, 0.9945218953682746221, 0.000000000000000000 ) ) ;
#24057=ADVANCED_FACE ( 'NONE', ( #18255 ), #156, .T. ) ;
#24059=EDGE_CURVE ( 'NONE', #19420, #22904, #18079, .T. ) ;
#24063=DIRECTION ( 'NONE',  ( 0.9945218953682729568, -0.1045284632676570929, -0.000000000000000000 ) ) ;
#24064=DIRECTION ( 'NONE',  ( -0.4067366430758009299, -0.9135454576426005335, 0.000000000000000000 ) ) ;
#24066=AXIS2_PLACEMENT_3D ( 'NONE', #16265, #15463, #37397 ) ;
#24070=ORIENTED_EDGE ( 'NONE', *, *, #37352, .T. ) ;
#24075=ORIENTED_EDGE ( 'NONE', *, *, #20355, .T. ) ;
#24076=CARTESIAN_POINT ( 'NONE',  ( -14.96161608456797687, 21.61429412723690291, 10.49999999999999822 ) ) ;
#24077=VERTEX_POINT ( 'NONE', #31434 ) ;
#24079=FACE_OUTER_BOUND ( 'NONE', #28316, .T. ) ;
#24081=DIRECTION ( 'NONE',  ( 0.000000000000000000, 0.000000000000000000, -1.000000000000000000 ) ) ;
#24082=AXIS2_PLACEMENT_3D ( 'NONE', #4720, #10615, #36007 ) ;
#24087=VERTEX_POINT ( 'NONE', #39974 ) ;
#24089=VECTOR ( 'NONE', #22789, 1000.000000000000000 ) ;
#24092=CARTESIAN_POINT ( 'NONE',  ( 1.828660225305861919, 9.087095699275852922, 10.50000000000000000 ) ) ;
#24096=DIRECTION ( 'NONE',  ( -0.7431448254773862505, 0.6691306063588670083, 0.000000000000000000 ) ) ;
#24098=CIRCLE ( 'NONE', #24728, 15.00000000000000000 ) ;
#24102=LINE ( 'NONE', #17827, #32064 ) ;
#24107=CIRCLE ( 'NONE', #29212, 0.5000000000000002220 ) ;
#24108=LINE ( 'NONE', #5425, #23718 ) ;
#24109=FACE_OUTER_BOUND ( 'NONE', #12915, .T. ) ;
#24110=DIRECTION ( 'NONE',  ( 1.000000000000000000, 0.000000000000000000, 0.000000000000000000 ) ) ;
#24111=PLANE ( 'NONE',  #25776 ) ;
#24112=DIRECTION ( 'NONE',  ( 0.000000000000000000, -0.000000000000000000, -1.000000000000000000 ) ) ;
#24113=FACE_OUTER_BOUND ( 'NONE', #34834, .T. ) ;
#24115=DIRECTION ( 'NONE',  ( -0.2185080122244104361, 0.6724985119639612652, -0.7071067811865437980 ) ) ;
#24116=ORIENTED_EDGE ( 'NONE', *, *, #18557, .T. ) ;
#24118=DIRECTION ( 'NONE',  ( -0.000000000000000000, -0.000000000000000000, 1.000000000000000000 ) ) ;
#24119=CARTESIAN_POINT ( 'NONE',  ( -13.81877807188819851, 20.04207961888471345, 9.500000000000000000 ) ) ;
#24120=CIRCLE ( 'NONE', #20884, 0.5000000000000004441 ) ;
#24124=ORIENTED_EDGE ( 'NONE', *, *, #39823, .T. ) ;
#24125=LINE ( 'NONE', #36521, #25047 ) ;
#24131=LINE ( 'NONE', #39167, #3700 ) ;
#24133=ORIENTED_EDGE ( 'NONE', *, *, #31693, .T. ) ;
#24136=VERTEX_POINT ( 'NONE', #18847 ) ;
#24137=CARTESIAN_POINT ( 'NONE',  ( -7.766013557953293400, 28.81973365084998306, 10.50000000000000000 ) ) ;
#24142=EDGE_CURVE ( 'NONE', #39323, #659, #37533, .T. ) ;
#24143=VERTEX_POINT ( 'NONE', #31045 ) ;
#24144=CIRCLE ( 'NONE', #799, 0.5000000000000003331 ) ;
#24146=ORIENTED_EDGE ( 'NONE', *, *, #38192, .F. ) ;
#24147=EDGE_CURVE ( 'NONE', #23843, #22927, #12739, .T. ) ;
#24148=CARTESIAN_POINT ( 'NONE',  ( 13.28503138821879581, 15.53523575316139649, 7.000000000000000000 ) ) ;
#24149=DIRECTION ( 'NONE',  ( -1.000000000000000000, 0.000000000000000000, 0.000000000000000000 ) ) ;
#24150=CONICAL_SURFACE ( 'NONE', #23518, 1.000000000000007772, 0.7853981633974554954 ) ;
#24151=PLANE ( 'NONE',  #39528 ) ;
#24152=EDGE_LOOP ( 'NONE', ( #29542, #35751, #20512 ) ) ;
#24155=CARTESIAN_POINT ( 'NONE',  ( -0.4999999999999950040, -6.123233995736694545E-17, 11.00000000000000000 ) ) ;
#24156=LINE ( 'NONE', #1837, #17586 ) ;
#24162=CARTESIAN_POINT ( 'NONE',  ( 8.412270287199559604, 10.07085245822950981, 10.50000000000000000 ) ) ;
#24163=AXIS2_PLACEMENT_3D ( 'NONE', #36410, #8573, #33774 ) ;
#24164=DIRECTION ( 'NONE',  ( -0.07391278520356926729, -0.7032331762534078656, -0.7071067811865435759 ) ) ;
#24165=EDGE_CURVE ( 'NONE', #6733, #21617, #34948, .T. ) ;
#24166=EDGE_CURVE ( 'NONE', #24961, #37999, #9708, .T. ) ;
#24174=LINE ( 'NONE', #36569, #21159 ) ;
#24175=ORIENTED_EDGE ( 'NONE', *, *, #6937, .F. ) ;
#24181=CARTESIAN_POINT ( 'NONE',  ( -9.038171950369942920, 10.91067434175333872, 10.96580508970281720 ) ) ;
#24184=DIRECTION ( 'NONE',  ( 0.000000000000000000, 0.000000000000000000, 1.000000000000000000 ) ) ;
#24185=CARTESIAN_POINT ( 'NONE',  ( -2.564829916171942337, 8.028556778314829501, 10.96580508970281898 ) ) ;
#24186=ORIENTED_EDGE ( 'NONE', *, *, #30238, .T. ) ;
#24188=EDGE_CURVE ( 'NONE', #36419, #11885, #28983, .T. ) ;
#24190=ORIENTED_EDGE ( 'NONE', *, *, #17618, .T. ) ;
#24193=ORIENTED_EDGE ( 'NONE', *, *, #27520, .T. ) ;
#24196=DIRECTION ( 'NONE',  ( 1.000000000000000000, 0.000000000000000000, 0.000000000000000000 ) ) ;
#24200=ORIENTED_EDGE ( 'NONE', *, *, #7144, .F. ) ;
#24201=CARTESIAN_POINT ( 'NONE',  ( 14.31603901957230462, 19.98981538725070095, 9.500000000000000000 ) ) ;
#24202=AXIS2_PLACEMENT_3D ( 'NONE', #34415, #39903, #2936 ) ;
#24203=DIRECTION ( 'NONE',  ( 1.000000000000000000, 0.000000000000000000, 0.000000000000000000 ) ) ;
#24206=CARTESIAN_POINT ( 'NONE',  ( 5.537946624086020009, 36.44027069998191593, 7.000000000000000000 ) ) ;
#24208=ADVANCED_FACE ( 'NONE', ( #3995 ), #19851, .T. ) ;
#24209=ADVANCED_FACE ( 'NONE', ( #22478 ), #20606, .T. ) ;
#24211=CARTESIAN_POINT ( 'NONE',  ( 4.440908595777811385, 35.94977745735560859, 7.000000000000000000 ) ) ;
#24213=ORIENTED_EDGE ( 'NONE', *, *, #7121, .F. ) ;
#24214=CIRCLE ( 'NONE', #38485, 6.000000000000000000 ) ;
#24216=ORIENTED_EDGE ( 'NONE', *, *, #29670, .F. ) ;
#24221=CARTESIAN_POINT ( 'NONE',  ( -3.607749162633398843, 7.931741834401822899, 10.49999999999999822 ) ) ;
#24223=ORIENTED_EDGE ( 'NONE', *, *, #437, .F. ) ;
#24227=CARTESIAN_POINT ( 'NONE',  ( 8.118377661053324701, 10.47536095541698486, 11.00000000000000000 ) ) ;
#24230=AXIS2_PLACEMENT_3D ( 'NONE', #27411, #14828, #5673 ) ;
#24231=ORIENTED_EDGE ( 'NONE', *, *, #26393, .T. ) ;
#24234=CARTESIAN_POINT ( 'NONE',  ( -7.530592408761008549, 11.28437794979203623, 7.000000000000000000 ) ) ;
#24235=EDGE_LOOP ( 'NONE', ( #37227, #17869, #28982, #30471, #25089, #29439, #24213 ) ) ;
#24237=CARTESIAN_POINT ( 'NONE',  ( -8.412270287199731911, 10.07085245822962349, 10.49999999999999822 ) ) ;
#24238=AXIS2_PLACEMENT_3D ( 'NONE', #4469, #10767, #25593 ) ;
#24240=VERTEX_POINT ( 'NONE', #32240 ) ;
#24245=AXIS2_PLACEMENT_3D ( 'NONE', #22737, #17274, #8104 ) ;
#24247=EDGE_LOOP ( 'NONE', ( #3676, #18650, #35898, #22784 ) ) ;
#24248=EDGE_CURVE ( 'NONE', #35146, #11442, #38125, .T. ) ;
#24251=LINE ( 'NONE', #9212, #31036 ) ;
#24254=FACE_OUTER_BOUND ( 'NONE', #31559, .T. ) ;
#24257=CARTESIAN_POINT ( 'NONE',  ( 11.44473057578109199, 31.45924896672603310, 11.00000000000000000 ) ) ;
#24258=ORIENTED_EDGE ( 'NONE', *, *, #33022, .F. ) ;
#24264=DIRECTION ( 'NONE',  ( -0.5877852522924800205, -0.8090169943749424553, -0.000000000000000000 ) ) ;
#24272=LINE ( 'NONE', #5974, #4891 ) ;
#24275=CYLINDRICAL_SURFACE ( 'NONE', #17698, 0.4999999999999995559 ) ;
#24276=ORIENTED_EDGE ( 'NONE', *, *, #14626, .T. ) ;
#24278=CARTESIAN_POINT ( 'NONE',  ( -7.126083911573537044, 10.99048532364579245, 10.50000000000000000 ) ) ;
#24280=CARTESIAN_POINT ( 'NONE',  ( 9.004335565032041799, 10.95724613078621879, 10.99999999999999822 ) ) ;
#24284=LINE ( 'NONE', #3538, #7290 ) ;
#24288=PLANE ( 'NONE',  #4399 ) ;
#24289=DIRECTION ( 'NONE',  ( 1.000000000000000000, 0.000000000000000000, 0.000000000000000000 ) ) ;
#24290=LINE ( 'NONE', #30791, #33604 ) ;
#24291=ORIENTED_EDGE ( 'NONE', *, *, #1172, .T. ) ;
#24296=DIRECTION ( 'NONE',  ( 0.000000000000000000, 0.000000000000000000, 1.000000000000000000 ) ) ;
#24297=EDGE_CURVE ( 'NONE', #38258, #28430, #3794, .T. ) ;
#24300=DIRECTION ( 'NONE',  ( 1.000000000000000000, 0.000000000000000000, 0.000000000000000000 ) ) ;
#24303=ORIENTED_EDGE ( 'NONE', *, *, #16154, .F. ) ;
#24304=CARTESIAN_POINT ( 'NONE',  ( -8.007761790012255076, 9.776959832083379709, 7.000000000000000000 ) ) ;
#24305=DIRECTION ( 'NONE',  ( -1.000000000000000000, 0.000000000000000000, 0.000000000000000000 ) ) ;
#24308=DIRECTION ( 'NONE',  ( 0.2079116908177663092, 0.9781476007338041345, -0.000000000000000000 ) ) ;
#24309=DIRECTION ( 'NONE',  ( 0.8090169943749425663, -0.5877852522924797984, 0.000000000000000000 ) ) ;
#24310=DIRECTION ( 'NONE',  ( -0.000000000000000000, -0.000000000000000000, -1.000000000000000000 ) ) ;
#24311=EDGE_CURVE ( 'NONE', #36470, #7488, #23701, .T. ) ;
#24313=CARTESIAN_POINT ( 'NONE',  ( 10.44103466624280685, 32.57396620494213124, 7.000000000000000000 ) ) ;
#24314=DIRECTION ( 'NONE',  ( -0.000000000000000000, -0.000000000000000000, -1.000000000000000000 ) ) ;
#24315=ADVANCED_FACE ( 'NONE', ( #29996 ), #8257, .F. ) ;
#24316=CIRCLE ( 'NONE', #39220, 1.000000000000007772 ) ;
#24319=EDGE_LOOP ( 'NONE', ( #27124, #32219, #34638, #13664 ) ) ;
#24321=PLANE ( 'NONE',  #29137 ) ;
#24328=VECTOR ( 'NONE', #20428, 1000.000000000000227 ) ;
#24329=DIRECTION ( 'NONE',  ( -0.1470157664651938756, 0.6916548014802249567, 0.7071067811865492381 ) ) ;
#24330=CARTESIAN_POINT ( 'NONE',  ( 3.992867117591230031, 8.524771480177552263, 9.500000000000000000 ) ) ;
#24331=CIRCLE ( 'NONE', #10725, 0.5000000000000007772 ) ;
#24341=EDGE_LOOP ( 'NONE', ( #1817, #2376, #4343 ) ) ;
#24342=EDGE_CURVE ( 'NONE', #35146, #10152, #36099, .T. ) ;
#24343=CARTESIAN_POINT ( 'NONE',  ( 1.974196316410860241, 7.629928981499271679, 7.202682876670048806 ) ) ;
#24344=PLANE ( 'NONE',  #29073 ) ;
#24347=VECTOR ( 'NONE', #26625, 1000.000000000000000 ) ;
#24348=ORIENTED_EDGE ( 'NONE', *, *, #33340, .T. ) ;
#24350=ORIENTED_EDGE ( 'NONE', *, *, #19552, .F. ) ;
#24351=DIRECTION ( 'NONE',  ( -0.000000000000000000, -0.000000000000000000, -1.000000000000000000 ) ) ;
#24353=CARTESIAN_POINT ( 'NONE',  ( -1.000000000000000000, 37.50000000000000711, 7.000000000000000000 ) ) ;
#24354=AXIS2_PLACEMENT_3D ( 'NONE', #39293, #15114, #18171 ) ;
#24358=CARTESIAN_POINT ( 'NONE',  ( 8.100578861132810005, 28.44816123811117592, 10.50000000000000178 ) ) ;
#24359=DIRECTION ( 'NONE',  ( 0.6691306063588561281, -0.7431448254773961315, 0.000000000000000000 ) ) ;
#24368=DIRECTION ( 'NONE',  ( -0.4067366430757884399, 0.9135454576426061957, 0.000000000000000000 ) ) ;
#24371=B_SPLINE_CURVE_WITH_KNOTS ( 'NONE', 3,
 ( #16677, #29058, #38400, #15520, #10575, #22958 ),
 .UNSPECIFIED., .F., .F.,
 ( 4, 2, 4 ),
 ( 0.000000000000000000, 0.5000000000000000000, 1.000000000000000000 ),
 .UNSPECIFIED. ) ;
#24375=PLANE ( 'NONE',  #3009 ) ;
#24379=AXIS2_PLACEMENT_3D ( 'NONE', #19162, #22204, #13262 ) ;
#24383=VECTOR ( 'NONE', #20331, 1000.000000000000114 ) ;
#24384=DIRECTION ( 'NONE',  ( -0.000000000000000000, -0.000000000000000000, -1.000000000000000000 ) ) ;
#24385=ORIENTED_EDGE ( 'NONE', *, *, #8372, .F. ) ;
#24387=DIRECTION ( 'NONE',  ( -0.8090169943749504489, -0.5877852522924690293, 0.000000000000000000 ) ) ;
#24388=LINE ( 'NONE', #36781, #32302 ) ;
#24391=LINE ( 'NONE', #2859, #20931 ) ;
#24398=DIRECTION ( 'NONE',  ( -0.5877852522924691403, 0.8090169943749503378, 0.000000000000000000 ) ) ;
#24400=DIRECTION ( 'NONE',  ( -0.1045284632676570929, -0.9945218953682730678, 0.000000000000000000 ) ) ;
#24401=ORIENTED_EDGE ( 'NONE', *, *, #24863, .T. ) ;
#24402=DIRECTION ( 'NONE',  ( 0.000000000000000000, 0.000000000000000000, -1.000000000000000000 ) ) ;
#24404=AXIS2_PLACEMENT_3D ( 'NONE', #13825, #1440, #17298 ) ;
#24406=VECTOR ( 'NONE', #15930, 1000.000000000000000 ) ;
#24407=DIRECTION ( 'NONE',  ( 0.9781476007338036904, -0.2079116908177681133, 0.000000000000000000 ) ) ;
#24409=VECTOR ( 'NONE', #31212, 1000.000000000000114 ) ;
#24410=EDGE_CURVE ( 'NONE', #37413, #12011, #20666, .T. ) ;
#24412=FACE_OUTER_BOUND ( 'NONE', #4786, .T. ) ;
#24413=CARTESIAN_POINT ( 'NONE',  ( -9.677076426724111613, 26.69573495723220091, 11.00000000000000000 ) ) ;
#24415=ORIENTED_EDGE ( 'NONE', *, *, #6638, .T. ) ;
#24416=VERTEX_POINT ( 'NONE', #11911 ) ;
#24420=EDGE_CURVE ( 'NONE', #27849, #24787, #36167, .T. ) ;
#24422=ADVANCED_FACE ( 'NONE', ( #33064 ), #29694, .T. ) ;
#24423=VERTEX_POINT ( 'NONE', #27150 ) ;
#24428=DIRECTION ( 'NONE',  ( 1.000000000000000000, 0.000000000000000000, 0.000000000000000000 ) ) ;
#24429=ORIENTED_EDGE ( 'NONE', *, *, #5443, .F. ) ;
#24432=CARTESIAN_POINT ( 'NONE',  ( 14.06524961900339399, 27.71236540882591015, 7.500000000000000888 ) ) ;
#24435=CARTESIAN_POINT ( 'NONE',  ( -8.593266739736662885, 16.38397459621564067, 10.50000000000000000 ) ) ;
#24436=FACE_OUTER_BOUND ( 'NONE', #38775, .T. ) ;
#24437=ORIENTED_EDGE ( 'NONE', *, *, #31962, .F. ) ;
#24444=VERTEX_POINT ( 'NONE', #11712 ) ;
#24446=ADVANCED_FACE ( 'NONE', ( #12697 ), #21250, .T. ) ;
#24447=LINE ( 'NONE', #24052, #36493 ) ;
#24449=DIRECTION ( 'NONE',  ( -1.000000000000000000, 0.000000000000000000, 0.000000000000000000 ) ) ;
#24451=CARTESIAN_POINT ( 'NONE',  ( 5.767236651883443699, 13.71142893291679421, 10.00000000000000000 ) ) ;
#24452=FACE_OUTER_BOUND ( 'NONE', #27001, .T. ) ;
#24453=ORIENTED_EDGE ( 'NONE', *, *, #37444, .T. ) ;
#24455=CARTESIAN_POINT ( 'NONE',  ( 7.096882951594524869, 29.56287847632726695, 10.49999999999999467 ) ) ;
#24458=CARTESIAN_POINT ( 'NONE',  ( -12.67417846324126174, 14.47720745114824226, 7.000000000000000000 ) ) ;
#24459=EDGE_CURVE ( 'NONE', #8130, #2159, #8298, .T. ) ;
#24461=VECTOR ( 'NONE', #11308, 1000.000000000000000 ) ;
#24463=ORIENTED_EDGE ( 'NONE', *, *, #34955, .F. ) ;
#24466=DIRECTION ( 'NONE',  ( -1.000000000000000000, 0.000000000000000000, 0.000000000000000000 ) ) ;
#24473=CARTESIAN_POINT ( 'NONE',  ( -5.440908595777636414, 35.94977745735568675, 7.000000000000000000 ) ) ;
#24475=CARTESIAN_POINT ( 'NONE',  ( -0.4999999999999991673, 33.00000000000000000, 11.00000000000000000 ) ) ;
#24476=VECTOR ( 'NONE', #25104, 1000.000000000000227 ) ;
#24479=CARTESIAN_POINT ( 'NONE',  ( -14.97277451176450924, 21.48159783397892397, 10.49999999999999822 ) ) ;
#24481=ORIENTED_EDGE ( 'NONE', *, *, #30913, .T. ) ;
#24483=DIRECTION ( 'NONE',  ( 0.8090169943749504489, 0.5877852522924690293, -0.000000000000000000 ) ) ;
#24485=CARTESIAN_POINT ( 'NONE',  ( -12.30736835487442704, 14.81698729810789672, 9.000000000000001776 ) ) ;
#24489=FACE_OUTER_BOUND ( 'NONE', #33822, .T. ) ;
#24491=DIRECTION ( 'NONE',  ( -0.8090169943749505599, -0.5877852522924689183, 0.000000000000000000 ) ) ;
#24492=EDGE_CURVE ( 'NONE', #20144, #3653, #18020, .T. ) ;
#24494=VECTOR ( 'NONE', #15894, 999.9999999999997726 ) ;
#24496=ORIENTED_EDGE ( 'NONE', *, *, #29099, .T. ) ;
#24498=VECTOR ( 'NONE', #38284, 999.9999999999998863 ) ;
#24499=CIRCLE ( 'NONE', #15429, 6.000000000000001776 ) ;
#24500=DIRECTION ( 'NONE',  ( -0.1470157664651888241, 0.6916548014802291755, -0.7071067811865460184 ) ) ;
#24503=CARTESIAN_POINT ( 'NONE',  ( -5.383930013064101239, 36.46347792550319866, 10.49999999999999822 ) ) ;
#24504=CARTESIAN_POINT ( 'NONE',  ( 14.86556419889026337, 20.43481210330100595, 10.49999999999999289 ) ) ;
#24505=DIRECTION ( 'NONE',  ( 1.000000000000000000, 6.938893903907210234E-15, 0.000000000000000000 ) ) ;
#24506=CARTESIAN_POINT ( 'NONE',  ( 6.404490139165913476, 34.42612703509930583, 9.500000000000000000 ) ) ;
#24508=EDGE_CURVE ( 'NONE', #6906, #24961, #12178, .T. ) ;
#24511=CARTESIAN_POINT ( 'NONE',  ( 9.529746168869746015, 10.91601215036168959, 7.382773698552464126 ) ) ;
#24512=VERTEX_POINT ( 'NONE', #33662 ) ;
#24514=CARTESIAN_POINT ( 'NONE',  ( 14.47283171447379502, 21.48159823030310989, 9.500000000000000000 ) ) ;
#24515=CARTESIAN_POINT ( 'NONE',  ( 10.70158575030369796, 30.79011836036717753, 9.500000000000000000 ) ) ;
#24516=EDGE_CURVE ( 'NONE', #22721, #34828, #30021, .T. ) ;
#24521=VECTOR ( 'NONE', #25009, 1000.000000000000227 ) ;
#24522=ORIENTED_EDGE ( 'NONE', *, *, #7144, .T. ) ;
#24523=CARTESIAN_POINT ( 'NONE',  ( -4.000124606132347438, 8.490627681068769306, 10.49999999999999822 ) ) ;
#24534=B_SPLINE_CURVE_WITH_KNOTS ( 'NONE', 3,
 ( #2005, #20888, #11139, #20489 ),
 .UNSPECIFIED., .F., .F.,
 ( 4, 4 ),
 ( 0.000000000000000000, 0.06666641432897602026 ),
 .UNSPECIFIED. ) ;
#24536=VECTOR ( 'NONE', #23252, 1000.000000000000000 ) ;
#24537=ORIENTED_EDGE ( 'NONE', *, *, #38029, .F. ) ;
#24541=EDGE_LOOP ( 'NONE', ( #13991, #5987, #18663, #23236 ) ) ;
#24543=CARTESIAN_POINT ( 'NONE',  ( 9.331903152615748098, 11.35703883385568780, 7.000000000000000000 ) ) ;
#24544=ADVANCED_FACE ( 'NONE', ( #12502 ), #27941, .F. ) ;
#24546=EDGE_CURVE ( 'NONE', #35208, #27705, #37288, .T. ) ;
#24548=EDGE_CURVE ( 'NONE', #9704, #37413, #34442, .T. ) ;
#24549=ORIENTED_EDGE ( 'NONE', *, *, #3911, .F. ) ;
#24553=DIRECTION ( 'NONE',  ( 1.000000000000000000, 0.000000000000000000, 0.000000000000000000 ) ) ;
#24554=VECTOR ( 'NONE', #37975, 1000.000000000000000 ) ;
#24555=AXIS2_PLACEMENT_3D ( 'NONE', #12045, #3100, #19942 ) ;
#24556=LINE ( 'NONE', #27996, #32429 ) ;
#24557=ORIENTED_EDGE ( 'NONE', *, *, #3090, .F. ) ;
#24560=DIRECTION ( 'NONE',  ( -1.000000000000000000, 0.000000000000000000, 0.000000000000000000 ) ) ;
#24562=DIRECTION ( 'NONE',  ( 0.000000000000000000, 0.000000000000000000, -1.000000000000000000 ) ) ;
#24567=VERTEX_POINT ( 'NONE', #31389 ) ;
#24572=DIRECTION ( 'NONE',  ( -1.000000000000000000, 0.000000000000000000, 0.000000000000000000 ) ) ;
#24577=CARTESIAN_POINT ( 'NONE',  ( 11.48173768534035943, 32.16538668264416145, 10.49999999999999822 ) ) ;
#24579=ORIENTED_EDGE ( 'NONE', *, *, #14965, .F. ) ;
#24581=CARTESIAN_POINT ( 'NONE',  ( 0.9938779058054629800, 37.09261900150649893, 10.49999999999999822 ) ) ;
#24583=AXIS2_PLACEMENT_3D ( 'NONE', #38432, #19951, #4507 ) ;
#24584=AXIS2_PLACEMENT_3D ( 'NONE', #36904, #30615, #33671 ) ;
#24585=CARTESIAN_POINT ( 'NONE',  ( -9.359089477944888102, 11.31962006718894109, 10.49999999999999822 ) ) ;
#24586=EDGE_LOOP ( 'NONE', ( #9155, #5885, #28288 ) ) ;
#24591=B_SPLINE_SURFACE_WITH_KNOTS ( 'NONE', 1, 3, ( 
 ( #4363, #32616, #1323, #35657, #16161, #28547, #721, #28945, #4160, #13505 ),
 ( #25893, #38292, #25488, #34848, #10463, #35249, #7406, #26095, #38493, #8825 ) ),
 .UNSPECIFIED., .F., .F., .F.,
 ( 2, 2 ),
 ( 4, 2, 2, 2, 4 ),
 ( 0.000000000000000000, 1.000000000000000000 ),
 ( 1.875797233020303878, 2.268496314719027129, 2.661195396417750381, 3.053894478116473632, 3.446593559815196883 ),
 .UNSPECIFIED. ) ;
#24592=ORIENTED_EDGE ( 'NONE', *, *, #14579, .T. ) ;
#24597=ORIENTED_EDGE ( 'NONE', *, *, #6164, .F. ) ;
#24601=CYLINDRICAL_SURFACE ( 'NONE', #3972, 0.5000000000000006661 ) ;
#24605=LINE ( 'NONE', #31301, #26139 ) ;
#24608=DIRECTION ( 'NONE',  ( 1.000000000000000000, 0.000000000000000000, 0.000000000000000000 ) ) ;
#24610=VECTOR ( 'NONE', #12128, 1000.000000000000000 ) ;
#24613=CARTESIAN_POINT ( 'NONE',  ( 7.713869163865849643, 10.18146832927074996, 10.49999999999999822 ) ) ;
#24614=AXIS2_PLACEMENT_3D ( 'NONE', #6304, #12804, #3661 ) ;
#24615=LINE ( 'NONE', #24211, #34573 ) ;
#24616=CARTESIAN_POINT ( 'NONE',  ( 2.544902299099474519, 8.122308845603164684, 10.99387789255784398 ) ) ;
#24617=ORIENTED_EDGE ( 'NONE', *, *, #19505, .F. ) ;
#24622=ORIENTED_EDGE ( 'NONE', *, *, #18293, .F. ) ;
#24623=ORIENTED_EDGE ( 'NONE', *, *, #7160, .F. ) ;
#24633=CARTESIAN_POINT ( 'NONE',  ( 6.811226782241714517, 35.33967249274190436, 9.500000000000000000 ) ) ;
#24634=CARTESIAN_POINT ( 'NONE',  ( 13.05736835487433289, 16.11602540378438420, 7.000000000000000000 ) ) ;
#24637=ORIENTED_EDGE ( 'NONE', *, *, #9384, .T. ) ;
#24645=CIRCLE ( 'NONE', #22053, 15.00000000000000000 ) ;
#24646=CARTESIAN_POINT ( 'NONE',  ( -10.16122020288868733, 33.53402030034415304, 7.000000000000000000 ) ) ;
#24650=DIRECTION ( 'NONE',  ( 0.8660254037844364872, -0.5000000000000038858, 0.000000000000000000 ) ) ;
#24654=VERTEX_POINT ( 'NONE', #31192 ) ;
#24657=LINE ( 'NONE', #24855, #13612 ) ;
#24661=ORIENTED_EDGE ( 'NONE', *, *, #29498, .F. ) ;
#24664=ADVANCED_FACE ( 'NONE', ( #12306 ), #3357, .T. ) ;
#24665=EDGE_CURVE ( 'NONE', #34232, #16528, #316, .T. ) ;
#24670=AXIS2_PLACEMENT_3D ( 'NONE', #13957, #39342, #17222 ) ;
#24671=EDGE_LOOP ( 'NONE', ( #26269, #17300, #9343, #20831, #30893, #7091, #38119 ) ) ;
#24673=FACE_OUTER_BOUND ( 'NONE', #17401, .T. ) ;
#24675=LINE ( 'NONE', #30781, #14616 ) ;
#24678=CARTESIAN_POINT ( 'NONE',  ( -14.76265446396242176, 21.90695576875699757, 10.49999999999999467 ) ) ;
#24680=EDGE_LOOP ( 'NONE', ( #15925, #20650, #39194, #38062 ) ) ;
#24682=CARTESIAN_POINT ( 'NONE',  ( -11.11016527260153630, 31.83082137946488643, 7.500000000000004441 ) ) ;
#24684=DIRECTION ( 'NONE',  ( 0.000000000000000000, 0.000000000000000000, 1.000000000000000000 ) ) ;
#24685=VERTEX_POINT ( 'NONE', #18610 ) ;
#24688=VECTOR ( 'NONE', #3708, 999.9999999999998863 ) ;
#24689=CARTESIAN_POINT ( 'NONE',  ( -5.644276917315528941, 36.40655018617697891, 10.49999999999999467 ) ) ;
#24691=AXIS2_PLACEMENT_3D ( 'NONE', #11920, #35906, #30418 ) ;
#24693=EDGE_CURVE ( 'NONE', #9581, #29091, #19194, .T. ) ;
#24695=CARTESIAN_POINT ( 'NONE',  ( -13.94482798346716201, 26.50521816028930644, 7.000000000000000000 ) ) ;
#24697=VECTOR ( 'NONE', #7510, 999.9999999999998863 ) ;
#24698=CARTESIAN_POINT ( 'NONE',  ( 2.525645716490524606, 8.212903943950921715, 11.00000000000000000 ) ) ;
#24700=LINE ( 'NONE', #25098, #22907 ) ;
#24702=CARTESIAN_POINT ( 'NONE',  ( 0.000000000000000000, 22.50000000000000355, 7.000000000000000000 ) ) ;
#24703=DIRECTION ( 'NONE',  ( 0.000000000000000000, 0.000000000000000000, -1.000000000000000000 ) ) ;
#24705=DIRECTION ( 'NONE',  ( 1.000000000000000000, 0.000000000000000000, 0.000000000000000000 ) ) ;
#24706=CARTESIAN_POINT ( 'NONE',  ( 11.89076109989491314, 31.64473967131989340, 7.202682876670051471 ) ) ;
#24709=DIRECTION ( 'NONE',  ( 1.000000000000000000, 0.000000000000000000, 0.000000000000000000 ) ) ;
#24710=ORIENTED_EDGE ( 'NONE', *, *, #18685, .T. ) ;
#24712=DIRECTION ( 'NONE',  ( -0.04273212933194531216, -0.8153776007405577619, 0.5773502691896226224 ) ) ;
#24719=ORIENTED_EDGE ( 'NONE', *, *, #2018, .F. ) ;
#24720=DIRECTION ( 'NONE',  ( -0.000000000000000000, -0.000000000000000000, -1.000000000000000000 ) ) ;
#24727=PLANE ( 'NONE',  #4358 ) ;
#24728=AXIS2_PLACEMENT_3D ( 'NONE', #9325, #34699, #18667 ) ;
#24730=ORIENTED_EDGE ( 'NONE', *, *, #34199, .F. ) ;
#24733=EDGE_LOOP ( 'NONE', ( #39426, #9501, #34294, #29723 ) ) ;
#24734=FACE_OUTER_BOUND ( 'NONE', #36243, .T. ) ;
#24735=DIRECTION ( 'NONE',  ( -0.9510565162951541973, -0.3090169943749456194, 0.000000000000000000 ) ) ;
#24737=EDGE_CURVE ( 'NONE', #2507, #32523, #29344, .T. ) ;
#24739=EDGE_CURVE ( 'NONE', #3978, #36251, #13697, .T. ) ;
#24740=AXIS2_PLACEMENT_3D ( 'NONE', #17120, #26647, #1671 ) ;
#24741=ORIENTED_EDGE ( 'NONE', *, *, #6160, .T. ) ;
#24742=FACE_OUTER_BOUND ( 'NONE', #8216, .T. ) ;
#24743=VERTEX_POINT ( 'NONE', #20007 ) ;
#24744=CARTESIAN_POINT ( 'NONE',  ( -7.126083911573537044, 10.99048532364579245, 9.500000000000000000 ) ) ;
#24745=CARTESIAN_POINT ( 'NONE',  ( 4.591666147298500533, 15.32946292166668556, 7.000000000000000000 ) ) ;
#24746=EDGE_CURVE ( 'NONE', #11507, #31582, #38127, .T. ) ;
#24748=VERTEX_POINT ( 'NONE', #7194 ) ;
#24750=DIRECTION ( 'NONE',  ( -1.000000000000000000, -1.224646799147353947E-16, 0.000000000000000000 ) ) ;
#24751=DIRECTION ( 'NONE',  ( -0.5877852522924796874, -0.8090169943749426773, 0.000000000000000000 ) ) ;
#24752=AXIS2_PLACEMENT_3D ( 'NONE', #2059, #36182, #33142 ) ;
#24753=CARTESIAN_POINT ( 'NONE',  ( -7.713869163866016621, 10.18146832927085121, 10.50000000000000711 ) ) ;
#24759=CARTESIAN_POINT ( 'NONE',  ( -14.84160187385925589, 20.32586711127000711, 7.500000000000004441 ) ) ;
#24761=B_SPLINE_CURVE_WITH_KNOTS ( 'NONE', 3,
 ( #2696, #33192, #39860, #21381, #10188, #28272 ),
 .UNSPECIFIED., .F., .F.,
 ( 4, 2, 4 ),
 ( 0.000000000000000000, 0.5000000000000000000, 1.000000000000000000 ),
 .UNSPECIFIED. ) ;
#24763=EDGE_CURVE ( 'NONE', #34172, #15434, #16964, .T. ) ;
#24764=EDGE_CURVE ( 'NONE', #5911, #32217, #5677, .T. ) ;
#24766=CARTESIAN_POINT ( 'NONE',  ( -10.81260707898136708, 32.90853150812170469, 10.49999999999999822 ) ) ;
#24767=ADVANCED_FACE ( 'NONE', ( #22432 ), #22232, .T. ) ;
#24769=CONICAL_SURFACE ( 'NONE', #7241, 1.000000000000000888, 0.7853981633974552734 ) ;
#24772=FACE_OUTER_BOUND ( 'NONE', #14807, .T. ) ;
#24773=EDGE_LOOP ( 'NONE', ( #11807, #18009, #4528, #24792 ) ) ;
#24775=CARTESIAN_POINT ( 'NONE',  ( 0.5000000000000000000, 37.39061994947686429, 10.82238861112342043 ) ) ;
#24776=CARTESIAN_POINT ( 'NONE',  ( -14.36830325120615548, 20.48707633493503621, 7.000000000000000000 ) ) ;
#24777=CARTESIAN_POINT ( 'NONE',  ( -9.156995300982224251, 10.74712803024086938, 10.82238861112329609 ) ) ;
#24778=ORIENTED_EDGE ( 'NONE', *, *, #23651, .T. ) ;
#24781=VECTOR ( 'NONE', #1458, 1000.000000000000000 ) ;
#24783=ORIENTED_EDGE ( 'NONE', *, *, #38159, .F. ) ;
#24785=LINE ( 'NONE', #9558, #34555 ) ;
#24786=ADVANCED_FACE ( 'NONE', ( #26085 ), #13290, .T. ) ;
#24787=VERTEX_POINT ( 'NONE', #19801 ) ;
#24792=ORIENTED_EDGE ( 'NONE', *, *, #2842, .F. ) ;
#24795=CARTESIAN_POINT ( 'NONE',  ( -1.400691654708310585, 37.43445890845833901, 7.000000000000000000 ) ) ;
#24797=EDGE_CURVE ( 'NONE', #18928, #34264, #34887, .T. ) ;
#24799=EDGE_LOOP ( 'NONE', ( #20176, #29312, #23966, #30145, #38883, #675, #5747 ) ) ;
#24800=CONICAL_SURFACE ( 'NONE', #30671, 1.000000000000013101, 0.7853981633974566057 ) ;
#24801=CARTESIAN_POINT ( 'NONE',  ( 3.938766756526715263, 8.166638875703695177, 10.49999999999999822 ) ) ;
#24802=CARTESIAN_POINT ( 'NONE',  ( 10.20374679324142342, 33.03312760923203939, 10.49999999999999645 ) ) ;
#24803=DIRECTION ( 'NONE',  ( 0.3090169943749465631, -0.9510565162951538642, 0.000000000000000000 ) ) ;
#24806=CYLINDRICAL_SURFACE ( 'NONE', #16614, 0.4999999999999995559 ) ;
#24807=AXIS2_PLACEMENT_3D ( 'NONE', #33239, #23675, #11884 ) ;
#24809=CARTESIAN_POINT ( 'NONE',  ( -9.776449189803978257, 11.12328344838602767, 7.150945465624456432 ) ) ;
#24810=LINE ( 'NONE', #30317, #6037 ) ;
#24812=ADVANCED_FACE ( 'NONE', ( #4150 ), #25685, .T. ) ;
#24815=CONICAL_SURFACE ( 'NONE', #22838, 1.000000000000004441, 0.7853981633974528309 ) ;
#24819=ORIENTED_EDGE ( 'NONE', *, *, #34244, .F. ) ;
#24824=ORIENTED_EDGE ( 'NONE', *, *, #14701, .F. ) ;
#24826=PRODUCT_DEFINITION_CONTEXT ( 'detailed design', #14524, 'design' ) ;
#24828=CONICAL_SURFACE ( 'NONE', #7303, 0.4999999999999955036, 0.7853981633974447263 ) ;
#24829=DIRECTION ( 'NONE',  ( 1.000000000000000000, 0.000000000000000000, 0.000000000000000000 ) ) ;
#24830=ORIENTED_EDGE ( 'NONE', *, *, #21507, .F. ) ;
#24832=CARTESIAN_POINT ( 'NONE',  ( -11.48173768534023154, 32.16538668264431777, 7.000000000000000000 ) ) ;
#24834=EDGE_LOOP ( 'NONE', ( #30054, #17708, #17049, #20685 ) ) ;
#24836=ORIENTED_EDGE ( 'NONE', *, *, #19189, .T. ) ;
#24838=AXIS2_PLACEMENT_3D ( 'NONE', #26510, #17385, #8623 ) ;
#24841=ADVANCED_FACE ( 'NONE', ( #37686 ), #35446, .F. ) ;
#24842=ORIENTED_EDGE ( 'NONE', *, *, #39274, .F. ) ;
#24844=DIRECTION ( 'NONE',  ( -0.5000000000000041078, -0.8660254037844362651, 0.000000000000000000 ) ) ;
#24846=AXIS2_PLACEMENT_3D ( 'NONE', #17761, #36242, #39271 ) ;
#24848=CARTESIAN_POINT ( 'NONE',  ( -0.5000000000000005551, 32.50000000000000000, 10.49999999999999645 ) ) ;
#24849=AXIS2_PLACEMENT_3D ( 'NONE', #17639, #17231, #5620 ) ;
#24851=VECTOR ( 'NONE', #5220, 1000.000000000000000 ) ;
#24855=CARTESIAN_POINT ( 'NONE',  ( 8.238488885696289898, 24.65111619403943877, 7.000000000000000000 ) ) ;
#24863=EDGE_CURVE ( 'NONE', #27538, #18534, #15481, .T. ) ;
#24874=ORIENTED_EDGE ( 'NONE', *, *, #27020, .T. ) ;
#24877=DIRECTION ( 'NONE',  ( 1.000000000000000000, 0.000000000000000000, 0.000000000000000000 ) ) ;
#24879=EDGE_LOOP ( 'NONE', ( #33106, #33270, #24231, #16205 ) ) ;
#24882=CARTESIAN_POINT ( 'NONE',  ( -5.440908595777636414, 35.94977745735568675, 11.00000000000000000 ) ) ;
#24884=CARTESIAN_POINT ( 'NONE',  ( -3.813962023474485985, 32.29559562678527129, 10.00000000000000000 ) ) ;
#24885=EDGE_LOOP ( 'NONE', ( #21980, #39410, #23129, #3135 ) ) ;
#24888=FACE_OUTER_BOUND ( 'NONE', #4147, .T. ) ;
#24892=B_SPLINE_CURVE_WITH_KNOTS ( 'NONE', 3,
 ( #3265, #224, #36996, #33949 ),
 .UNSPECIFIED., .F., .F.,
 ( 4, 4 ),
 ( 0.000000000000000000, 1.000000000000000000 ),
 .UNSPECIFIED. ) ;
#24895=CARTESIAN_POINT ( 'NONE',  ( -10.44103466624267185, 32.57396620494226624, 11.00000000000000000 ) ) ;
#24896=ORIENTED_EDGE ( 'NONE', *, *, #32515, .T. ) ;
#24897=EDGE_CURVE ( 'NONE', #39323, #38584, #21255, .T. ) ;
#24898=LINE ( 'NONE', #40134, #36596 ) ;
#24903=LINE ( 'NONE', #37694, #28897 ) ;
#24904=LINE ( 'NONE', #34646, #16923 ) ;
#24905=CARTESIAN_POINT ( 'NONE',  ( 2.806807826039672715, 9.295007390093600108, 7.000000000000000000 ) ) ;
#24906=DIRECTION ( 'NONE',  ( 0.9781476007338069101, 0.2079116908177532641, 0.000000000000000000 ) ) ;
#24907=CARTESIAN_POINT ( 'NONE',  ( -1.204925152852743375, 12.02153850147729486, 10.50000000000000000 ) ) ;
#24910=CARTESIAN_POINT ( 'NONE',  ( -10.14060191828654212, 25.26915018278947755, 10.50000000000000000 ) ) ;
#24914=CIRCLE ( 'NONE', #932, 0.5000000000000000000 ) ;
#24915=CARTESIAN_POINT ( 'NONE',  ( 13.24038105676655341, 15.43301270189216190, 10.49999999999999822 ) ) ;
#24921=B_SPLINE_SURFACE_WITH_KNOTS ( 'NONE', 1, 3, ( 
 ( #1446, #19526, #4084, #26223, #1048, #16896, #19937, #32124, #4290, #23178 ),
 ( #35576, #36379, #14641, #11597, #17705, #23983, #8346, #39415, #27033, #8543 ) ),
 .UNSPECIFIED., .F., .F., .F.,
 ( 2, 2 ),
 ( 4, 2, 2, 2, 4 ),
 ( 0.000000000000000000, 1.000000000000000000 ),
 ( -1.183199640139722675, -0.7905005584409985353, -0.3978014767422745068, -0.005102395043550450593, 0.3875966866551736056 ),
 .UNSPECIFIED. ) ;
#24922=ORIENTED_EDGE ( 'NONE', *, *, #16084, .T. ) ;
#24923=DIRECTION ( 'NONE',  ( -0.8090169943749426773, 0.5877852522924796874, 0.000000000000000000 ) ) ;
#24932=CARTESIAN_POINT ( 'NONE',  ( 8.633502029282041690, 11.46765470489692795, 9.500000000000000000 ) ) ;
#24933=EDGE_CURVE ( 'NONE', #35208, #30083, #14102, .T. ) ;
#24934=ORIENTED_EDGE ( 'NONE', *, *, #33963, .T. ) ;
#24938=CARTESIAN_POINT ( 'NONE',  ( 5.440908595777814050, 35.94977745735560859, 7.500000000000000888 ) ) ;
#24939=CARTESIAN_POINT ( 'NONE',  ( -11.94134295108997890, 16.18301270189233421, 7.000000000000000000 ) ) ;
#24943=ORIENTED_EDGE ( 'NONE', *, *, #5045, .T. ) ;
#24944=ADVANCED_FACE ( 'NONE', ( #11265 ), #4967, .T. ) ;
#24947=EDGE_CURVE ( 'NONE', #26077, #10398, #38893, .T. ) ;
#24949=DIRECTION ( 'NONE',  ( 0.000000000000000000, 0.000000000000000000, 1.000000000000000000 ) ) ;
#24951=DIRECTION ( 'NONE',  ( 0.000000000000000000, 0.000000000000000000, 1.000000000000000000 ) ) ;
#24955=DIRECTION ( 'NONE',  ( -0.7071067811865546782, 0.000000000000000000, -0.7071067811865403563 ) ) ;
#24957=CARTESIAN_POINT ( 'NONE',  ( 6.557822374958316658, 35.99981354310111215, 11.00000000000000000 ) ) ;
#24958=PLANE ( 'NONE',  #20989 ) ;
#24960=VECTOR ( 'NONE', #11219, 1000.000000000000000 ) ;
#24961=VERTEX_POINT ( 'NONE', #23851 ) ;
#24965=DIRECTION ( 'NONE',  ( -0.000000000000000000, -0.000000000000000000, -1.000000000000000000 ) ) ;
#24968=EDGE_CURVE ( 'NONE', #37600, #31884, #26636, .T. ) ;
#24969=CARTESIAN_POINT ( 'NONE',  ( 11.07315816304239320, 31.12468366354660532, 10.50000000000000000 ) ) ;
#24976=VERTEX_POINT ( 'NONE', #20813 ) ;
#24979=DIRECTION ( 'NONE',  ( 0.000000000000000000, 0.000000000000000000, 1.000000000000000000 ) ) ;
#24980=AXIS2_PLACEMENT_3D ( 'NONE', #28468, #643, #22566 ) ;
#24981=PLANE ( 'NONE',  #39024 ) ;
#24985=CARTESIAN_POINT ( 'NONE',  ( -5.644276917315533382, 36.40655018617698602, 7.000000000000000000 ) ) ;
#24986=ORIENTED_EDGE ( 'NONE', *, *, #10015, .F. ) ;
#24987=VECTOR ( 'NONE', #20834, 1000.000000000000000 ) ;
#24989=CARTESIAN_POINT ( 'NONE',  ( -9.331903152615899089, 11.35703883385581037, 10.50000000000000533 ) ) ;
#24990=ORIENTED_EDGE ( 'NONE', *, *, #26697, .T. ) ;
#24992=AXIS2_PLACEMENT_3D ( 'NONE', #23960, #2428, #5467 ) ;
#24996=DIRECTION ( 'NONE',  ( -0.6691306063588671194, -0.7431448254773862505, 0.000000000000000000 ) ) ;
#24997=CARTESIAN_POINT ( 'NONE',  ( -1.160189012974344180, 37.45561938550757475, 7.203056206335832101 ) ) ;
#25002=CARTESIAN_POINT ( 'NONE',  ( 3.503793317224327630, 8.420815634768672453, 11.00000000000000355 ) ) ;
#25004=DIRECTION ( 'NONE',  ( 0.000000000000000000, 0.000000000000000000, 1.000000000000000000 ) ) ;
#25009=DIRECTION ( 'NONE',  ( 0.1045284632676436176, -0.9945218953682742891, 0.000000000000000000 ) ) ;
#25010=EDGE_CURVE ( 'NONE', #21446, #23552, #39489, .T. ) ;
#25011=EDGE_LOOP ( 'NONE', ( #10098, #2831, #27142, #15319 ) ) ;
#25012=VECTOR ( 'NONE', #16159, 1000.000000000000114 ) ;
#25014=AXIS2_PLACEMENT_3D ( 'NONE', #22973, #29677, #35376 ) ;
#25019=ORIENTED_EDGE ( 'NONE', *, *, #36090, .T. ) ;
#25020=ORIENTED_EDGE ( 'NONE', *, *, #36452, .T. ) ;
#25024=ORIENTED_EDGE ( 'NONE', *, *, #12633, .F. ) ;
#25025=EDGE_CURVE ( 'NONE', #13640, #15240, #38156, .T. ) ;
#25028=CARTESIAN_POINT ( 'NONE',  ( 0.5000000000000000000, 37.44611345180490503, 10.76099332938163755 ) ) ;
#25029=ORIENTED_EDGE ( 'NONE', *, *, #13699, .T. ) ;
#25031=DIRECTION ( 'NONE',  ( 1.000000000000000000, 0.000000000000000000, 0.000000000000000000 ) ) ;
#25033=ORIENTED_EDGE ( 'NONE', *, *, #33755, .F. ) ;
#25035=ORIENTED_EDGE ( 'NONE', *, *, #290, .T. ) ;
#25039=ORIENTED_EDGE ( 'NONE', *, *, #21909, .T. ) ;
#25041=VECTOR ( 'NONE', #35165, 1000.000000000000114 ) ;
#25042=EDGE_CURVE ( 'NONE', #14313, #6492, #30152, .T. ) ;
#25044=ADVANCED_FACE ( 'NONE', ( #26699 ), #8964, .T. ) ;
#25046=AXIS2_PLACEMENT_3D ( 'NONE', #4828, #33079, #5229 ) ;
#25047=VECTOR ( 'NONE', #30437, 1000.000000000000114 ) ;
#25049=VECTOR ( 'NONE', #24164, 1000.000000000000114 ) ;
#25050=CYLINDRICAL_SURFACE ( 'NONE', #11731, 0.5000000000000000000 ) ;
#25052=CARTESIAN_POINT ( 'NONE',  ( -16.72075857324140102, 7.444561356925720297, 7.000000000000000000 ) ) ;
#25054=CARTESIAN_POINT ( 'NONE',  ( 0.5000000000000002220, 36.50000000000000711, 10.00000000000000000 ) ) ;
#25055=DIRECTION ( 'NONE',  ( 0.6691306063588670083, 0.7431448254773863615, 0.000000000000000000 ) ) ;
#25063=EDGE_CURVE ( 'NONE', #38335, #37600, #3125, .T. ) ;
#25064=CARTESIAN_POINT ( 'NONE',  ( -2.036571916123810055, 8.108948098542073879, 7.000000000000000000 ) ) ;
#25066=ORIENTED_EDGE ( 'NONE', *, *, #18470, .F. ) ;
#25068=ORIENTED_EDGE ( 'NONE', *, *, #39297, .F. ) ;
#25070=CARTESIAN_POINT ( 'NONE',  ( 1.932616070714738177, 8.598021898908950078, 10.50000000000000000 ) ) ;
#25073=CIRCLE ( 'NONE', #1068, 0.5000000000000004441 ) ;
#25074=ORIENTED_EDGE ( 'NONE', *, *, #4112, .T. ) ;
#25077=CYLINDRICAL_SURFACE ( 'NONE', #15706, 0.5000000000000004441 ) ;
#25079=ORIENTED_EDGE ( 'NONE', *, *, #30691, .F. ) ;
#25081=VECTOR ( 'NONE', #33976, 1000.000000000000114 ) ;
#25083=CARTESIAN_POINT ( 'NONE',  ( -13.30736835491669368, 15.59574623945408511, 10.49999999999999822 ) ) ;
#25085=ORIENTED_EDGE ( 'NONE', *, *, #31935, .T. ) ;
#25089=ORIENTED_EDGE ( 'NONE', *, *, #30545, .F. ) ;
#25093=EDGE_CURVE ( 'NONE', #28064, #11050, #19983, .T. ) ;
#25094=DIRECTION ( 'NONE',  ( 0.07391278520356926729, 0.7032331762534078656, -0.7071067811865435759 ) ) ;
#25096=CIRCLE ( 'NONE', #30305, 0.5000000000000004441 ) ;
#25097=DIRECTION ( 'NONE',  ( 1.000000000000000000, 0.000000000000000000, 0.000000000000000000 ) ) ;
#25098=CARTESIAN_POINT ( 'NONE',  ( -2.140527761532693418, 7.619874298175171035, 7.000000000000000000 ) ) ;
#25100=FACE_OUTER_BOUND ( 'NONE', #33766, .T. ) ;
#25103=B_SPLINE_CURVE_WITH_KNOTS ( 'NONE', 3,
 ( #22371, #13432, #31727, #25826, #22574, #1256 ),
 .UNSPECIFIED., .F., .F.,
 ( 4, 2, 4 ),
 ( 0.000000000000000000, 0.5000000000000000000, 1.000000000000000000 ),
 .UNSPECIFIED. ) ;
#25104=DIRECTION ( 'NONE',  ( -0.8910065241883629028, 0.4539904997395564079, 3.261825160244155287E-15 ) ) ;
#25105=DIRECTION ( 'NONE',  ( -1.000000000000000000, 0.000000000000000000, 0.000000000000000000 ) ) ;
#25106=LINE ( 'NONE', #12910, #20358 ) ;
#25109=DIRECTION ( 'NONE',  ( -1.000000000000000000, 0.000000000000000000, 0.000000000000000000 ) ) ;
#25110=EDGE_LOOP ( 'NONE', ( #23776, #2489, #38132, #2249, #31527, #31135 ) ) ;
#25112=CARTESIAN_POINT ( 'NONE',  ( -8.410254037844435260, 17.06698729810786475, 10.50000000000000000 ) ) ;
#25119=FACE_OUTER_BOUND ( 'NONE', #10586, .T. ) ;
#25126=DIRECTION ( 'NONE',  ( 0.5000000000000039968, 0.8660254037844363761, 0.000000000000000000 ) ) ;
#25127=EDGE_CURVE ( 'NONE', #13873, #5508, #24251, .T. ) ;
#25130=VECTOR ( 'NONE', #6142, 1000.000000000000000 ) ;
#25131=TOROIDAL_SURFACE ( 'NONE', #5669, 1.000000000000000000, 0.5000000000000000000 ) ;
#25136=AXIS2_PLACEMENT_3D ( 'NONE', #19593, #31985, #16351 ) ;
#25140=CIRCLE ( 'NONE', #29054, 0.5000000000000004441 ) ;
#25142=VERTEX_POINT ( 'NONE', #30557 ) ;
#25143=ORIENTED_EDGE ( 'NONE', *, *, #9740, .T. ) ;
#25144=CARTESIAN_POINT ( 'NONE',  ( -9.343266739736645121, 17.68301270189229868, 11.00000000000000000 ) ) ;
#25145=CARTESIAN_POINT ( 'NONE',  ( -14.97283171447380390, 21.48159823030330884, 7.000000000000000000 ) ) ;
#25146=LINE ( 'NONE', #18464, #17529 ) ;
#25148=EDGE_CURVE ( 'NONE', #25142, #6401, #4560, .T. ) ;
#25150=CARTESIAN_POINT ( 'NONE',  ( -5.982165713378355676, 28.55918256678905820, 7.000000000000000000 ) ) ;
#25152=ADVANCED_FACE ( 'NONE', ( #5956 ), #21792, .T. ) ;
#25153=CIRCLE ( 'NONE', #3840, 0.4999999999999998890 ) ;
#25154=DIRECTION ( 'NONE',  ( 0.6916548014802255118, 0.1470157664652010365, -0.7071067811865469066 ) ) ;
#25156=DIRECTION ( 'NONE',  ( 1.000000000000000000, 0.000000000000000000, 0.000000000000000000 ) ) ;
#25159=AXIS2_PLACEMENT_3D ( 'NONE', #12686, #37276, #22031 ) ;
#25164=DIRECTION ( 'NONE',  ( 1.000000000000000000, 0.000000000000000000, 0.000000000000000000 ) ) ;
#25168=CARTESIAN_POINT ( 'NONE',  ( -5.068835528549854530, 13.82204480395809476, 10.50000000000000533 ) ) ;
#25169=VECTOR ( 'NONE', #20943, 999.9999999999998863 ) ;
#25174=EDGE_CURVE ( 'NONE', #13016, #10646, #5074, .T. ) ;
#25175=FACE_OUTER_BOUND ( 'NONE', #27394, .T. ) ;
#25176=LINE ( 'NONE', #37368, #17031 ) ;
#25178=VERTEX_POINT ( 'NONE', #34000 ) ;
#25180=DIRECTION ( 'NONE',  ( 0.9945218953682742891, 0.1045284632676437425, 0.000000000000000000 ) ) ;
#25181=CARTESIAN_POINT ( 'NONE',  ( -13.63396663385394803, 16.24580510161721847, 7.000000000000000000 ) ) ;
#25182=DIRECTION ( 'NONE',  ( 0.7431448254773862505, -0.6691306063588670083, -0.000000000000000000 ) ) ;
#25186=DIRECTION ( 'NONE',  ( -0.3090169943749573322, -0.9510565162951504226, 0.000000000000000000 ) ) ;
#25187=ORIENTED_EDGE ( 'NONE', *, *, #12593, .F. ) ;
#25192=AXIS2_PLACEMENT_3D ( 'NONE', #21396, #10916, #38936 ) ;
#25193=ORIENTED_EDGE ( 'NONE', *, *, #10162, .F. ) ;
#25195=AXIS2_PLACEMENT_3D ( 'NONE', #2813, #18263, #9715 ) ;
#25197=FACE_OUTER_BOUND ( 'NONE', #16531, .T. ) ;
#25198=ADVANCED_FACE ( 'NONE', ( #18360 ), #32310, .T. ) ;
#25201=DIRECTION ( 'NONE',  ( -0.000000000000000000, -0.000000000000000000, -1.000000000000000000 ) ) ;
#25202=ORIENTED_EDGE ( 'NONE', *, *, #6067, .T. ) ;
#25203=CARTESIAN_POINT ( 'NONE',  ( -3.914034194965524183, 30.06176806842423943, 9.000000000000001776 ) ) ;
#25211=CARTESIAN_POINT ( 'NONE',  ( 9.363324537585983265, 32.27640801132196913, 9.500000000000000000 ) ) ;
#25212=AXIS2_PLACEMENT_3D ( 'NONE', #16839, #1192, #32683 ) ;
#25215=VECTOR ( 'NONE', #20882, 999.9999999999998863 ) ;
#25218=CYLINDRICAL_SURFACE ( 'NONE', #23742, 0.5000000000000007772 ) ;
#25220=ORIENTED_EDGE ( 'NONE', *, *, #33755, .T. ) ;
#25221=ORIENTED_EDGE ( 'NONE', *, *, #1200, .F. ) ;
#25222=CIRCLE ( 'NONE', #28466, 6.000000000000003553 ) ;
#25229=ORIENTED_EDGE ( 'NONE', *, *, #27179, .F. ) ;
#25231=CARTESIAN_POINT ( 'NONE',  ( 13.49038105676655164, 15.86602540378438064, 7.000000000000000000 ) ) ;
#25232=CARTESIAN_POINT ( 'NONE',  ( 2.525645716490518389, 8.212903943950921715, 7.499999999999990230 ) ) ;
#25237=CARTESIAN_POINT ( 'NONE',  ( -11.48173768534023154, 32.16538668264431777, 10.49999999999999822 ) ) ;
#25239=ORIENTED_EDGE ( 'NONE', *, *, #17590, .F. ) ;
#25240=CARTESIAN_POINT ( 'NONE',  ( 4.591666147298500533, 15.32946292166668556, 9.000000000000001776 ) ) ;
#25241=EDGE_CURVE ( 'NONE', #10259, #24976, #18558, .T. ) ;
#25243=VECTOR ( 'NONE', #29511, 1000.000000000000227 ) ;
#25245=DIRECTION ( 'NONE',  ( 0.1045284632676564129, 0.9945218953682731788, 0.000000000000000000 ) ) ;
#25248=PLANE ( 'NONE',  #5231 ) ;
#25249=B_SPLINE_SURFACE_WITH_KNOTS ( 'NONE', 1, 3, ( 
 ( #16032, #31671, #18146, #19272, #33785, #30330, #10137, #6478, #27279, #37570 ),
 ( #33586, #18883, #15834, #27471, #3437, #5739, #31471, #14890, #34523, #24227 ) ),
 .UNSPECIFIED., .F., .F., .F.,
 ( 2, 2 ),
 ( 4, 2, 2, 2, 4 ),
 ( 0.000000000000000000, 1.000000000000000000 ),
 ( 4.237807397716039759, 4.630506479414762566, 5.023205561113485373, 5.415904642812208181, 5.808603724510930100 ),
 .UNSPECIFIED. ) ;
#25255=CARTESIAN_POINT ( 'NONE',  ( 0.5000000000000003331, 36.00000000000000711, 7.000000000000000000 ) ) ;
#25260=CARTESIAN_POINT ( 'NONE',  ( 10.26940745284089829, 33.04623494220481206, 10.49999999999999822 ) ) ;
#25264=ADVANCED_FACE ( 'NONE', ( #32091 ), #26473, .T. ) ;
#25267=CARTESIAN_POINT ( 'NONE',  ( 7.851720845715640884, 9.718492148735345282, 7.202682876670055023 ) ) ;
#25268=EDGE_CURVE ( 'NONE', #28022, #8314, #29051, .T. ) ;
#25270=DIRECTION ( 'NONE',  ( -0.9135454576426059736, -0.4067366430757887730, 0.000000000000000000 ) ) ;
#25271=ADVANCED_FACE ( 'NONE', ( #14808 ), #34251, .T. ) ;
#25272=AXIS2_PLACEMENT_3D ( 'NONE', #16772, #17386, #29761 ) ;
#25276=CARTESIAN_POINT ( 'NONE',  ( -13.94482798346716201, 26.50521816028930644, 7.499999999999993783 ) ) ;
#25278=VERTEX_POINT ( 'NONE', #5460 ) ;
#25281=DIRECTION ( 'NONE',  ( 0.000000000000000000, 0.000000000000000000, -1.000000000000000000 ) ) ;
#25292=EDGE_CURVE ( 'NONE', #28965, #11507, #29241, .T. ) ;
#25293=VERTEX_POINT ( 'NONE', #29441 ) ;
#25300=CARTESIAN_POINT ( 'NONE',  ( 12.30736835487432579, 14.81698729810772619, 7.000000000000000000 ) ) ;
#25301=DIRECTION ( 'NONE',  ( 0.2876062384759450752, -0.6459741880212618304, -0.7071067811865399122 ) ) ;
#25304=FACE_OUTER_BOUND ( 'NONE', #35655, .T. ) ;
#25305=CARTESIAN_POINT ( 'NONE',  ( -3.503793317224517700, 8.420815634768727520, 9.000000000000001776 ) ) ;
#25307=CARTESIAN_POINT ( 'NONE',  ( -8.410254037844435260, 17.06698729810786475, 10.50000000000000178 ) ) ;
#25308=ORIENTED_EDGE ( 'NONE', *, *, #15748, .T. ) ;
#25310=DIRECTION ( 'NONE',  ( 0.000000000000000000, 0.000000000000000000, 1.000000000000000000 ) ) ;
#25311=CARTESIAN_POINT ( 'NONE',  ( 12.88757880222261321, 15.63670317852378489, 10.99387789255783510 ) ) ;
#25316=EDGE_LOOP ( 'NONE', ( #20380, #34114, #10995 ) ) ;
#25319=AXIS2_PLACEMENT_3D ( 'NONE', #37545, #15806, #12161 ) ;
#25325=CARTESIAN_POINT ( 'NONE',  ( 11.48173768534036121, 32.16538668264416145, 10.49999999999999822 ) ) ;
#25327=ORIENTED_EDGE ( 'NONE', *, *, #26611, .F. ) ;
#25330=ORIENTED_EDGE ( 'NONE', *, *, #31146, .T. ) ;
#25332=LINE ( 'NONE', #9709, #31685 ) ;
#25333=VECTOR ( 'NONE', #6310, 1000.000000000000000 ) ;
#25339=CARTESIAN_POINT ( 'NONE',  ( -1.000000000000000000, 37.50000000000000711, 11.00000000000000000 ) ) ;
#25340=CARTESIAN_POINT ( 'NONE',  ( 14.97283171447379146, 21.48159823030311344, 11.00000000000000000 ) ) ;
#25342=DIRECTION ( 'NONE',  ( -1.000000000000000000, 0.000000000000000000, 0.000000000000000000 ) ) ;
#25343=VERTEX_POINT ( 'NONE', #39586 ) ;
#25345=VECTOR ( 'NONE', #8872, 999.9999999999998863 ) ;
#25346=CARTESIAN_POINT ( 'NONE',  ( 8.118377661053333583, 10.47536095541699197, 11.00000000000000000 ) ) ;
#25347=DIRECTION ( 'NONE',  ( -0.1045284632676436315, 0.9945218953682742891, 0.000000000000000000 ) ) ;
#25348=DIRECTION ( 'NONE',  ( 0.1470157664652037011, 0.6916548014802281763, -0.7071067811865437980 ) ) ;
#25349=DIRECTION ( 'NONE',  ( 0.000000000000000000, 0.000000000000000000, -1.000000000000000000 ) ) ;
#25350=LINE ( 'NONE', #34507, #10625 ) ;
#25352=ORIENTED_EDGE ( 'NONE', *, *, #159, .T. ) ;
#25356=CARTESIAN_POINT ( 'NONE',  ( -9.303655249773278513, 10.73386218874833808, 7.000000000000000000 ) ) ;
#25360=CARTESIAN_POINT ( 'NONE',  ( 0.5000000000000005551, 33.00000000000000000, 10.50000000000000000 ) ) ;
#25366=CARTESIAN_POINT ( 'NONE',  ( 13.52529089031629184, 27.94609563178149614, 10.49999999999999822 ) ) ;
#25367=DIRECTION ( 'NONE',  ( -0.000000000000000000, -0.000000000000000000, -1.000000000000000000 ) ) ;
#25368=EDGE_LOOP ( 'NONE', ( #28081, #20003, #28453 ) ) ;
#25370=FACE_OUTER_BOUND ( 'NONE', #18411, .T. ) ;
#25371=CARTESIAN_POINT ( 'NONE',  ( 14.97009266215792067, 21.42933399866928923, 10.49999999999999112 ) ) ;
#25372=ORIENTED_EDGE ( 'NONE', *, *, #18248, .F. ) ;
#25374=EDGE_CURVE ( 'NONE', #26679, #2909, #14610, .T. ) ;
#25376=CARTESIAN_POINT ( 'NONE',  ( 4.096822963000107620, 8.035697679810645866, 10.50000000000000000 ) ) ;
#25377=DIRECTION ( 'NONE',  ( 0.9945218953682742891, 0.1045284632676437564, 0.000000000000000000 ) ) ;
#25379=ORIENTED_EDGE ( 'NONE', *, *, #35032, .F. ) ;
#25381=CARTESIAN_POINT ( 'NONE',  ( -11.44473057578096942, 31.45924896672619298, 7.500000000000004441 ) ) ;
#25387=DIRECTION ( 'NONE',  ( -0.000000000000000000, -0.000000000000000000, 1.000000000000000000 ) ) ;
#25389=CARTESIAN_POINT ( 'NONE',  ( -4.984135866956332706, 36.15314577889358105, 9.500000000000000000 ) ) ;
#25391=CARTESIAN_POINT ( 'NONE',  ( 3.585007771387210607, 8.038731668389077711, 10.82238861112335471 ) ) ;
#25393=EDGE_CURVE ( 'NONE', #28064, #11564, #14797, .T. ) ;
#25395=EDGE_CURVE ( 'NONE', #8749, #36443, #5995, .T. ) ;
#25396=DIRECTION ( 'NONE',  ( -0.000000000000000000, -0.000000000000000000, -1.000000000000000000 ) ) ;
#25399=VECTOR ( 'NONE', #19912, 1000.000000000000114 ) ;
#25405=VERTEX_POINT ( 'NONE', #11563 ) ;
#25411=ORIENTED_EDGE ( 'NONE', *, *, #35765, .F. ) ;
#25412=VERTEX_POINT ( 'NONE', #29642 ) ;
#25414=CARTESIAN_POINT ( 'NONE',  ( -6.407695755496608747, 35.66262363504867494, 10.99999999999999467 ) ) ;
#25415=EDGE_CURVE ( 'NONE', #16860, #7168, #26596, .T. ) ;
#25419=LINE ( 'NONE', #19329, #5363 ) ;
#25420=VERTEX_POINT ( 'NONE', #39186 ) ;
#25426=ORIENTED_EDGE ( 'NONE', *, *, #11912, .F. ) ;
#25430=ORIENTED_EDGE ( 'NONE', *, *, #162, .F. ) ;
#25433=DIRECTION ( 'NONE',  ( -0.000000000000000000, -0.000000000000000000, -1.000000000000000000 ) ) ;
#25435=CIRCLE ( 'NONE', #16348, 15.00000000000000000 ) ;
#25436=CARTESIAN_POINT ( 'NONE',  ( -7.611215932167762155, 18.68301270189229513, 9.000000000000001776 ) ) ;
#25437=EDGE_CURVE ( 'NONE', #1824, #4212, #35577, .T. ) ;
#25442=CARTESIAN_POINT ( 'NONE',  ( -3.295881626406750087, 9.398963235502531433, 9.500000000000000000 ) ) ;
#25444=EDGE_LOOP ( 'NONE', ( #37918, #7042, #36045, #7577 ) ) ;
#25448=CARTESIAN_POINT ( 'NONE',  ( -3.503793317224518145, 8.420815634768723967, 7.000000000000000000 ) ) ;
#25453=ORIENTED_EDGE ( 'NONE', *, *, #26135, .F. ) ;
#25455=CARTESIAN_POINT ( 'NONE',  ( 8.188662802687307618, 9.932154366953152902, 7.455539900862802050 ) ) ;
#25457=EDGE_CURVE ( 'NONE', #24423, #7663, #36856, .T. ) ;
#25458=CARTESIAN_POINT ( 'NONE',  ( -12.68475447279705648, 27.14725768220950286, 10.50000000000000000 ) ) ;
#25459=CIRCLE ( 'NONE', #6667, 0.5000000000000004441 ) ;
#25463=CARTESIAN_POINT ( 'NONE',  ( 7.468455364333221880, 29.89744377950669474, 11.00000000000000000 ) ) ;
#25465=ORIENTED_EDGE ( 'NONE', *, *, #34498, .F. ) ;
#25467=CARTESIAN_POINT ( 'NONE',  ( 11.69134295108989186, 15.74999999999995204, 7.000000000000000000 ) ) ;
#25469=CARTESIAN_POINT ( 'NONE',  ( -2.518583951651248931, 7.712953814960721743, 7.499999999999997335 ) ) ;
#25470=DIRECTION ( 'NONE',  ( 1.000000000000000000, 0.000000000000000000, 0.000000000000000000 ) ) ;
#25471=VERTEX_POINT ( 'NONE', #15405 ) ;
#25474=AXIS2_PLACEMENT_3D ( 'NONE', #25823, #28472, #6530 ) ;
#25476=ORIENTED_EDGE ( 'NONE', *, *, #31611, .F. ) ;
#25478=DIRECTION ( 'NONE',  ( 0.000000000000000000, 0.000000000000000000, 1.000000000000000000 ) ) ;
#25479=ORIENTED_EDGE ( 'NONE', *, *, #31240, .T. ) ;
#25481=EDGE_CURVE ( 'NONE', #25659, #36019, #3214, .T. ) ;
#25486=CARTESIAN_POINT ( 'NONE',  ( 3.295881626406585774, 9.398963235502479918, 7.000000000000000000 ) ) ;
#25487=ORIENTED_EDGE ( 'NONE', *, *, #27020, .F. ) ;
#25488=CARTESIAN_POINT ( 'NONE',  ( -6.713764256189716839, 35.89999254728751055, 10.49999999999999822 ) ) ;
#25489=AXIS2_PLACEMENT_3D ( 'NONE', #18777, #31167, #291 ) ;
#25490=LINE ( 'NONE', #24905, #11021 ) ;
#25492=CARTESIAN_POINT ( 'NONE',  ( -7.824485034907247893, 10.87986945260456473, 7.500000000000000888 ) ) ;
#25496=CARTESIAN_POINT ( 'NONE',  ( 5.068835528549737290, 13.82204480395803081, 10.49999999999999822 ) ) ;
#25501=CARTESIAN_POINT ( 'NONE',  ( 13.14565515434632026, 15.48770272715369956, 10.82238861112334938 ) ) ;
#25503=DIRECTION ( 'NONE',  ( -0.000000000000000000, -0.000000000000000000, -1.000000000000000000 ) ) ;
#25507=ORIENTED_EDGE ( 'NONE', *, *, #5023, .T. ) ;
#25508=CARTESIAN_POINT ( 'NONE',  ( 14.38243823352023476, 26.25560849141422182, 10.49999999999999822 ) ) ;
#25510=ADVANCED_FACE ( 'NONE', ( #3406 ), #18658, .T. ) ;
#25516=EDGE_LOOP ( 'NONE', ( #32875, #2871, #22581, #13989 ) ) ;
#25521=VERTEX_POINT ( 'NONE', #33712 ) ;
#25524=EDGE_CURVE ( 'NONE', #2211, #12521, #39981, .T. ) ;
#25526=ORIENTED_EDGE ( 'NONE', *, *, #19039, .F. ) ;
#25529=CARTESIAN_POINT ( 'NONE',  ( 12.80736835487433289, 15.68301270189216545, 7.000000000000000000 ) ) ;
#25532=TOROIDAL_SURFACE ( 'NONE', #8023, 1.000000000000000000, 0.5000000000000000000 ) ;
#25534=ORIENTED_EDGE ( 'NONE', *, *, #3954, .T. ) ;
#25535=DIRECTION ( 'NONE',  ( -0.8090169943749426773, 0.5877852522924797984, 0.000000000000000000 ) ) ;
#25537=EDGE_CURVE ( 'NONE', #9089, #17047, #22576, .T. ) ;
#25539=DIRECTION ( 'NONE',  ( 1.000000000000000000, 0.000000000000000000, 0.000000000000000000 ) ) ;
#25540=ORIENTED_EDGE ( 'NONE', *, *, #22527, .F. ) ;
#25541=CIRCLE ( 'NONE', #7354, 15.00000000000000000 ) ;
#25543=CARTESIAN_POINT ( 'NONE',  ( -14.01196168477328641, 27.85442546840040734, 7.455539900862793168 ) ) ;
#25544=DIRECTION ( 'NONE',  ( -0.6459741880212603871, -0.2876062384759424106, -0.7071067811865422437 ) ) ;
#25547=CARTESIAN_POINT ( 'NONE',  ( -9.363324537585850038, 32.27640801132209702, 9.500000000000000000 ) ) ;
#25550=DIRECTION ( 'NONE',  ( -0.9135454576426051965, -0.4067366430757904938, 0.000000000000000000 ) ) ;
#25551=ORIENTED_EDGE ( 'NONE', *, *, #37830, .F. ) ;
#25553=FACE_OUTER_BOUND ( 'NONE', #29470, .T. ) ;
#25554=DIRECTION ( 'NONE',  ( 1.000000000000000000, 0.000000000000000000, 0.000000000000000000 ) ) ;
#25557=CARTESIAN_POINT ( 'NONE',  ( -9.331903152615899089, 11.35703883385581037, 7.500000000000000888 ) ) ;
#25560=CARTESIAN_POINT ( 'NONE',  ( 9.393455880287467252, 11.27231877233265323, 10.49999999999999822 ) ) ;
#25566=EDGE_CURVE ( 'NONE', #10996, #32239, #21945, .T. ) ;
#25568=CARTESIAN_POINT ( 'NONE',  ( 14.00731263743715793, 27.57698287931455994, 10.82238861112332629 ) ) ;
#25569=DIRECTION ( 'NONE',  ( -0.2079116908177516265, 0.9781476007338072431, 0.000000000000000000 ) ) ;
#25570=ORIENTED_EDGE ( 'NONE', *, *, #32615, .F. ) ;
#25572=VECTOR ( 'NONE', #36010, 1000.000000000000000 ) ;
#25573=FACE_OUTER_BOUND ( 'NONE', #6090, .T. ) ;
#25574=ORIENTED_EDGE ( 'NONE', *, *, #20432, .F. ) ;
#25577=LINE ( 'NONE', #31481, #30360 ) ;
#25578=ORIENTED_EDGE ( 'NONE', *, *, #38231, .T. ) ;
#25583=AXIS2_PLACEMENT_3D ( 'NONE', #10177, #22552, #3873 ) ;
#25587=CARTESIAN_POINT ( 'NONE',  ( 8.118377661053324701, 10.47536095541698486, 7.000000000000000000 ) ) ;
#25588=CARTESIAN_POINT ( 'NONE',  ( -8.238488885696254371, 24.65111619403957022, 9.000000000000001776 ) ) ;
#25590=AXIS2_PLACEMENT_3D ( 'NONE', #18123, #30309, #18715 ) ;
#25591=DIRECTION ( 'NONE',  ( -1.000000000000000000, 0.000000000000000000, 0.000000000000000000 ) ) ;
#25592=ORIENTED_EDGE ( 'NONE', *, *, #7273, .T. ) ;
#25593=DIRECTION ( 'NONE',  ( 1.000000000000000000, 0.000000000000000000, 0.000000000000000000 ) ) ;
#25595=DIRECTION ( 'NONE',  ( -0.000000000000000000, -0.000000000000000000, -1.000000000000000000 ) ) ;
#25597=DIRECTION ( 'NONE',  ( -0.000000000000000000, -0.000000000000000000, 1.000000000000000000 ) ) ;
#25600=VERTEX_POINT ( 'NONE', #9111 ) ;
#25602=PLANE ( 'NONE',  #6782 ) ;
#25605=ORIENTED_EDGE ( 'NONE', *, *, #22281, .T. ) ;
#25609=DIRECTION ( 'NONE',  ( -0.000000000000000000, -0.000000000000000000, -1.000000000000000000 ) ) ;
#25611=ORIENTED_EDGE ( 'NONE', *, *, #38079, .F. ) ;
#25613=VECTOR ( 'NONE', #2981, 1000.000000000000000 ) ;
#25616=VECTOR ( 'NONE', #2771, 1000.000000000000000 ) ;
#25618=FACE_OUTER_BOUND ( 'NONE', #15326, .T. ) ;
#25621=CARTESIAN_POINT ( 'NONE',  ( -8.137585970691988635, 29.15429895402941085, 10.00000000000000000 ) ) ;
#25622=DIRECTION ( 'NONE',  ( 0.000000000000000000, 0.000000000000000000, 1.000000000000000000 ) ) ;
#25623=ADVANCED_FACE ( 'NONE', ( #24742 ), #34096, .F. ) ;
#25624=ORIENTED_EDGE ( 'NONE', *, *, #19067, .T. ) ;
#25631=ORIENTED_EDGE ( 'NONE', *, *, #12633, .T. ) ;
#25633=CARTESIAN_POINT ( 'NONE',  ( -6.404490139165758045, 34.42612703509939820, 10.50000000000000000 ) ) ;
#25634=AXIS2_PLACEMENT_3D ( 'NONE', #1856, #14234, #39016 ) ;
#25636=PLANE ( 'NONE',  #6426 ) ;
#25638=DIRECTION ( 'NONE',  ( 0.000000000000000000, 0.000000000000000000, -1.000000000000000000 ) ) ;
#25640=CIRCLE ( 'NONE', #21760, 0.5000000000000004441 ) ;
#25643=ADVANCED_FACE ( 'NONE', ( #31050 ), #33902, .T. ) ;
#25649=CARTESIAN_POINT ( 'NONE',  ( -4.780767545418437514, 35.69637305007227468, 10.50000000000000000 ) ) ;
#25658=DIRECTION ( 'NONE',  ( -0.3090169943749573878, -0.9510565162951503115, 0.000000000000000000 ) ) ;
#25659=VERTEX_POINT ( 'NONE', #165 ) ;
#25661=CARTESIAN_POINT ( 'NONE',  ( -14.91650131011210156, 21.43496667674312306, 10.76099332938164288 ) ) ;
#25663=DIRECTION ( 'NONE',  ( 1.000000000000000000, 0.000000000000000000, 0.000000000000000000 ) ) ;
#25669=ORIENTED_EDGE ( 'NONE', *, *, #11064, .F. ) ;
#25672=ADVANCED_FACE ( 'NONE', ( #12554 ), #8915, .T. ) ;
#25673=LINE ( 'NONE', #34825, #38764 ) ;
#25675=AXIS2_PLACEMENT_3D ( 'NONE', #7166, #1087, #28909 ) ;
#25676=ORIENTED_EDGE ( 'NONE', *, *, #39560, .T. ) ;
#25682=AXIS2_PLACEMENT_3D ( 'NONE', #33918, #18279, #30672 ) ;
#25685=CYLINDRICAL_SURFACE ( 'NONE', #31632, 0.5000000000000004441 ) ;
#25687=DIRECTION ( 'NONE',  ( 0.9135454576426004225, -0.4067366430758009854, 0.000000000000000000 ) ) ;
#25697=AXIS2_PLACEMENT_3D ( 'NONE', #7928, #4488, #29067 ) ;
#25698=DIRECTION ( 'NONE',  ( 1.000000000000000000, 0.000000000000000000, 0.000000000000000000 ) ) ;
#25699=CARTESIAN_POINT ( 'NONE',  ( 11.87435565298210882, 15.06698729810772619, 9.500000000000000000 ) ) ;
#25701=LINE ( 'NONE', #12520, #16553 ) ;
#25704=VECTOR ( 'NONE', #14131, 1000.000000000000000 ) ;
#25709=DIRECTION ( 'NONE',  ( 0.6847716512521591081, 0.4446959099295441087, 0.5773502691896197359 ) ) ;
#25713=ORIENTED_EDGE ( 'NONE', *, *, #2542, .T. ) ;
#25715=CARTESIAN_POINT ( 'NONE',  ( 14.45052027064708255, 26.47704597190804066, 10.49999999999999822 ) ) ;
#25721=ORIENTED_EDGE ( 'NONE', *, *, #2844, .T. ) ;
#25724=ADVANCED_FACE ( 'NONE', ( #31987 ), #13907, .T. ) ;
#25735=AXIS2_PLACEMENT_3D ( 'NONE', #2503, #31273, #15082 ) ;
#25736=VERTEX_POINT ( 'NONE', #11071 ) ;
#25738=CARTESIAN_POINT ( 'NONE',  ( -12.05736835487443237, 14.38397459621567442, 7.499999999999993783 ) ) ;
#25740=EDGE_CURVE ( 'NONE', #4731, #21130, #29106, .T. ) ;
#25741=DIRECTION ( 'NONE',  ( 0.000000000000000000, 0.000000000000000000, -1.000000000000000000 ) ) ;
#25743=EDGE_CURVE ( 'NONE', #3918, #36944, #19594, .T. ) ;
#25746=DIRECTION ( 'NONE',  ( 0.7431448254773961315, 0.6691306063588561281, 0.000000000000000000 ) ) ;
#25749=PLANE ( 'NONE',  #37194 ) ;
#25751=CARTESIAN_POINT ( 'NONE',  ( 2.629601561899395534, 7.723830143584016206, 10.49999999999999822 ) ) ;
#25753=ADVANCED_FACE ( 'NONE', ( #17172 ), #12861, .T. ) ;
#25769=EDGE_CURVE ( 'NONE', #15233, #12521, #21316, .T. ) ;
#25770=ORIENTED_EDGE ( 'NONE', *, *, #13737, .T. ) ;
#25772=AXIS2_PLACEMENT_3D ( 'NONE', #29191, #35285, #25930 ) ;
#25775=EDGE_CURVE ( 'NONE', #14003, #11406, #39464, .T. ) ;
#25776=AXIS2_PLACEMENT_3D ( 'NONE', #20475, #39351, #23911 ) ;
#25777=DIRECTION ( 'NONE',  ( 1.000000000000000000, 0.000000000000000000, 0.000000000000000000 ) ) ;
#25778=ORIENTED_EDGE ( 'NONE', *, *, #25415, .F. ) ;
#25780=LINE ( 'NONE', #10346, #29087 ) ;
#25781=FACE_OUTER_BOUND ( 'NONE', #20309, .T. ) ;
#25782=ORIENTED_EDGE ( 'NONE', *, *, #16084, .F. ) ;
#25785=ORIENTED_EDGE ( 'NONE', *, *, #18014, .T. ) ;
#25787=VERTEX_POINT ( 'NONE', #22095 ) ;
#25791=DIRECTION ( 'NONE',  ( -0.000000000000000000, -0.000000000000000000, -1.000000000000000000 ) ) ;
#25792=ADVANCED_FACE ( 'NONE', ( #4765 ), #32341, .T. ) ;
#25794=AXIS2_PLACEMENT_3D ( 'NONE', #11800, #14041, #30292 ) ;
#25797=ORIENTED_EDGE ( 'NONE', *, *, #1972, .T. ) ;
#25800=DIRECTION ( 'NONE',  ( 0.000000000000000000, 0.000000000000000000, -1.000000000000000000 ) ) ;
#25804=AXIS2_PLACEMENT_3D ( 'NONE', #22223, #307, #20349 ) ;
#25806=ORIENTED_EDGE ( 'NONE', *, *, #2053, .F. ) ;
#25807=DIRECTION ( 'NONE',  ( -0.3090169943749573878, -0.9510565162951503115, 0.000000000000000000 ) ) ;
#25808=DIRECTION ( 'NONE',  ( 0.4731467892558156030, -0.5254827454987647251, -0.7071067811865427988 ) ) ;
#25811=CARTESIAN_POINT ( 'NONE',  ( -14.62786683182126168, 20.45979510329166828, 10.94611345180490503 ) ) ;
#25816=CARTESIAN_POINT ( 'NONE',  ( -22.32447841415231338, 25.34915137120643180, 11.00000000000000000 ) ) ;
#25820=DIRECTION ( 'NONE',  ( 1.000000000000000000, 0.000000000000000000, -0.000000000000000000 ) ) ;
#25823=CARTESIAN_POINT ( 'NONE',  ( 3.610593701936712474, 31.83882289796390097, 10.50000000000000000 ) ) ;
#25826=CARTESIAN_POINT ( 'NONE',  ( 14.36910708881319110, 26.64307479831611047, 10.76099332938163755 ) ) ;
#25834=CIRCLE ( 'NONE', #13500, 15.00000000000000000 ) ;
#25837=VERTEX_POINT ( 'NONE', #28938 ) ;
#25841=CARTESIAN_POINT ( 'NONE',  ( 5.187504188494417079, 36.60991850771481637, 7.000000000000000000 ) ) ;
#25842=CARTESIAN_POINT ( 'NONE',  ( -10.44103466624267185, 32.57396620494226624, 11.00000000000000000 ) ) ;
#25843=AXIS2_PLACEMENT_3D ( 'NONE', #15629, #31268, #6277 ) ;
#25850=ORIENTED_EDGE ( 'NONE', *, *, #4376, .T. ) ;
#25855=CARTESIAN_POINT ( 'NONE',  ( -1.400691654708310585, 37.43445890845833901, 7.000000000000000000 ) ) ;
#25857=ORIENTED_EDGE ( 'NONE', *, *, #35332, .F. ) ;
#25859=FACE_OUTER_BOUND ( 'NONE', #6255, .T. ) ;
#25862=CARTESIAN_POINT ( 'NONE',  ( -10.10646936306323518, 32.94553861768095970, 7.500000000000004441 ) ) ;
#25864=DIRECTION ( 'NONE',  ( 0.000000000000000000, 0.000000000000000000, -1.000000000000000000 ) ) ;
#25865=ORIENTED_EDGE ( 'NONE', *, *, #6640, .T. ) ;
#25868=LINE ( 'NONE', #10644, #5332 ) ;
#25870=ORIENTED_EDGE ( 'NONE', *, *, #18697, .T. ) ;
#25873=DIRECTION ( 'NONE',  ( -0.000000000000000000, -0.000000000000000000, -1.000000000000000000 ) ) ;
#25875=ORIENTED_EDGE ( 'NONE', *, *, #37956, .T. ) ;
#25877=AXIS2_PLACEMENT_3D ( 'NONE', #20283, #11140, #4838 ) ;
#25879=VECTOR ( 'NONE', #26570, 1000.000000000000000 ) ;
#25880=EDGE_CURVE ( 'NONE', #14950, #2452, #1867, .T. ) ;
#25882=ORIENTED_EDGE ( 'NONE', *, *, #28504, .T. ) ;
#25886=DIRECTION ( 'NONE',  ( -0.9510565162951503115, 0.3090169943749573878, -0.000000000000000000 ) ) ;
#25887=DIRECTION ( 'NONE',  ( 0.6691306063588662312, 0.7431448254773869166, 0.000000000000000000 ) ) ;
#25888=LINE ( 'NONE', #13092, #6505 ) ;
#25889=CARTESIAN_POINT ( 'NONE',  ( 11.81630298851978722, 31.79381426990546089, 10.50000000000000178 ) ) ;
#25890=LINE ( 'NONE', #7812, #26297 ) ;
#25891=EDGE_LOOP ( 'NONE', ( #4391, #1056, #2615, #5369, #34477, #6538, #14709, #26213 ) ) ;
#25892=EDGE_CURVE ( 'NONE', #25343, #8719, #40128, .T. ) ;
#25893=CARTESIAN_POINT ( 'NONE',  ( -6.557822374958133693, 35.99981354310120452, 10.49999999999999822 ) ) ;
#25897=DIRECTION ( 'NONE',  ( -0.4067366430757888285, 0.9135454576426059736, 0.000000000000000000 ) ) ;
#25898=DIRECTION ( 'NONE',  ( 0.05233595624293101850, -0.9986295347545744994, -3.618009791163114596E-16 ) ) ;
#25901=AXIS2_PLACEMENT_3D ( 'NONE', #28946, #10464, #35658 ) ;
#25906=CARTESIAN_POINT ( 'NONE',  ( -7.267999511062860130, 35.13630417120410954, 7.000000000000000000 ) ) ;
#25911=B_SPLINE_SURFACE_WITH_KNOTS ( 'NONE', 1, 3, ( 
 ( #25371, #16648, #37771, #22324, #6878, #29030, #16439, #16243, #28625, #10342 ),
 ( #13384, #37971, #7080, #19478, #12590, #29232, #35737, #29832, #38575, #11150 ) ),
 .UNSPECIFIED., .F., .F., .F.,
 ( 2, 2 ),
 ( 4, 2, 2, 2, 4 ),
 ( 0.000000000000000000, 1.000000000000000000 ),
 ( 1.496612791730134617, 1.889311873428863198, 2.282010955127591778, 2.674710036826319914, 3.067409118525048495 ),
 .UNSPECIFIED. ) ;
#25914=CARTESIAN_POINT ( 'NONE',  ( 14.14332487906622049, 26.04398259919119951, 10.49999999999999822 ) ) ;
#25920=ORIENTED_EDGE ( 'NONE', *, *, #2563, .F. ) ;
#25925=ORIENTED_EDGE ( 'NONE', *, *, #8268, .T. ) ;
#25927=ADVANCED_FACE ( 'NONE', ( #35239 ), #29146, .T. ) ;
#25928=DIRECTION ( 'NONE',  ( 0.9510565162951504226, -0.3090169943749573322, 0.000000000000000000 ) ) ;
#25929=VERTEX_POINT ( 'NONE', #24055 ) ;
#25930=DIRECTION ( 'NONE',  ( -0.6691306063588576825, 0.7431448254773946882, 0.000000000000000000 ) ) ;
#25931=FACE_OUTER_BOUND ( 'NONE', #5132, .T. ) ;
#25934=AXIS2_PLACEMENT_3D ( 'NONE', #12463, #34011, #40092 ) ;
#25939=DIRECTION ( 'NONE',  ( 0.000000000000000000, 0.000000000000000000, 1.000000000000000000 ) ) ;
#25940=CARTESIAN_POINT ( 'NONE',  ( 13.16028273094469192, 27.30176617939681449, 7.000000000000000000 ) ) ;
#25941=ORIENTED_EDGE ( 'NONE', *, *, #32693, .F. ) ;
#25943=CARTESIAN_POINT ( 'NONE',  ( -14.98807736202308227, 21.89862425409926772, 7.338691926023216183 ) ) ;
#25944=DIRECTION ( 'NONE',  ( -0.1045284632676436176, 0.9945218953682742891, 0.000000000000000000 ) ) ;
#25946=PLANE ( 'NONE',  #714 ) ;
#25948=DIRECTION ( 'NONE',  ( -1.000000000000000000, 0.000000000000000000, 0.000000000000000000 ) ) ;
#25951=EDGE_LOOP ( 'NONE', ( #26722, #36107, #2316, #15547 ) ) ;
#25953=DIRECTION ( 'NONE',  ( -0.4999999999999933942, 0.8660254037844425934, 0.000000000000000000 ) ) ;
#25956=CARTESIAN_POINT ( 'NONE',  ( 9.343266739736582949, 17.68301270189218855, 10.50000000000000000 ) ) ;
#25964=CARTESIAN_POINT ( 'NONE',  ( 0.5000000000000001110, 37.00000000000000711, 7.500000000000000888 ) ) ;
#25966=EDGE_LOOP ( 'NONE', ( #12467, #35009, #3494, #11775 ) ) ;
#25967=CIRCLE ( 'NONE', #16937, 6.000000000000003553 ) ;
#25969=ORIENTED_EDGE ( 'NONE', *, *, #20447, .T. ) ;
#25971=CYLINDRICAL_SURFACE ( 'NONE', #27392, 0.5000000000000001110 ) ;
#25974=EDGE_CURVE ( 'NONE', #39672, #2261, #15484, .T. ) ;
#25976=EDGE_CURVE ( 'NONE', #30884, #13873, #22599, .T. ) ;
#25977=CARTESIAN_POINT ( 'NONE',  ( -12.30736835487442704, 14.81698729810789672, 7.000000000000000000 ) ) ;
#25980=ORIENTED_EDGE ( 'NONE', *, *, #15553, .T. ) ;
#25982=AXIS2_PLACEMENT_3D ( 'NONE', #34794, #34592, #3313 ) ;
#25983=ADVANCED_FACE ( 'NONE', ( #8212 ), #21205, .T. ) ;
#25984=CIRCLE ( 'NONE', #21469, 6.000000000000001776 ) ;
#25988=LINE ( 'NONE', #35142, #6706 ) ;
#25989=DIRECTION ( 'NONE',  ( -0.6293203910498448295, -0.7771459614569649066, 0.000000000000000000 ) ) ;
#25991=CYLINDRICAL_SURFACE ( 'NONE', #27201, 6.000000000000015987 ) ;
#25992=ORIENTED_EDGE ( 'NONE', *, *, #22920, .F. ) ;
#25993=DIRECTION ( 'NONE',  ( 0.2876062384759449642, -0.6459741880212592768, -0.7071067811865424657 ) ) ;
#25995=CIRCLE ( 'NONE', #30548, 6.000000000000003553 ) ;
#25996=ADVANCED_FACE ( 'NONE', ( #30559 ), #33216, .T. ) ;
#25997=FACE_OUTER_BOUND ( 'NONE', #23380, .T. ) ;
#26002=CARTESIAN_POINT ( 'NONE',  ( 8.137585970692077453, 29.15429895402930072, 10.00000000000000000 ) ) ;
#26006=LINE ( 'NONE', #1639, #1680 ) ;
#26007=EDGE_LOOP ( 'NONE', ( #6139, #28006, #26622, #23144 ) ) ;
#26013=LINE ( 'NONE', #10789, #1065 ) ;
#26014=ORIENTED_EDGE ( 'NONE', *, *, #31965, .F. ) ;
#26018=EDGE_CURVE ( 'NONE', #37387, #42, #2327, .T. ) ;
#26021=CARTESIAN_POINT ( 'NONE',  ( -4.984135866956334482, 36.15314577889358105, 7.500000000000000888 ) ) ;
#26022=ORIENTED_EDGE ( 'NONE', *, *, #24763, .T. ) ;
#26026=CYLINDRICAL_SURFACE ( 'NONE', #10216, 0.5000000000000006661 ) ;
#26028=EDGE_LOOP ( 'NONE', ( #130, #2299, #6031, #38237 ) ) ;
#26030=CARTESIAN_POINT ( 'NONE',  ( -5.644276917315582232, 36.40655018617695760, 10.59344459855552678 ) ) ;
#26031=EDGE_LOOP ( 'NONE', ( #24146, #2427, #15671, #35994 ) ) ;
#26033=EDGE_CURVE ( 'NONE', #26924, #21498, #20815, .T. ) ;
#26041=VECTOR ( 'NONE', #9524, 1000.000000000000000 ) ;
#26042=LINE ( 'NONE', #25841, #4463 ) ;
#26044=FACE_OUTER_BOUND ( 'NONE', #39202, .T. ) ;
#26046=CARTESIAN_POINT ( 'NONE',  ( -2.629601561899595374, 7.723830143584053509, 10.49999999999999822 ) ) ;
#26049=AXIS2_PLACEMENT_3D ( 'NONE', #20547, #32940, #26830 ) ;
#26054=ORIENTED_EDGE ( 'NONE', *, *, #19201, .F. ) ;
#26057=CARTESIAN_POINT ( 'NONE',  ( 10.73132186042472469, 32.83534196859159238, 10.82238861112332273 ) ) ;
#26059=ORIENTED_EDGE ( 'NONE', *, *, #9312, .T. ) ;
#26062=ORIENTED_EDGE ( 'NONE', *, *, #11983, .T. ) ;
#26064=DIRECTION ( 'NONE',  ( 0.1045284632676570929, 0.9945218953682730678, 0.000000000000000000 ) ) ;
#26066=CARTESIAN_POINT ( 'NONE',  ( 13.53204082366770855, 16.02694346567353634, 7.203056206335837430 ) ) ;
#26074=ADVANCED_FACE ( 'NONE', ( #6350 ), #12896, .T. ) ;
#26077=VERTEX_POINT ( 'NONE', #10006 ) ;
#26081=ORIENTED_EDGE ( 'NONE', *, *, #38926, .F. ) ;
#26085=FACE_OUTER_BOUND ( 'NONE', #5770, .T. ) ;
#26086=CIRCLE ( 'NONE', #807, 0.4999999999999986122 ) ;
#26088=AXIS2_PLACEMENT_3D ( 'NONE', #21007, #2323, #11464 ) ;
#26089=CARTESIAN_POINT ( 'NONE',  ( 12.41947502333593967, 43.35441443594645250, 7.500000000000000888 ) ) ;
#26091=CIRCLE ( 'NONE', #31300, 0.5000000000000000000 ) ;
#26092=DIRECTION ( 'NONE',  ( -0.9510565162951504226, 0.3090169943749573322, 0.000000000000000000 ) ) ;
#26094=EDGE_LOOP ( 'NONE', ( #6874, #36611, #31756, #29627 ) ) ;
#26095=CARTESIAN_POINT ( 'NONE',  ( -6.843305518951122046, 35.42677428760902103, 10.49999999999999822 ) ) ;
#26098=ADVANCED_FACE ( 'NONE', ( #9615 ), #9811, .T. ) ;
#26099=FACE_OUTER_BOUND ( 'NONE', #10019, .T. ) ;
#26100=DIRECTION ( 'NONE',  ( -0.6724985119639614872, -0.2185080122244129619, -0.7071067811865427988 ) ) ;
#26102=FACE_OUTER_BOUND ( 'NONE', #28824, .T. ) ;
#26103=ORIENTED_EDGE ( 'NONE', *, *, #39545, .F. ) ;
#26106=VECTOR ( 'NONE', #1955, 1000.000000000000000 ) ;
#26109=CARTESIAN_POINT ( 'NONE',  ( 14.35088184066152373, 20.32132268570678235, 10.83333333333333393 ) ) ;
#26111=EDGE_LOOP ( 'NONE', ( #5898, #24481, #31556 ) ) ;
#26114=VERTEX_POINT ( 'NONE', #6943 ) ;
#26128=ORIENTED_EDGE ( 'NONE', *, *, #28134, .F. ) ;
#26131=CIRCLE ( 'NONE', #71, 0.4999999999999997780 ) ;
#26134=CARTESIAN_POINT ( 'NONE',  ( 8.339609403135806787, 11.87216320208440123, 9.500000000000000000 ) ) ;
#26135=EDGE_CURVE ( 'NONE', #34064, #39672, #18951, .T. ) ;
#26137=CONICAL_SURFACE ( 'NONE', #24838, 1.000000000000007772, 0.7853981633974557175 ) ;
#26139=VECTOR ( 'NONE', #31500, 1000.000000000000114 ) ;
#26141=CARTESIAN_POINT ( 'NONE',  ( 8.118377661053324701, 10.47536095541698486, 9.000000000000001776 ) ) ;
#26144=DIRECTION ( 'NONE',  ( 0.7431448254773962425, 0.6691306063588561281, 0.000000000000000000 ) ) ;
#26145=ORIENTED_EDGE ( 'NONE', *, *, #24142, .F. ) ;
#26147=CARTESIAN_POINT ( 'NONE',  ( -13.93689154498694904, 28.04681619138562709, 7.338691926023206413 ) ) ;
#26149=DIRECTION ( 'NONE',  ( 1.000000000000000000, 0.000000000000000000, 0.000000000000000000 ) ) ;
#26150=CARTESIAN_POINT ( 'NONE',  ( 14.47283171447379146, 21.48159823030312054, 11.00000000000000000 ) ) ;
#26151=CARTESIAN_POINT ( 'NONE',  ( -19.48557158514982390, 33.75000000000009948, 11.00000000000000000 ) ) ;
#26152=VECTOR ( 'NONE', #8068, 1000.000000000000000 ) ;
#26153=DIRECTION ( 'NONE',  ( -0.000000000000000000, -0.000000000000000000, -1.000000000000000000 ) ) ;
#26155=CARTESIAN_POINT ( 'NONE',  ( -12.69371393710745011, 14.59393057220544776, 10.76099332938163933 ) ) ;
#26156=ORIENTED_EDGE ( 'NONE', *, *, #21487, .T. ) ;
#26158=FACE_OUTER_BOUND ( 'NONE', #14894, .T. ) ;
#26160=EDGE_CURVE ( 'NONE', #37653, #13704, #25222, .T. ) ;
#26161=CARTESIAN_POINT ( 'NONE',  ( -0.4999999999999998890, 37.47223625998407925, 10.68306085400112693 ) ) ;
#26163=ADVANCED_FACE ( 'NONE', ( #18759 ), #11631, .T. ) ;
#26173=CARTESIAN_POINT ( 'NONE',  ( 3.813962023474619212, 32.29559562678521445, 11.00000000000000000 ) ) ;
#26177=ORIENTED_EDGE ( 'NONE', *, *, #38814, .F. ) ;
#26179=DIRECTION ( 'NONE',  ( 0.1045284632676436454, -0.9945218953682745111, 0.000000000000000000 ) ) ;
#26180=EDGE_LOOP ( 'NONE', ( #22486, #31683, #32377, #15636 ) ) ;
#26181=CARTESIAN_POINT ( 'NONE',  ( -4.188939243032556270, 44.61227686191953268, 11.00000000000000000 ) ) ;
#26182=EDGE_CURVE ( 'NONE', #34284, #39323, #34396, .T. ) ;
#26184=ADVANCED_FACE ( 'NONE', ( #37244 ), #37043, .F. ) ;
#26185=ORIENTED_EDGE ( 'NONE', *, *, #2867, .T. ) ;
#26187=ORIENTED_EDGE ( 'NONE', *, *, #7884, .F. ) ;
#26189=AXIS2_PLACEMENT_3D ( 'NONE', #1887, #23000, #14059 ) ;
#26190=ORIENTED_EDGE ( 'NONE', *, *, #36357, .T. ) ;
#26194=LINE ( 'NONE', #7503, #11708 ) ;
#26196=CIRCLE ( 'NONE', #6721, 0.5000000000000004441 ) ;
#26197=DIRECTION ( 'NONE',  ( -0.000000000000000000, -0.000000000000000000, -1.000000000000000000 ) ) ;
#26200=CARTESIAN_POINT ( 'NONE',  ( -2.629601561899596263, 7.723830143584054397, 10.63089969389957012 ) ) ;
#26201=DIRECTION ( 'NONE',  ( 0.8660254037844364872, -0.5000000000000038858, 0.000000000000000000 ) ) ;
#26202=EDGE_CURVE ( 'NONE', #26207, #37486, #27895, .T. ) ;
#26206=VECTOR ( 'NONE', #3752, 1000.000000000000000 ) ;
#26207=VERTEX_POINT ( 'NONE', #69 ) ;
#26211=CARTESIAN_POINT ( 'NONE',  ( -14.36830325120615903, 20.48707633493503621, 11.00000000000000000 ) ) ;
#26212=FACE_OUTER_BOUND ( 'NONE', #27571, .T. ) ;
#26213=ORIENTED_EDGE ( 'NONE', *, *, #19067, .F. ) ;
#26218=CARTESIAN_POINT ( 'NONE',  ( -9.584141256673788689, 10.96086782047184727, 7.338980292232258229 ) ) ;
#26220=VERTEX_POINT ( 'NONE', #12656 ) ;
#26222=DIRECTION ( 'NONE',  ( 0.1045284632676436593, -0.9945218953682742891, 0.000000000000000000 ) ) ;
#26223=CARTESIAN_POINT ( 'NONE',  ( -12.64565515434644105, 14.62167732336942194, 10.82238861112330675 ) ) ;
#26227=VERTEX_POINT ( 'NONE', #28294 ) ;
#26229=CARTESIAN_POINT ( 'NONE',  ( -10.32110986824222110, 33.06327772184317126, 10.49999999999999822 ) ) ;
#26230=CYLINDRICAL_SURFACE ( 'NONE', #36911, 0.5000000000000004441 ) ;
#26231=CARTESIAN_POINT ( 'NONE',  ( 12.05736835487432579, 14.38397459621550567, 7.499999999999997335 ) ) ;
#26232=ORIENTED_EDGE ( 'NONE', *, *, #2234, .T. ) ;
#26234=LINE ( 'NONE', #27042, #28053 ) ;
#26235=VERTEX_POINT ( 'NONE', #21794 ) ;
#26241=VERTEX_POINT ( 'NONE', #31150 ) ;
#26244=LINE ( 'NONE', #10409, #24089 ) ;
#26246=CARTESIAN_POINT ( 'NONE',  ( 7.133890061153791429, 30.26901619224539175, 10.49999999999999645 ) ) ;
#26247=CARTESIAN_POINT ( 'NONE',  ( 14.36830325120613594, 20.48707633493483371, 7.000000000000000000 ) ) ;
#26252=DIRECTION ( 'NONE',  ( -0.6459741880212604981, -0.2876062384759471291, 0.7071067811865402453 ) ) ;
#26253=EDGE_CURVE ( 'NONE', #37413, #7636, #471, .T. ) ;
#26257=CARTESIAN_POINT ( 'NONE',  ( 11.11016527260166420, 31.83082137946473367, 7.000000000000000000 ) ) ;
#26259=CARTESIAN_POINT ( 'NONE',  ( -9.697889840765284930, 31.90483559858339646, 7.000000000000000000 ) ) ;
#26260=ORIENTED_EDGE ( 'NONE', *, *, #36068, .F. ) ;
#26262=ORIENTED_EDGE ( 'NONE', *, *, #34957, .T. ) ;
#26263=TOROIDAL_SURFACE ( 'NONE', #38619, 1.000000000000000000, 0.5000000000000000000 ) ;
#26269=ORIENTED_EDGE ( 'NONE', *, *, #37982, .F. ) ;
#26276=ORIENTED_EDGE ( 'NONE', *, *, #19639, .T. ) ;
#26279=CARTESIAN_POINT ( 'NONE',  ( 12.68475447279710799, 27.14725768220933944, 7.000000000000000000 ) ) ;
#26281=ORIENTED_EDGE ( 'NONE', *, *, #24007, .T. ) ;
#26283=CARTESIAN_POINT ( 'NONE',  ( -0.5000000000000004441, 36.00000000000000711, 7.000000000000000000 ) ) ;
#26285=ORIENTED_EDGE ( 'NONE', *, *, #33211, .T. ) ;
#26288=EDGE_CURVE ( 'NONE', #36981, #21371, #32760, .T. ) ;
#26289=TOROIDAL_SURFACE ( 'NONE', #11363, 1.000000000000000000, 0.5000000000000000000 ) ;
#26296=CARTESIAN_POINT ( 'NONE',  ( 14.72980548178180804, 19.66324911046165269, 7.102474990965864876 ) ) ;
#26297=VECTOR ( 'NONE', #4769, 1000.000000000000227 ) ;
#26298=VECTOR ( 'NONE', #3641, 1000.000000000000000 ) ;
#26299=CARTESIAN_POINT ( 'NONE',  ( 12.30736835487432579, 14.81698729810772619, 7.000000000000000000 ) ) ;
#26300=B_SPLINE_CURVE_WITH_KNOTS ( 'NONE', 3,
 ( #3270, #9373, #15663, #28050, #34751, #10169, #37791, #34356 ),
 .UNSPECIFIED., .F., .F.,
 ( 4, 2, 2, 4 ),
 ( 0.000000000000000000, 0.0002364868538934295958, 0.0004729737077868591917, 0.0009459474155737161065 ),
 .UNSPECIFIED. ) ;
#26303=FACE_OUTER_BOUND ( 'NONE', #26463, .T. ) ;
#26304=ADVANCED_FACE ( 'NONE', ( #16510 ), #25636, .T. ) ;
#26305=DIRECTION ( 'NONE',  ( -1.000000000000000000, 0.000000000000000000, 0.000000000000000000 ) ) ;
#26306=VERTEX_POINT ( 'NONE', #7150 ) ;
#26308=PLANE ( 'NONE',  #32420 ) ;
#26310=DIRECTION ( 'NONE',  ( 1.000000000000000000, 0.000000000000000000, 0.000000000000000000 ) ) ;
#26318=CARTESIAN_POINT ( 'NONE',  ( 10.44103466624280685, 32.57396620494213124, 9.000000000000001776 ) ) ;
#26322=ORIENTED_EDGE ( 'NONE', *, *, #5012, .T. ) ;
#26324=CARTESIAN_POINT ( 'NONE',  ( 14.41595319144214926, 26.31931657363112720, 10.49999999999999822 ) ) ;
#26327=CIRCLE ( 'NONE', #39317, 0.5000000000000004441 ) ;
#26336=DIRECTION ( 'NONE',  ( -0.8090169943749426773, 0.5877852522924796874, 0.000000000000000000 ) ) ;
#26340=ORIENTED_EDGE ( 'NONE', *, *, #24410, .T. ) ;
#26342=DIRECTION ( 'NONE',  ( -1.000000000000000000, 0.000000000000000000, 0.000000000000000000 ) ) ;
#26343=EDGE_CURVE ( 'NONE', #5601, #1586, #26042, .T. ) ;
#26344=( LENGTH_UNIT ( ) NAMED_UNIT ( * ) SI_UNIT ( .MILLI., .METRE. ) );
#26348=CYLINDRICAL_SURFACE ( 'NONE', #21686, 0.4999999999999984457 ) ;
#26349=DIRECTION ( 'NONE',  ( 1.000000000000000000, 0.000000000000000000, 0.000000000000000000 ) ) ;
#26354=CARTESIAN_POINT ( 'NONE',  ( -1.590043107810763079, 12.61456814725308107, 10.00000000000000000 ) ) ;
#26358=DIRECTION ( 'NONE',  ( -1.000000000000000000, 0.000000000000000000, 0.000000000000000000 ) ) ;
#26359=LINE ( 'NONE', #4422, #38526 ) ;
#26361=LINE ( 'NONE', #8072, #18559 ) ;
#26362=VERTEX_POINT ( 'NONE', #35602 ) ;
#26378=VERTEX_POINT ( 'NONE', #35398 ) ;
#26379=FACE_OUTER_BOUND ( 'NONE', #24541, .T. ) ;
#26381=CYLINDRICAL_SURFACE ( 'NONE', #27787, 0.4999999999999995559 ) ;
#26382=ADVANCED_FACE ( 'NONE', ( #17123 ), #10614, .T. ) ;
#26383=CARTESIAN_POINT ( 'NONE',  ( -8.412270287199726582, 10.07085245822961994, 10.49999999999999822 ) ) ;
#26384=ORIENTED_EDGE ( 'NONE', *, *, #2043, .T. ) ;
#26389=ORIENTED_EDGE ( 'NONE', *, *, #40163, .F. ) ;
#26393=EDGE_CURVE ( 'NONE', #19420, #2652, #38844, .T. ) ;
#26394=CARTESIAN_POINT ( 'NONE',  ( 9.831584923911636409, 26.22020669908449975, 10.50000000000000000 ) ) ;
#26395=CARTESIAN_POINT ( 'NONE',  ( -3.789799368034432181, 7.986433676831034667, 7.485699520496976511 ) ) ;
#26397=CYLINDRICAL_SURFACE ( 'NONE', #12298, 0.5000000000000000000 ) ;
#26398=ORIENTED_EDGE ( 'NONE', *, *, #14701, .T. ) ;
#26399=CARTESIAN_POINT ( 'NONE',  ( -14.31603901957233660, 19.98981538725089990, 10.49999999999999467 ) ) ;
#26405=CIRCLE ( 'NONE', #23194, 0.4999999999999998890 ) ;
#26406=VERTEX_POINT ( 'NONE', #22995 ) ;
#26407=DIRECTION ( 'NONE',  ( 0.000000000000000000, 0.000000000000000000, 1.000000000000000000 ) ) ;
#26408=CARTESIAN_POINT ( 'NONE',  ( 0.000000000000000000, 22.50000000000000355, 7.000000000000000000 ) ) ;
#26409=ADVANCED_FACE ( 'NONE', ( #32148 ), #4106, .T. ) ;
#26410=EDGE_CURVE ( 'NONE', #37009, #16315, #20718, .T. ) ;
#26414=DIRECTION ( 'NONE',  ( 0.4156269377774587936, 0.5720614028176801424, -0.7071067811865477948 ) ) ;
#26415=ORIENTED_EDGE ( 'NONE', *, *, #25025, .F. ) ;
#26416=CIRCLE ( 'NONE', #23167, 1.000000000000014655 ) ;
#26420=CARTESIAN_POINT ( 'NONE',  ( 1.838889047819958655, 31.15129278236397781, 9.000000000000001776 ) ) ;
#26424=LINE ( 'NONE', #27032, #8125 ) ;
#26430=CARTESIAN_POINT ( 'NONE',  ( -10.14084140100247389, 32.97648733965221624, 10.49999999999999822 ) ) ;
#26431=FACE_OUTER_BOUND ( 'NONE', #9603, .T. ) ;
#26432=FACE_OUTER_BOUND ( 'NONE', #11489, .T. ) ;
#26433=ORIENTED_EDGE ( 'NONE', *, *, #593, .F. ) ;
#26435=EDGE_CURVE ( 'NONE', #21143, #35248, #3815, .T. ) ;
#26436=LINE ( 'NONE', #38834, #7957 ) ;
#26440=ORIENTED_EDGE ( 'NONE', *, *, #16400, .T. ) ;
#26444=B_SPLINE_CURVE_WITH_KNOTS ( 'NONE', 3,
 ( #31197, #27552, #9266, #18416 ),
 .UNSPECIFIED., .F., .F.,
 ( 4, 4 ),
 ( 0.000000000000000000, 1.000000000000000000 ),
 .UNSPECIFIED. ) ;
#26445=FACE_OUTER_BOUND ( 'NONE', #36643, .T. ) ;
#26449=ORIENTED_EDGE ( 'NONE', *, *, #27220, .F. ) ;
#26452=CARTESIAN_POINT ( 'NONE',  ( -1.278175571584109660, 14.08178954835378427, 9.000000000000001776 ) ) ;
#26454=ADVANCED_FACE ( 'NONE', ( #13859 ), #34306, .T. ) ;
#26457=VECTOR ( 'NONE', #26414, 1000.000000000000000 ) ;
#26458=CARTESIAN_POINT ( 'NONE',  ( -11.11016527260153808, 31.83082137946488643, 7.500000000000004441 ) ) ;
#26460=ORIENTED_EDGE ( 'NONE', *, *, #35662, .F. ) ;
#26462=CIRCLE ( 'NONE', #4398, 0.5000000000000004441 ) ;
#26463=EDGE_LOOP ( 'NONE', ( #15079, #21625, #713, #2017 ) ) ;
#26465=AXIS2_PLACEMENT_3D ( 'NONE', #11104, #30595, #20652 ) ;
#26467=DIRECTION ( 'NONE',  ( 0.8660254037844431485, 0.4999999999999921174, -0.000000000000000000 ) ) ;
#26469=ORIENTED_EDGE ( 'NONE', *, *, #13596, .F. ) ;
#26472=EDGE_LOOP ( 'NONE', ( #36739, #23902, #18596, #1155 ) ) ;
#26473=CONICAL_SURFACE ( 'NONE', #5707, 0.5000000000000002220, 0.7853981633974506105 ) ;
#26475=DIRECTION ( 'NONE',  ( 0.000000000000000000, 0.000000000000000000, -1.000000000000000000 ) ) ;
#26477=CARTESIAN_POINT ( 'NONE',  ( 13.44717671261699010, 15.85337785810300026, 7.339470489435489853 ) ) ;
#26479=B_SPLINE_CURVE_WITH_KNOTS ( 'NONE', 3,
 ( #27300, #39878, #8817, #17776, #15303, #39688, #18556, #24646 ),
 .UNSPECIFIED., .F., .F.,
 ( 4, 2, 2, 4 ),
 ( 0.000000000000000000, 0.0002364868538934288640, 0.0004729737077868577280, 0.0009459474155737242380 ),
 .UNSPECIFIED. ) ;
#26480=ORIENTED_EDGE ( 'NONE', *, *, #9427, .F. ) ;
#26483=DIRECTION ( 'NONE',  ( -0.6459741880212607201, -0.2876062384759439094, -0.7071067811865414665 ) ) ;
#26487=CARTESIAN_POINT ( 'NONE',  ( -8.145563986382438060, 10.43794218875019908, 10.99999999999999289 ) ) ;
#26489=VERTEX_POINT ( 'NONE', #29500 ) ;
#26491=ADVANCED_FACE ( 'NONE', ( #29301 ), #1470, .T. ) ;
#26499=AXIS2_PLACEMENT_3D ( 'NONE', #39335, #5007, #29192 ) ;
#26501=EDGE_CURVE ( 'NONE', #11836, #29721, #31648, .T. ) ;
#26504=VECTOR ( 'NONE', #14357, 1000.000000000000000 ) ;
#26506=CARTESIAN_POINT ( 'NONE',  ( -13.94482798346716201, 26.50521816028930999, 9.500000000000000000 ) ) ;
#26507=LINE ( 'NONE', #16968, #30219 ) ;
#26510=CARTESIAN_POINT ( 'NONE',  ( -8.927394655428429360, 11.06314620770957013, 7.000000000000000000 ) ) ;
#26511=CARTESIAN_POINT ( 'NONE',  ( -14.57486473880221745, 26.18419839932921533, 7.000000000000000000 ) ) ;
#26515=CARTESIAN_POINT ( 'NONE',  ( 3.295881626406574672, 9.398963235502481695, 10.50000000000000000 ) ) ;
#26524=DIRECTION ( 'NONE',  ( -1.000000000000000000, 0.000000000000000000, 0.000000000000000000 ) ) ;
#26527=CARTESIAN_POINT ( 'NONE',  ( -14.51883047965001694, 21.47676356526632446, 11.00000000000000355 ) ) ;
#26530=LINE ( 'NONE', #23478, #32861 ) ;
#26537=ORIENTED_EDGE ( 'NONE', *, *, #39419, .F. ) ;
#26540=DIRECTION ( 'NONE',  ( 1.000000000000000000, 0.000000000000000000, 0.000000000000000000 ) ) ;
#26541=LINE ( 'NONE', #38930, #30350 ) ;
#26542=VECTOR ( 'NONE', #15907, 1000.000000000000114 ) ;
#26543=EDGE_LOOP ( 'NONE', ( #33157, #7281, #34501, #18112 ) ) ;
#26551=PLANE ( 'NONE',  #20321 ) ;
#26554=ORIENTED_EDGE ( 'NONE', *, *, #29593, .F. ) ;
#26555=CARTESIAN_POINT ( 'NONE',  ( -12.80736835487442349, 15.68301270189233954, 7.000000000000000000 ) ) ;
#26558=FACE_OUTER_BOUND ( 'NONE', #20481, .T. ) ;
#26559=ORIENTED_EDGE ( 'NONE', *, *, #8513, .F. ) ;
#26561=DIRECTION ( 'NONE',  ( 0.6691306063588671194, 0.7431448254773862505, 0.000000000000000000 ) ) ;
#26562=PLANE ( 'NONE',  #12362 ) ;
#26563=DIRECTION ( 'NONE',  ( -0.000000000000000000, -0.000000000000000000, -1.000000000000000000 ) ) ;
#26564=CARTESIAN_POINT ( 'NONE',  ( -6.686869517299739663, 14.99761530854305391, 10.50000000000000533 ) ) ;
#26565=CARTESIAN_POINT ( 'NONE',  ( -1.734965421685230824, 7.600674680189156263, 7.000000000000000000 ) ) ;
#26567=DIRECTION ( 'NONE',  ( -0.5254827454987587299, -0.4731467892558131605, -0.7071067811865487940 ) ) ;
#26568=ORIENTED_EDGE ( 'NONE', *, *, #10502, .T. ) ;
#26570=DIRECTION ( 'NONE',  ( 0.4067366430758009299, 0.9135454576426005335, -0.000000000000000000 ) ) ;
#26573=DIRECTION ( 'NONE',  ( 0.6691306063588570163, -0.7431448254773953543, 0.000000000000000000 ) ) ;
#26581=CARTESIAN_POINT ( 'NONE',  ( -12.30736835487442704, 14.81698729810789672, 7.499999999999993783 ) ) ;
#26585=CONICAL_SURFACE ( 'NONE', #31109, 0.5000000000000111022, 0.7853981633974492782 ) ;
#26586=DIRECTION ( 'NONE',  ( 0.000000000000000000, -0.000000000000000000, -1.000000000000000000 ) ) ;
#26588=CARTESIAN_POINT ( 'NONE',  ( -5.034171952701850472, 35.03623199971308111, 10.00000000000000000 ) ) ;
#26590=CIRCLE ( 'NONE', #9074, 0.4999999999999998335 ) ;
#26591=ORIENTED_EDGE ( 'NONE', *, *, #32902, .T. ) ;
#26593=ORIENTED_EDGE ( 'NONE', *, *, #35561, .F. ) ;
#26595=ORIENTED_EDGE ( 'NONE', *, *, #37296, .F. ) ;
#26596=LINE ( 'NONE', #2028, #7652 ) ;
#26597=VERTEX_POINT ( 'NONE', #14454 ) ;
#26601=CARTESIAN_POINT ( 'NONE',  ( 0.000000000000000000, 22.50000000000000355, 7.000000000000000000 ) ) ;
#26602=ORIENTED_EDGE ( 'NONE', *, *, #31759, .T. ) ;
#26605=CARTESIAN_POINT ( 'NONE',  ( 10.39021566973303656, 20.90519018800546647, 10.00000000000000000 ) ) ;
#26608=ORIENTED_EDGE ( 'NONE', *, *, #12218, .F. ) ;
#26609=FACE_OUTER_BOUND ( 'NONE', #5263, .T. ) ;
#26610=DIRECTION ( 'NONE',  ( -0.9135454576426070838, -0.4067366430757864970, 0.000000000000000000 ) ) ;
#26611=EDGE_CURVE ( 'NONE', #30937, #22876, #12261, .T. ) ;
#26613=CARTESIAN_POINT ( 'NONE',  ( 14.36830325120613594, 20.48707633493483371, 7.500000000000010658 ) ) ;
#26615=CARTESIAN_POINT ( 'NONE',  ( 13.48130249190479724, 27.93180293473185927, 9.500000000000000000 ) ) ;
#26619=EDGE_CURVE ( 'NONE', #4691, #16943, #34973, .T. ) ;
#26620=DIRECTION ( 'NONE',  ( -0.3090169943749434545, 0.9510565162951548634, 0.000000000000000000 ) ) ;
#26621=EDGE_CURVE ( 'NONE', #7162, #34341, #27056, .T. ) ;
#26622=ORIENTED_EDGE ( 'NONE', *, *, #23307, .F. ) ;
#26623=ORIENTED_EDGE ( 'NONE', *, *, #22264, .T. ) ;
#26625=DIRECTION ( 'NONE',  ( -0.000000000000000000, -0.000000000000000000, 1.000000000000000000 ) ) ;
#26626=DIRECTION ( 'NONE',  ( 0.8090169943749430104, -0.5877852522924791323, 0.000000000000000000 ) ) ;
#26627=VECTOR ( 'NONE', #2917, 999.9999999999998863 ) ;
#26633=PLANE ( 'NONE',  #14200 ) ;
#26634=CARTESIAN_POINT ( 'NONE',  ( -2.535262076962894184, 8.167662524930003443, 10.99999999999999289 ) ) ;
#26636=B_SPLINE_CURVE_WITH_KNOTS ( 'NONE', 3,
 ( #23654, #8418, #8211, #17777, #20616, #1725, #26296, #20414 ),
 .UNSPECIFIED., .F., .F.,
 ( 4, 2, 2, 4 ),
 ( 0.000000000000000000, 0.0002364868538934280237, 0.0004729737077868560475, 0.0009459474155737213107 ),
 .UNSPECIFIED. ) ;
#26637=ORIENTED_EDGE ( 'NONE', *, *, #691, .T. ) ;
#26639=CYLINDRICAL_SURFACE ( 'NONE', #11857, 0.5000000000000004441 ) ;
#26640=VERTEX_POINT ( 'NONE', #30102 ) ;
#26643=ORIENTED_EDGE ( 'NONE', *, *, #33127, .F. ) ;
#26645=ADVANCED_FACE ( 'NONE', ( #26649 ), #39038, .T. ) ;
#26647=DIRECTION ( 'NONE',  ( -0.8090169943749505599, -0.5877852522924690293, 0.000000000000000000 ) ) ;
#26649=FACE_OUTER_BOUND ( 'NONE', #21728, .T. ) ;
#26650=ORIENTED_EDGE ( 'NONE', *, *, #22999, .F. ) ;
#26652=DIRECTION ( 'NONE',  ( -0.000000000000000000, -0.000000000000000000, -1.000000000000000000 ) ) ;
#26654=AXIS2_PLACEMENT_3D ( 'NONE', #2278, #24005, #9169 ) ;
#26655=CARTESIAN_POINT ( 'NONE',  ( 2.140527761532491802, 7.619874298175139948, 10.49999999999999822 ) ) ;
#26662=EDGE_CURVE ( 'NONE', #6928, #26114, #11217, .T. ) ;
#26663=ORIENTED_EDGE ( 'NONE', *, *, #15825, .F. ) ;
#26665=ORIENTED_EDGE ( 'NONE', *, *, #34779, .T. ) ;
#26668=FACE_OUTER_BOUND ( 'NONE', #39261, .T. ) ;
#26673=VECTOR ( 'NONE', #177, 1000.000000000000000 ) ;
#26678=LINE ( 'NONE', #39066, #4313 ) ;
#26679=VERTEX_POINT ( 'NONE', #23803 ) ;
#26682=DIRECTION ( 'NONE',  ( 0.3090169943749448977, -0.9510565162951543083, 0.000000000000000000 ) ) ;
#26684=ORIENTED_EDGE ( 'NONE', *, *, #30468, .F. ) ;
#26686=CARTESIAN_POINT ( 'NONE',  ( -8.016213763118818392, 9.982035245863954742, 10.49999999999999822 ) ) ;
#26693=AXIS2_PLACEMENT_3D ( 'NONE', #8560, #14451, #24196 ) ;
#26695=EDGE_LOOP ( 'NONE', ( #34469, #32327, #36586 ) ) ;
#26697=EDGE_CURVE ( 'NONE', #29281, #24654, #5314, .T. ) ;
#26699=FACE_OUTER_BOUND ( 'NONE', #1562, .T. ) ;
#26700=CARTESIAN_POINT ( 'NONE',  ( 13.63581098909226874, 27.45627467658428955, 7.000000000000000000 ) ) ;
#26701=VECTOR ( 'NONE', #18691, 1000.000000000000227 ) ;
#26703=DIRECTION ( 'NONE',  ( 1.000000000000000000, 0.000000000000000000, 0.000000000000000000 ) ) ;
#26704=FACE_OUTER_BOUND ( 'NONE', #13345, .T. ) ;
#26710=CYLINDRICAL_SURFACE ( 'NONE', #21624, 0.5000000000000004441 ) ;
#26711=CARTESIAN_POINT ( 'NONE',  ( 8.401171878996485987, 21.11424711454080594, 9.000000000000001776 ) ) ;
#26712=B_SPLINE_CURVE_WITH_KNOTS ( 'NONE', 3,
 ( #37820, #13231, #16289, #13638, #22775, #31728 ),
 .UNSPECIFIED., .F., .F.,
 ( 4, 2, 4 ),
 ( 0.000000000000000000, 0.4666667928354990558, 0.9333335856709981115 ),
 .UNSPECIFIED. ) ;
#26713=EDGE_CURVE ( 'NONE', #19050, #25293, #33615, .T. ) ;
#26717=CIRCLE ( 'NONE', #34439, 0.5000000000000007772 ) ;
#26722=ORIENTED_EDGE ( 'NONE', *, *, #18412, .T. ) ;
#26723=CARTESIAN_POINT ( 'NONE',  ( -14.97009266215794554, 21.42933399866948818, 10.49999999999999822 ) ) ;
#26724=ORIENTED_EDGE ( 'NONE', *, *, #3908, .T. ) ;
#26726=DIRECTION ( 'NONE',  ( -0.000000000000000000, 0.000000000000000000, 1.000000000000000000 ) ) ;
#26738=FACE_OUTER_BOUND ( 'NONE', #10479, .T. ) ;
#26739=ORIENTED_EDGE ( 'NONE', *, *, #15807, .F. ) ;
#26742=DIRECTION ( 'NONE',  ( -0.000000000000000000, -0.000000000000000000, 1.000000000000000000 ) ) ;
#26744=CARTESIAN_POINT ( 'NONE',  ( 9.625795778761983001, 10.95253033666821274, 7.000000000000000000 ) ) ;
#26750=DIRECTION ( 'NONE',  ( -0.1045284632676570929, -0.9945218953682730678, 0.000000000000000000 ) ) ;
#26751=ORIENTED_EDGE ( 'NONE', *, *, #18470, .T. ) ;
#26754=DIRECTION ( 'NONE',  ( 0.000000000000000000, 0.000000000000000000, 1.000000000000000000 ) ) ;
#26756=CARTESIAN_POINT ( 'NONE',  ( 6.811226782241714517, 35.33967249274190436, 11.00000000000000000 ) ) ;
#26757=DIRECTION ( 'NONE',  ( 0.8660254037844377084, -0.5000000000000019984, 0.000000000000000000 ) ) ;
#26759=CARTESIAN_POINT ( 'NONE',  ( 9.408554248005412290, 10.90613044664325670, 10.49999999999999822 ) ) ;
#26762=ORIENTED_EDGE ( 'NONE', *, *, #32867, .T. ) ;
#26764=CARTESIAN_POINT ( 'NONE',  ( 5.034171952702015673, 35.03623199971300295, 10.00000000000000000 ) ) ;
#26765=CYLINDRICAL_SURFACE ( 'NONE', #9485, 0.5000000000000004441 ) ;
#26768=DIRECTION ( 'NONE',  ( -0.000000000000000000, -0.000000000000000000, -1.000000000000000000 ) ) ;
#26770=CARTESIAN_POINT ( 'NONE',  ( -16.72075857324140102, 7.444561356925720297, 7.000000000000000000 ) ) ;
#26771=DIRECTION ( 'NONE',  ( 0.000000000000000000, 0.000000000000000000, -1.000000000000000000 ) ) ;
#26777=LINE ( 'NONE', #5845, #14082 ) ;
#26778=ORIENTED_EDGE ( 'NONE', *, *, #18987, .T. ) ;
#26780=ORIENTED_EDGE ( 'NONE', *, *, #27420, .T. ) ;
#26782=FACE_OUTER_BOUND ( 'NONE', #34443, .T. ) ;
#26784=CARTESIAN_POINT ( 'NONE',  ( -2.140527761532693418, 7.619874298175171035, 11.00000000000000000 ) ) ;
#26787=ORIENTED_EDGE ( 'NONE', *, *, #4667, .T. ) ;
#26789=EDGE_CURVE ( 'NONE', #6055, #9203, #15659, .T. ) ;
#26794=AXIS2_PLACEMENT_3D ( 'NONE', #13634, #19735, #22174 ) ;
#26795=ORIENTED_EDGE ( 'NONE', *, *, #33265, .T. ) ;
#26797=CARTESIAN_POINT ( 'NONE',  ( -0.5000000000000000000, 37.50000000000000711, 10.63089969389957190 ) ) ;
#26798=ORIENTED_EDGE ( 'NONE', *, *, #30238, .F. ) ;
#26799=DIRECTION ( 'NONE',  ( 0.000000000000000000, 0.000000000000000000, -1.000000000000000000 ) ) ;
#26800=CARTESIAN_POINT ( 'NONE',  ( 6.506711629694180488, 35.47525137376717908, 10.83333333333333037 ) ) ;
#26801=CIRCLE ( 'NONE', #8657, 6.000000000000003553 ) ;
#26802=CARTESIAN_POINT ( 'NONE',  ( 4.727507481117211086, 31.88885898370940453, 10.50000000000000000 ) ) ;
#26805=PLANE ( 'NONE',  #20226 ) ;
#26806=VECTOR ( 'NONE', #15154, 1000.000000000000000 ) ;
#26807=CARTESIAN_POINT ( 'NONE',  ( -1.590043107810761525, 12.61456814725308817, 10.50000000000001066 ) ) ;
#26808=ADVANCED_FACE ( 'NONE', ( #21745 ), #39548, .T. ) ;
#26810=VECTOR ( 'NONE', #14356, 1000.000000000000000 ) ;
#26812=VERTEX_POINT ( 'NONE', #37599 ) ;
#26813=CARTESIAN_POINT ( 'NONE',  ( 12.68475447279711688, 27.14725768220934299, 9.500000000000000000 ) ) ;
#26815=ADVANCED_FACE ( 'NONE', ( #13001 ), #9765, .T. ) ;
#26817=DIRECTION ( 'NONE',  ( 0.5877852522924689183, -0.8090169943749505599, -0.000000000000000000 ) ) ;
#26820=VECTOR ( 'NONE', #23665, 1000.000000000000114 ) ;
#26823=CARTESIAN_POINT ( 'NONE',  ( 14.11133924723984379, 27.61078317377175750, 10.49999999999999822 ) ) ;
#26827=LINE ( 'NONE', #39217, #34093 ) ;
#26829=CARTESIAN_POINT ( 'NONE',  ( -2.317734025672947951, 9.191051544684766483, 7.000000000000000000 ) ) ;
#26830=DIRECTION ( 'NONE',  ( 1.000000000000000000, 0.000000000000000000, 0.000000000000000000 ) ) ;
#26831=EDGE_LOOP ( 'NONE', ( #31657, #39263, #15259, #38232 ) ) ;
#26833=LINE ( 'NONE', #17710, #8329 ) ;
#26834=DIRECTION ( 'NONE',  ( 0.5720614028176875809, -0.4156269377774574059, 0.7071067811865425767 ) ) ;
#26836=VERTEX_POINT ( 'NONE', #25389 ) ;
#26838=CARTESIAN_POINT ( 'NONE',  ( -13.63581098909220479, 27.45627467658446008, 7.499999999999993783 ) ) ;
#26844=( GEOMETRIC_REPRESENTATION_CONTEXT ( 3 ) GLOBAL_UNCERTAINTY_ASSIGNED_CONTEXT ( ( #38426 ) ) GLOBAL_UNIT_ASSIGNED_CONTEXT ( ( #7912, #38392, #7300 ) ) REPRESENTATION_CONTEXT ( 'NONE', 'WORKASPACE' ) );
#26846=EDGE_CURVE ( 'NONE', #22349, #3843, #15458, .T. ) ;
#26848=DIRECTION ( 'NONE',  ( -0.6916548014802257338, 0.1470157664652036178, -0.7071067811865463515 ) ) ;
#26850=AXIS2_PLACEMENT_3D ( 'NONE', #31444, #763, #12354 ) ;
#26851=CARTESIAN_POINT ( 'NONE',  ( 10.10646936306337729, 32.94553861768082470, 7.000000000000000000 ) ) ;
#26854=CARTESIAN_POINT ( 'NONE',  ( 14.52509594610761923, 21.97885917798724975, 10.49999999999999822 ) ) ;
#26856=CARTESIAN_POINT ( 'NONE',  ( 7.468455364333220992, 29.89744377950669474, 10.00000000000000000 ) ) ;
#26860=CARTESIAN_POINT ( 'NONE',  ( 13.48130249190479368, 27.93180293473185927, 11.00000000000000000 ) ) ;
#26861=CARTESIAN_POINT ( 'NONE',  ( -13.23567246089835869, 15.94827353674837767, 10.49999999999999822 ) ) ;
#26862=CARTESIAN_POINT ( 'NONE',  ( 2.535262076962677913, 8.167662524929967915, 11.00000000000000355 ) ) ;
#26869=EDGE_CURVE ( 'NONE', #29611, #25142, #24892, .T. ) ;
#26870=CARTESIAN_POINT ( 'NONE',  ( -14.31632963181202456, 26.62592636301959814, 10.82238861112336714 ) ) ;
#26874=ORIENTED_EDGE ( 'NONE', *, *, #17749, .T. ) ;
#26876=CARTESIAN_POINT ( 'NONE',  ( -5.440908595777636414, 35.94977745735568675, 11.00000000000000000 ) ) ;
#26878=CARTESIAN_POINT ( 'NONE',  ( -7.713869163866016621, 10.18146832927085121, 7.000000000000000000 ) ) ;
#26883=CARTESIAN_POINT ( 'NONE',  ( 13.95683075005237050, 28.08631143191933432, 7.000000000000000000 ) ) ;
#26884=ORIENTED_EDGE ( 'NONE', *, *, #8164, .F. ) ;
#26886=CARTESIAN_POINT ( 'NONE',  ( -7.899339922805356018, 10.02167583667232265, 10.49999999999999822 ) ) ;
#26887=FACE_OUTER_BOUND ( 'NONE', #28261, .T. ) ;
#26891=AXIS2_PLACEMENT_3D ( 'NONE', #33568, #25349, #28399 ) ;
#26894=ORIENTED_EDGE ( 'NONE', *, *, #14361, .F. ) ;
#26896=DIRECTION ( 'NONE',  ( 1.000000000000000000, 0.000000000000000000, -0.000000000000000000 ) ) ;
#26898=CARTESIAN_POINT ( 'NONE',  ( -8.843266739736659332, 16.81698729810787185, 10.00000000000000000 ) ) ;
#26901=EDGE_CURVE ( 'NONE', #25736, #23174, #30704, .T. ) ;
#26902=VECTOR ( 'NONE', #27167, 1000.000000000000114 ) ;
#26906=PLANE ( 'NONE',  #17267 ) ;
#26907=ORIENTED_EDGE ( 'NONE', *, *, #710, .T. ) ;
#26910=DIRECTION ( 'NONE',  ( 0.9135454576426005335, -0.4067366430758009299, 0.000000000000000000 ) ) ;
#26912=DIRECTION ( 'NONE',  ( 0.000000000000000000, 0.000000000000000000, 1.000000000000000000 ) ) ;
#26913=CARTESIAN_POINT ( 'NONE',  ( -14.72308455763294077, 20.12562289931506854, 10.49999999999999822 ) ) ;
#26916=ORIENTED_EDGE ( 'NONE', *, *, #19201, .T. ) ;
#26918=EDGE_CURVE ( 'NONE', #28310, #27267, #4491, .T. ) ;
#26920=ADVANCED_FACE ( 'NONE', ( #21950 ), #6500, .F. ) ;
#26921=EDGE_CURVE ( 'NONE', #13267, #36570, #18512, .T. ) ;
#26922=CARTESIAN_POINT ( 'NONE',  ( -11.44473057578096764, 31.45924896672619298, 10.49999999999999822 ) ) ;
#26924=VERTEX_POINT ( 'NONE', #1225 ) ;
#26926=ORIENTED_EDGE ( 'NONE', *, *, #19695, .F. ) ;
#26928=CARTESIAN_POINT ( 'NONE',  ( 9.941034666242805073, 32.57396620494213124, 9.500000000000000000 ) ) ;
#26934=CARTESIAN_POINT ( 'NONE',  ( 9.831584923911636409, 26.22020669908449975, 10.50000000000000000 ) ) ;
#26941=CIRCLE ( 'NONE', #9417, 15.00000000000000000 ) ;
#26945=VECTOR ( 'NONE', #8447, 1000.000000000000000 ) ;
#26946=DIRECTION ( 'NONE',  ( -0.3090169943749448977, 0.9510565162951543083, 0.000000000000000000 ) ) ;
#26948=DIRECTION ( 'NONE',  ( 0.5877852522924689183, -0.8090169943749503378, 0.000000000000000000 ) ) ;
#26949=ADVANCED_FACE ( 'NONE', ( #13197 ), #35550, .F. ) ;
#26952=ORIENTED_EDGE ( 'NONE', *, *, #2825, .T. ) ;
#26953=DIRECTION ( 'NONE',  ( -0.000000000000000000, 0.000000000000000000, 1.000000000000000000 ) ) ;
#26954=AXIS2_PLACEMENT_3D ( 'NONE', #10793, #23982, #36378 ) ;
#26955=DIRECTION ( 'NONE',  ( 1.000000000000000000, 0.000000000000000000, 0.000000000000000000 ) ) ;
#26956=ORIENTED_EDGE ( 'NONE', *, *, #29002, .F. ) ;
#26958=DIRECTION ( 'NONE',  ( 0.9659258262890684232, 0.2588190451025203509, 0.000000000000000000 ) ) ;
#26960=PLANE ( 'NONE',  #12914 ) ;
#26961=CIRCLE ( 'NONE', #3583, 5.999999999999996447 ) ;
#26966=DIRECTION ( 'NONE',  ( 0.000000000000000000, 0.000000000000000000, 1.000000000000000000 ) ) ;
#26967=CIRCLE ( 'NONE', #32810, 0.9999999999999997780 ) ;
#26974=EDGE_CURVE ( 'NONE', #5248, #13411, #19514, .T. ) ;
#26977=FACE_OUTER_BOUND ( 'NONE', #11151, .T. ) ;
#26978=FACE_OUTER_BOUND ( 'NONE', #6932, .T. ) ;
#26986=ORIENTED_EDGE ( 'NONE', *, *, #32339, .F. ) ;
#26987=APPLICATION_CONTEXT ( 'automotive_design' ) ;
#26989=ORIENTED_EDGE ( 'NONE', *, *, #3945, .T. ) ;
#26991=CARTESIAN_POINT ( 'NONE',  ( 13.95683075005237050, 28.08631143191933432, 10.50000000000000000 ) ) ;
#26992=EDGE_LOOP ( 'NONE', ( #4460, #2012, #21783, #20382 ) ) ;
#26993=CIRCLE ( 'NONE', #1676, 0.5000000000000004441 ) ;
#26995=EDGE_CURVE ( 'NONE', #2021, #4297, #1022, .T. ) ;
#26997=AXIS2_PLACEMENT_3D ( 'NONE', #23515, #26567, #7868 ) ;
#26999=EDGE_CURVE ( 'NONE', #36571, #28556, #5162, .T. ) ;
#27001=EDGE_LOOP ( 'NONE', ( #25229, #10140, #1748, #9251, #16 ) ) ;
#27003=ORIENTED_EDGE ( 'NONE', *, *, #28726, .F. ) ;
#27004=DIRECTION ( 'NONE',  ( 0.5877852522924801315, 0.8090169943749424553, -0.000000000000000000 ) ) ;
#27006=ADVANCED_FACE ( 'NONE', ( #10164 ), #25991, .F. ) ;
#27008=EDGE_LOOP ( 'NONE', ( #27992, #9277, #9009, #37217 ) ) ;
#27010=CARTESIAN_POINT ( 'NONE',  ( 4.794796183863160977, 36.71301971979253409, 7.000000000000000000 ) ) ;
#27011=LINE ( 'NONE', #39198, #37054 ) ;
#27014=ORIENTED_EDGE ( 'NONE', *, *, #38286, .F. ) ;
#27016=DIRECTION ( 'NONE',  ( -0.5877852522924690293, 0.8090169943749504489, 0.000000000000000000 ) ) ;
#27019=DIRECTION ( 'NONE',  ( 1.000000000000000000, 0.000000000000000000, 0.000000000000000000 ) ) ;
#27020=EDGE_CURVE ( 'NONE', #31127, #15240, #6897, .T. ) ;
#27021=EDGE_CURVE ( 'NONE', #3978, #38096, #10997, .T. ) ;
#27022=DIRECTION ( 'NONE',  ( 0.9781476007338070211, 0.2079116908177534029, -0.000000000000000000 ) ) ;
#27023=EDGE_CURVE ( 'NONE', #9166, #3260, #35001, .T. ) ;
#27025=AXIS2_PLACEMENT_3D ( 'NONE', #30178, #36472, #2549 ) ;
#27027=VECTOR ( 'NONE', #29326, 1000.000000000000000 ) ;
#27028=CARTESIAN_POINT ( 'NONE',  ( 3.610593701936714695, 31.83882289796390097, 10.49999999999999645 ) ) ;
#27032=CARTESIAN_POINT ( 'NONE',  ( -5.767236651883567156, 13.71142893291686171, 10.00000000000000000 ) ) ;
#27033=CARTESIAN_POINT ( 'NONE',  ( -12.09742388243079070, 14.36084852659847400, 10.49999999999999822 ) ) ;
#27034=CARTESIAN_POINT ( 'NONE',  ( 5.440908595777815826, 35.94977745735560859, 9.500000000000000000 ) ) ;
#27037=LINE ( 'NONE', #39420, #28413 ) ;
#27042=CARTESIAN_POINT ( 'NONE',  ( 15.02235689379175732, 21.92659494635341844, 10.50000000000000355 ) ) ;
#27043=ADVANCED_FACE ( 'NONE', ( #35350 ), #26397, .T. ) ;
#27044=ORIENTED_EDGE ( 'NONE', *, *, #8412, .F. ) ;
#27047=EDGE_CURVE ( 'NONE', #3614, #29069, #4467, .T. ) ;
#27052=B_SPLINE_CURVE_WITH_KNOTS ( 'NONE', 3,
 ( #28419, #19080, #10138, #34126 ),
 .UNSPECIFIED., .F., .F.,
 ( 4, 4 ),
 ( 0.000000000000000000, 1.000000000000000000 ),
 .UNSPECIFIED. ) ;
#27056=LINE ( 'NONE', #26851, #9664 ) ;
#27057=EDGE_LOOP ( 'NONE', ( #27189, #36761, #6322, #8792 ) ) ;
#27058=DIRECTION ( 'NONE',  ( -0.7431448254773862505, 0.6691306063588672304, -0.000000000000000000 ) ) ;
#27059=LINE ( 'NONE', #30905, #20202 ) ;
#27061=CARTESIAN_POINT ( 'NONE',  ( -14.36830325120615903, 20.48707633493503621, 7.000000000000000000 ) ) ;
#27065=DIRECTION ( 'NONE',  ( 0.2079116908177532919, -0.9781476007338070211, -0.000000000000000000 ) ) ;
#27066=CARTESIAN_POINT ( 'NONE',  ( 2.564829916171746937, 8.028556778314797526, 10.96580508970283141 ) ) ;
#27069=EDGE_LOOP ( 'NONE', ( #24116, #11610, #21892 ) ) ;
#27072=CARTESIAN_POINT ( 'NONE',  ( -14.41595319144209775, 26.31931657363132260, 10.49999999999999822 ) ) ;
#27083=ORIENTED_EDGE ( 'NONE', *, *, #25415, .T. ) ;
#27087=VERTEX_POINT ( 'NONE', #19298 ) ;
#27089=DIRECTION ( 'NONE',  ( 0.4067366430758009299, 0.9135454576426005335, 0.000000000000000000 ) ) ;
#27090=CARTESIAN_POINT ( 'NONE',  ( -14.42035624161473883, 26.65972665747678860, 11.00000000000000000 ) ) ;
#27091=VECTOR ( 'NONE', #18212, 999.9999999999998863 ) ;
#27092=EDGE_LOOP ( 'NONE', ( #27400, #17152, #15181, #32898 ) ) ;
#27094=VERTEX_POINT ( 'NONE', #28645 ) ;
#27097=ORIENTED_EDGE ( 'NONE', *, *, #26018, .F. ) ;
#27099=CARTESIAN_POINT ( 'NONE',  ( -15.64741614794215252, 37.44040872933206288, 7.000000000000000000 ) ) ;
#27101=CARTESIAN_POINT ( 'NONE',  ( 0.9999999999999991118, 36.00000000000000711, 10.00000000000000000 ) ) ;
#27102=FACE_OUTER_BOUND ( 'NONE', #34546, .T. ) ;
#27110=LINE ( 'NONE', #15118, #12310 ) ;
#27116=TOROIDAL_SURFACE ( 'NONE', #21257, 1.000000000000000000, 0.5000000000000000000 ) ;
#27118=ORIENTED_EDGE ( 'NONE', *, *, #2867, .F. ) ;
#27121=ADVANCED_FACE ( 'NONE', ( #34746 ), #31696, .T. ) ;
#27124=ORIENTED_EDGE ( 'NONE', *, *, #17381, .T. ) ;
#27125=CARTESIAN_POINT ( 'NONE',  ( -14.56494338438164071, 21.47191690367856864, 10.99387789255782799 ) ) ;
#27126=VERTEX_POINT ( 'NONE', #19498 ) ;
#27128=CARTESIAN_POINT ( 'NONE',  ( 5.440908595777814050, 35.94977745735560859, 7.000000000000000000 ) ) ;
#27136=ORIENTED_EDGE ( 'NONE', *, *, #9432, .T. ) ;
#27138=DIRECTION ( 'NONE',  ( -0.000000000000000000, -0.000000000000000000, -1.000000000000000000 ) ) ;
#27139=DIRECTION ( 'NONE',  ( 1.000000000000000000, 0.000000000000000000, 0.000000000000000000 ) ) ;
#27141=CARTESIAN_POINT ( 'NONE',  ( 15.02235689379175732, 21.92659494635341844, 10.50000000000000000 ) ) ;
#27142=ORIENTED_EDGE ( 'NONE', *, *, #29777, .F. ) ;
#27144=VECTOR ( 'NONE', #9104, 1000.000000000000000 ) ;
#27146=CIRCLE ( 'NONE', #10936, 1.000000000000004441 ) ;
#27147=PLANE ( 'NONE',  #31284 ) ;
#27150=CARTESIAN_POINT ( 'NONE',  ( 8.339609403135803234, 11.87216320208440123, 10.00000000000000000 ) ) ;
#27153=ORIENTED_EDGE ( 'NONE', *, *, #21533, .T. ) ;
#27154=ADVANCED_FACE ( 'NONE', ( #29046 ), #1421, .T. ) ;
#27155=FACE_OUTER_BOUND ( 'NONE', #15058, .T. ) ;
#27157=ORIENTED_EDGE ( 'NONE', *, *, #16970, .T. ) ;
#27159=CARTESIAN_POINT ( 'NONE',  ( -14.31603901957233838, 19.98981538725089990, 11.00000000000000000 ) ) ;
#27161=FACE_OUTER_BOUND ( 'NONE', #24341, .T. ) ;
#27167=DIRECTION ( 'NONE',  ( 0.4731467892558273158, 0.5254827454987467394, -0.7071067811865482389 ) ) ;
#27169=ORIENTED_EDGE ( 'NONE', *, *, #31962, .T. ) ;
#27171=DIRECTION ( 'NONE',  ( 1.000000000000000000, 0.000000000000000000, 0.000000000000000000 ) ) ;
#27172=CARTESIAN_POINT ( 'NONE',  ( 0.000000000000000000, 22.50000000000000355, 7.000000000000000000 ) ) ;
#27174=DIRECTION ( 'NONE',  ( -0.000000000000000000, -0.000000000000000000, -1.000000000000000000 ) ) ;
#27176=AXIS2_PLACEMENT_3D ( 'NONE', #17525, #8766, #12010 ) ;
#27178=FACE_OUTER_BOUND ( 'NONE', #37429, .T. ) ;
#27179=EDGE_CURVE ( 'NONE', #9314, #7162, #23559, .T. ) ;
#27180=DIRECTION ( 'NONE',  ( -1.224646799147351235E-16, 1.000000000000000000, 0.000000000000000000 ) ) ;
#27187=ORIENTED_EDGE ( 'NONE', *, *, #25093, .F. ) ;
#27189=ORIENTED_EDGE ( 'NONE', *, *, #1972, .F. ) ;
#27190=CARTESIAN_POINT ( 'NONE',  ( 4.524139159579308789, 31.43208625488810171, 10.49999999999999645 ) ) ;
#27191=CARTESIAN_POINT ( 'NONE',  ( 9.204968164644647288, 10.68109904802224541, 10.68306085400111982 ) ) ;
#27194=VECTOR ( 'NONE', #4728, 1000.000000000000114 ) ;
#27195=AXIS2_PLACEMENT_3D ( 'NONE', #2774, #14571, #24110 ) ;
#27196=ORIENTED_EDGE ( 'NONE', *, *, #38570, .F. ) ;
#27197=EDGE_CURVE ( 'NONE', #26812, #16537, #38244, .T. ) ;
#27198=DIRECTION ( 'NONE',  ( 0.8660254037844363761, -0.5000000000000038858, 0.000000000000000000 ) ) ;
#27200=EDGE_CURVE ( 'NONE', #6928, #37263, #34364, .T. ) ;
#27201=AXIS2_PLACEMENT_3D ( 'NONE', #16260, #37991, #4056 ) ;
#27202=CYLINDRICAL_SURFACE ( 'NONE', #2212, 0.5000000000000004441 ) ;
#27203=DIRECTION ( 'NONE',  ( -1.000000000000000000, 0.000000000000000000, 0.000000000000000000 ) ) ;
#27204=CARTESIAN_POINT ( 'NONE',  ( 10.47804177580207607, 33.28010392086025604, 10.49999999999999645 ) ) ;
#27205=ORIENTED_EDGE ( 'NONE', *, *, #4478, .F. ) ;
#27206=LINE ( 'NONE', #18271, #33460 ) ;
#27207=CARTESIAN_POINT ( 'NONE',  ( 10.47804177580207607, 33.28010392086025604, 10.50000000000000000 ) ) ;
#27208=DIRECTION ( 'NONE',  ( -0.000000000000000000, -0.000000000000000000, -1.000000000000000000 ) ) ;
#27212=ORIENTED_EDGE ( 'NONE', *, *, #21507, .T. ) ;
#27217=B_SPLINE_CURVE_WITH_KNOTS ( 'NONE', 3,
 ( #28026, #15639, #30881, #15437 ),
 .UNSPECIFIED., .F., .F.,
 ( 4, 4 ),
 ( 0.000000000000000000, 1.000000000000000000 ),
 .UNSPECIFIED. ) ;
#27218=DIRECTION ( 'NONE',  ( 0.000000000000000000, 0.000000000000000000, 1.000000000000000000 ) ) ;
#27220=EDGE_CURVE ( 'NONE', #7663, #5398, #39193, .T. ) ;
#27225=ADVANCED_FACE ( 'NONE', ( #36547 ), #24151, .T. ) ;
#27226=DIRECTION ( 'NONE',  ( -0.9781476007338069101, -0.2079116908177533751, 0.000000000000000000 ) ) ;
#27227=ORIENTED_EDGE ( 'NONE', *, *, #32488, .T. ) ;
#27228=EDGE_LOOP ( 'NONE', ( #17598, #38593, #27711, #20307 ) ) ;
#27231=LINE ( 'NONE', #18099, #21110 ) ;
#27232=CARTESIAN_POINT ( 'NONE',  ( -5.237540274239744775, 35.49300472853438038, 7.500000000000000888 ) ) ;
#27233=VERTEX_POINT ( 'NONE', #4864 ) ;
#27235=DIRECTION ( 'NONE',  ( -0.000000000000000000, -0.000000000000000000, -1.000000000000000000 ) ) ;
#27236=CARTESIAN_POINT ( 'NONE',  ( 0.000000000000000000, 22.50000000000000355, 7.000000000000000000 ) ) ;
#27237=VERTEX_POINT ( 'NONE', #14412 ) ;
#27240=VERTEX_POINT ( 'NONE', #17277 ) ;
#27250=VECTOR ( 'NONE', #39205, 1000.000000000000114 ) ;
#27252=ORIENTED_EDGE ( 'NONE', *, *, #33333, .T. ) ;
#27254=CARTESIAN_POINT ( 'NONE',  ( 13.86830325120613594, 20.48707633493483371, 7.500000000000010658 ) ) ;
#27255=CIRCLE ( 'NONE', #24670, 15.00000000000000000 ) ;
#27257=DIRECTION ( 'NONE',  ( -0.000000000000000000, -0.000000000000000000, -1.000000000000000000 ) ) ;
#27261=B_SPLINE_CURVE_WITH_KNOTS ( 'NONE', 3,
 ( #34159, #31700, #6111, #37002, #21955, #822 ),
 .UNSPECIFIED., .F., .F.,
 ( 4, 2, 4 ),
 ( 0.000000000000000000, 0.5000000000000000000, 1.000000000000000000 ),
 .UNSPECIFIED. ) ;
#27262=CARTESIAN_POINT ( 'NONE',  ( -12.88757880222275887, 15.63670317852396074, 10.99387789255782266 ) ) ;
#27263=CARTESIAN_POINT ( 'NONE',  ( 10.10646936306337729, 32.94553861768082470, 10.49999999999999645 ) ) ;
#27267=VERTEX_POINT ( 'NONE', #8718 ) ;
#27269=AXIS2_PLACEMENT_3D ( 'NONE', #34946, #10763, #4861 ) ;
#27272=ADVANCED_FACE ( 'NONE', ( #18071 ), #11570, .T. ) ;
#27273=CARTESIAN_POINT ( 'NONE',  ( 4.003810537522394242, 8.420815593655317954, 10.49999999999999822 ) ) ;
#27277=ORIENTED_EDGE ( 'NONE', *, *, #33229, .T. ) ;
#27279=CARTESIAN_POINT ( 'NONE',  ( 7.741055489194820893, 10.14404956260389667, 10.49999999999999822 ) ) ;
#27283=EDGE_CURVE ( 'NONE', #25293, #27469, #32111, .T. ) ;
#27286=DIRECTION ( 'NONE',  ( 0.000000000000000000, 0.000000000000000000, 1.000000000000000000 ) ) ;
#27291=AXIS2_PLACEMENT_3D ( 'NONE', #1985, #20671, #33068 ) ;
#27292=ORIENTED_EDGE ( 'NONE', *, *, #3618, .T. ) ;
#27294=VERTEX_POINT ( 'NONE', #36151 ) ;
#27297=ORIENTED_EDGE ( 'NONE', *, *, #24492, .T. ) ;
#27299=EDGE_CURVE ( 'NONE', #21130, #8575, #21400, .T. ) ;
#27300=CARTESIAN_POINT ( 'NONE',  ( -10.72918489117944674, 32.98258515686310943, 7.500000000000004441 ) ) ;
#27301=EDGE_CURVE ( 'NONE', #28965, #25600, #7114, .T. ) ;
#27303=CARTESIAN_POINT ( 'NONE',  ( 0.000000000000000000, 0.000000000000000000, 7.000000000000000000 ) ) ;
#27306=DIRECTION ( 'NONE',  ( -0.8660254037844364872, 0.5000000000000038858, -0.000000000000000000 ) ) ;
#27312=FACE_OUTER_BOUND ( 'NONE', #14704, .T. ) ;
#27315=ORIENTED_EDGE ( 'NONE', *, *, #1203, .T. ) ;
#27318=EDGE_CURVE ( 'NONE', #28310, #37355, #17679, .T. ) ;
#27319=CYLINDRICAL_SURFACE ( 'NONE', #39312, 0.4999999999999995559 ) ;
#27321=EDGE_LOOP ( 'NONE', ( #2349, #23277, #36279, #35234, #31575 ) ) ;
#27322=DIRECTION ( 'NONE',  ( -0.8090169943749510040, -0.5877852522924683631, 0.000000000000000000 ) ) ;
#27323=EDGE_LOOP ( 'NONE', ( #3546, #25713, #30523 ) ) ;
#27327=CARTESIAN_POINT ( 'NONE',  ( -9.343266739736648674, 17.68301270189230578, 10.00000000000000000 ) ) ;
#27335=AXIS2_PLACEMENT_3D ( 'NONE', #8158, #39237, #20564 ) ;
#27337=DIRECTION ( 'NONE',  ( 1.000000000000000000, 0.000000000000000000, 0.000000000000000000 ) ) ;
#27338=DIRECTION ( 'NONE',  ( 1.000000000000000000, 0.000000000000000000, 0.000000000000000000 ) ) ;
#27339=EDGE_LOOP ( 'NONE', ( #26665, #23089, #22433, #26384 ) ) ;
#27342=DIRECTION ( 'NONE',  ( -1.000000000000000000, 0.000000000000000000, 0.000000000000000000 ) ) ;
#27345=DIRECTION ( 'NONE',  ( -0.6123724356957974679, 0.3535533905932733978, -0.7071067811865451302 ) ) ;
#27346=ORIENTED_EDGE ( 'NONE', *, *, #4387, .F. ) ;
#27348=DIRECTION ( 'NONE',  ( -0.9135454576426059736, -0.4067366430757888285, 0.000000000000000000 ) ) ;
#27349=AXIS2_PLACEMENT_3D ( 'NONE', #13807, #25800, #38197 ) ;
#27350=DIRECTION ( 'NONE',  ( -0.000000000000000000, -0.000000000000000000, -1.000000000000000000 ) ) ;
#27354=PLANE ( 'NONE',  #11370 ) ;
#27356=EDGE_CURVE ( 'NONE', #3290, #26362, #11026, .T. ) ;
#27357=DIRECTION ( 'NONE',  ( -0.000000000000000000, -0.000000000000000000, 1.000000000000000000 ) ) ;
#27360=LINE ( 'NONE', #18226, #21644 ) ;
#27362=CARTESIAN_POINT ( 'NONE',  ( 13.42604558747167864, 21.08886574588663620, 7.000000000000000000 ) ) ;
#27365=FACE_OUTER_BOUND ( 'NONE', #29688, .T. ) ;
#27366=CARTESIAN_POINT ( 'NONE',  ( -13.81505241748936541, 27.51451374705156638, 10.96580508970282253 ) ) ;
#27373=DIRECTION ( 'NONE',  ( 0.000000000000000000, 0.000000000000000000, 1.000000000000000000 ) ) ;
#27379=ADVANCED_FACE ( 'NONE', ( #37346 ), #9319, .T. ) ;
#27383=CARTESIAN_POINT ( 'NONE',  ( -20.33644687577595178, 12.50987689638972356, 7.499999999999997335 ) ) ;
#27384=VERTEX_POINT ( 'NONE', #6455 ) ;
#27385=DIRECTION ( 'NONE',  ( 0.9781476007338041345, -0.2079116908177664202, 0.000000000000000000 ) ) ;
#27386=CARTESIAN_POINT ( 'NONE',  ( -8.118377661053488126, 10.47536095541708967, 7.500000000000000888 ) ) ;
#27387=B_SPLINE_CURVE_WITH_KNOTS ( 'NONE', 3,
 ( #36608, #30915, #34363, #2680, #2879, #24613 ),
 .UNSPECIFIED., .F., .F.,
 ( 4, 2, 4 ),
 ( 0.000000000000000000, 0.5000000000000000000, 1.000000000000000000 ),
 .UNSPECIFIED. ) ;
#27390=ADVANCED_FACE ( 'NONE', ( #18268 ), #18817, .T. ) ;
#27392=AXIS2_PLACEMENT_3D ( 'NONE', #22930, #26179, #32495 ) ;
#27393=DIRECTION ( 'NONE',  ( 0.8090169943749503378, 0.5877852522924691403, 0.000000000000000000 ) ) ;
#27394=EDGE_LOOP ( 'NONE', ( #22815, #12146, #18713 ) ) ;
#27398=AXIS2_PLACEMENT_3D ( 'NONE', #14540, #8242, #17810 ) ;
#27399=DIRECTION ( 'NONE',  ( 0.5877852522924690293, -0.8090169943749503378, 0.000000000000000000 ) ) ;
#27400=ORIENTED_EDGE ( 'NONE', *, *, #4933, .F. ) ;
#27401=ADVANCED_FACE ( 'NONE', ( #21702 ), #5863, .T. ) ;
#27402=FACE_OUTER_BOUND ( 'NONE', #31208, .T. ) ;
#27403=CARTESIAN_POINT ( 'NONE',  ( -2.525645716490711123, 8.212903943950955465, 11.00000000000000000 ) ) ;
#27405=DIRECTION ( 'NONE',  ( -0.000000000000000000, -0.000000000000000000, -1.000000000000000000 ) ) ;
#27409=ORIENTED_EDGE ( 'NONE', *, *, #24947, .T. ) ;
#27411=CARTESIAN_POINT ( 'NONE',  ( 8.927394655428276593, 11.06314620770945290, 9.000000000000001776 ) ) ;
#27412=AXIS2_PLACEMENT_3D ( 'NONE', #28102, #21806, #12070 ) ;
#27415=CARTESIAN_POINT ( 'NONE',  ( 8.505700342264139735, 22.10876900990906435, 9.000000000000001776 ) ) ;
#27420=EDGE_CURVE ( 'NONE', #32326, #8749, #31055, .T. ) ;
#27424=EDGE_LOOP ( 'NONE', ( #38262, #35351, #652, #28991 ) ) ;
#27425=ORIENTED_EDGE ( 'NONE', *, *, #27775, .T. ) ;
#27427=CARTESIAN_POINT ( 'NONE',  ( 0.9658050764552033041, 37.18846563620834189, 10.49999999999999822 ) ) ;
#27429=VECTOR ( 'NONE', #26483, 1000.000000000000000 ) ;
#27430=CARTESIAN_POINT ( 'NONE',  ( -9.415016184005896349, 11.18446770392341350, 10.49999999999999822 ) ) ;
#27431=ORIENTED_EDGE ( 'NONE', *, *, #28641, .T. ) ;
#27434=CARTESIAN_POINT ( 'NONE',  ( 14.06524961900336734, 27.71236540882597410, 7.000000000000000000 ) ) ;
#27437=DIRECTION ( 'NONE',  ( -0.6691306063588576825, 0.7431448254773946882, 0.000000000000000000 ) ) ;
#27443=DIRECTION ( 'NONE',  ( -0.2079116908177533474, 0.9781476007338067991, -0.000000000000000000 ) ) ;
#27446=AXIS2_PLACEMENT_3D ( 'NONE', #33327, #2240, #14628 ) ;
#27448=ORIENTED_EDGE ( 'NONE', *, *, #38667, .T. ) ;
#27450=AXIS2_PLACEMENT_3D ( 'NONE', #28112, #18580, #40104 ) ;
#27453=VECTOR ( 'NONE', #4664, 999.9999999999998863 ) ;
#27457=CARTESIAN_POINT ( 'NONE',  ( -9.911438049898041669, 11.24107483890965575, 7.000000000000000000 ) ) ;
#27458=CARTESIAN_POINT ( 'NONE',  ( -6.354454053420248272, 35.54304081427989814, 7.000000000000000000 ) ) ;
#27459=CARTESIAN_POINT ( 'NONE',  ( 9.593266739736579396, 18.11602540378440196, 10.50000000000000178 ) ) ;
#27461=AXIS2_PLACEMENT_3D ( 'NONE', #8272, #5226, #39550 ) ;
#27462=ORIENTED_EDGE ( 'NONE', *, *, #17005, .T. ) ;
#27467=CARTESIAN_POINT ( 'NONE',  ( -14.06932099033139849, 26.54566839026276170, 11.00000000000000000 ) ) ;
#27469=VERTEX_POINT ( 'NONE', #16009 ) ;
#27471=CARTESIAN_POINT ( 'NONE',  ( 8.347978306607052090, 10.15934277794823437, 10.82238861112330497 ) ) ;
#27473=CARTESIAN_POINT ( 'NONE',  ( 1.693998953219503667, 12.12549434688615513, 10.00000000000000000 ) ) ;
#27476=ORIENTED_EDGE ( 'NONE', *, *, #28253, .T. ) ;
#27482=LINE ( 'NONE', #25231, #34277 ) ;
#27484=CARTESIAN_POINT ( 'NONE',  ( 10.49474413300068854, 21.89971208337374975, 11.00000000000000000 ) ) ;
#27485=EDGE_LOOP ( 'NONE', ( #6917, #24291, #16343, #2147 ) ) ;
#27487=ORIENTED_EDGE ( 'NONE', *, *, #22993, .T. ) ;
#27489=AXIS2_PLACEMENT_3D ( 'NONE', #9516, #15805, #167 ) ;
#27491=ORIENTED_EDGE ( 'NONE', *, *, #28654, .T. ) ;
#27493=PLANE ( 'NONE',  #22912 ) ;
#27495=CARTESIAN_POINT ( 'NONE',  ( -12.05736835487443415, 14.38397459621567442, 10.49999999999999822 ) ) ;
#27496=CIRCLE ( 'NONE', #15175, 15.00000000000000000 ) ;
#27498=EDGE_CURVE ( 'NONE', #16093, #27094, #24556, .T. ) ;
#27499=CYLINDRICAL_SURFACE ( 'NONE', #27936, 0.5000000000000004441 ) ;
#27501=EDGE_CURVE ( 'NONE', #12231, #18928, #25146, .T. ) ;
#27504=ORIENTED_EDGE ( 'NONE', *, *, #36174, .T. ) ;
#27512=ORIENTED_EDGE ( 'NONE', *, *, #20532, .T. ) ;
#27513=CIRCLE ( 'NONE', #29454, 6.000000000000003553 ) ;
#27516=DIRECTION ( 'NONE',  ( -0.000000000000000000, -0.000000000000000000, -1.000000000000000000 ) ) ;
#27519=CARTESIAN_POINT ( 'NONE',  ( -6.651296319737220131, 27.81603774131167839, 7.000000000000000000 ) ) ;
#27520=EDGE_CURVE ( 'NONE', #18869, #12427, #24645, .T. ) ;
#27521=ORIENTED_EDGE ( 'NONE', *, *, #12857, .F. ) ;
#27524=EDGE_CURVE ( 'NONE', #13055, #18790, #6648, .T. ) ;
#27526=CARTESIAN_POINT ( 'NONE',  ( 9.080802685385512163, 10.85199816882120416, 10.94611345180490680 ) ) ;
#27529=AXIS2_PLACEMENT_3D ( 'NONE', #13760, #13560, #38751 ) ;
#27531=LINE ( 'NONE', #9241, #15075 ) ;
#27533=ORIENTED_EDGE ( 'NONE', *, *, #17159, .T. ) ;
#27535=CARTESIAN_POINT ( 'NONE',  ( 13.63581098909227052, 27.45627467658428600, 9.500000000000000000 ) ) ;
#27537=DIRECTION ( 'NONE',  ( 1.000000000000000000, 0.000000000000000000, 0.000000000000000000 ) ) ;
#27538=VERTEX_POINT ( 'NONE', #2819 ) ;
#27545=EDGE_CURVE ( 'NONE', #38699, #10050, #27601, .T. ) ;
#27547=CIRCLE ( 'NONE', #2267, 0.5000000000000004441 ) ;
#27548=ADVANCED_FACE ( 'NONE', ( #36951 ), #21501, .T. ) ;
#27551=CARTESIAN_POINT ( 'NONE',  ( 2.620168631248871005, 12.57794293788735729, 10.74999999999999289 ) ) ;
#27552=CARTESIAN_POINT ( 'NONE',  ( 14.04783364825886238, 26.18819932152407404, 10.66666666666666607 ) ) ;
#27554=DIRECTION ( 'NONE',  ( 0.3090169943749573322, 0.9510565162951504226, -0.000000000000000000 ) ) ;
#27555=CARTESIAN_POINT ( 'NONE',  ( 5.982165713378432059, 28.55918256678898715, 9.000000000000001776 ) ) ;
#27556=CARTESIAN_POINT ( 'NONE',  ( -9.705584749708384251, 11.06314620770957013, 7.221809905720049549 ) ) ;
#27557=CARTESIAN_POINT ( 'NONE',  ( 11.48173768534036121, 32.16538668264416145, 7.000000000000000000 ) ) ;
#27558=CARTESIAN_POINT ( 'NONE',  ( -3.503793317224518145, 8.420815634768723967, 11.00000000000000000 ) ) ;
#27559=CARTESIAN_POINT ( 'NONE',  ( -5.537946624085890335, 36.44027069998196566, 7.500000000000000888 ) ) ;
#27560=AXIS2_PLACEMENT_3D ( 'NONE', #26613, #14423, #39207 ) ;
#27562=CARTESIAN_POINT ( 'NONE',  ( 11.94134295108989363, 16.18301270189217078, 7.000000000000000000 ) ) ;
#27563=ORIENTED_EDGE ( 'NONE', *, *, #25042, .T. ) ;
#27565=DIRECTION ( 'NONE',  ( -0.9135454576426059736, -0.4067366430757888285, 0.000000000000000000 ) ) ;
#27566=CARTESIAN_POINT ( 'NONE',  ( -13.67979938750370650, 27.47056737363399392, 10.99999999999999289 ) ) ;
#27571=EDGE_LOOP ( 'NONE', ( #7740, #20783, #28388, #3623 ) ) ;
#27572=CIRCLE ( 'NONE', #13288, 0.9999999999999992228 ) ;
#27573=DIRECTION ( 'NONE',  ( -1.000000000000000000, 0.000000000000000000, 0.000000000000000000 ) ) ;
#27574=CARTESIAN_POINT ( 'NONE',  ( -14.42035624161473883, 26.65972665747678860, 7.000000000000000000 ) ) ;
#27576=VECTOR ( 'NONE', #24750, 1000.000000000000000 ) ;
#27581=CARTESIAN_POINT ( 'NONE',  ( 14.47283171447379502, 21.48159823030311344, 7.000000000000000000 ) ) ;
#27584=ORIENTED_EDGE ( 'NONE', *, *, #7561, .F. ) ;
#27587=ORIENTED_EDGE ( 'NONE', *, *, #9790, .F. ) ;
#27589=LINE ( 'NONE', #27984, #5066 ) ;
#27592=AXIS2_PLACEMENT_3D ( 'NONE', #14381, #26768, #39158 ) ;
#27595=ORIENTED_EDGE ( 'NONE', *, *, #22762, .T. ) ;
#27596=LINE ( 'NONE', #33905, #36565 ) ;
#27597=VECTOR ( 'NONE', #9433, 1000.000000000000000 ) ;
#27598=CARTESIAN_POINT ( 'NONE',  ( 11.11016527260166420, 31.83082137946473367, 11.00000000000000000 ) ) ;
#27600=CIRCLE ( 'NONE', #1015, 0.4999999999999997780 ) ;
#27601=LINE ( 'NONE', #15213, #14911 ) ;
#27602=ORIENTED_EDGE ( 'NONE', *, *, #37481, .T. ) ;
#27604=DIRECTION ( 'NONE',  ( 0.8090169943749503378, 0.5877852522924690293, 0.000000000000000000 ) ) ;
#27605=PLANE ( 'NONE',  #23468 ) ;
#27609=ORIENTED_EDGE ( 'NONE', *, *, #38260, .F. ) ;
#27611=PLANE ( 'NONE',  #15307 ) ;
#27613=LINE ( 'NONE', #33731, #2254 ) ;
#27618=EDGE_CURVE ( 'NONE', #1914, #7168, #35295, .T. ) ;
#27619=DIRECTION ( 'NONE',  ( 0.000000000000000000, -0.000000000000000000, 1.000000000000000000 ) ) ;
#27620=EDGE_LOOP ( 'NONE', ( #13396, #10754, #32800 ) ) ;
#27621=ORIENTED_EDGE ( 'NONE', *, *, #26343, .F. ) ;
#27623=CONICAL_SURFACE ( 'NONE', #25675, 1.000000000000004441, 0.7853981633974526089 ) ;
#27625=CARTESIAN_POINT ( 'NONE',  ( 12.68475447279711510, 27.14725768220934299, 10.50000000000000000 ) ) ;
#27626=AXIS2_PLACEMENT_3D ( 'NONE', #6553, #3516, #474 ) ;
#27627=CONICAL_SURFACE ( 'NONE', #10110, 1.000000000000004441, 0.7853981633974548293 ) ;
#27628=DIRECTION ( 'NONE',  ( 0.000000000000000000, 0.000000000000000000, -1.000000000000000000 ) ) ;
#27629=ORIENTED_EDGE ( 'NONE', *, *, #2123, .F. ) ;
#27633=AXIS2_PLACEMENT_3D ( 'NONE', #28355, #10272, #18826 ) ;
#27634=CARTESIAN_POINT ( 'NONE',  ( -8.927394655428429360, 11.06314620770957013, 7.000000000000000000 ) ) ;
#27635=ADVANCED_FACE ( 'NONE', ( #37743 ), #7050, .T. ) ;
#27636=ORIENTED_EDGE ( 'NONE', *, *, #14923, .F. ) ;
#27639=ORIENTED_EDGE ( 'NONE', *, *, #31867, .T. ) ;
#27641=ORIENTED_EDGE ( 'NONE', *, *, #24248, .F. ) ;
#27648=CARTESIAN_POINT ( 'NONE',  ( 7.713869163865849643, 10.18146832927074996, 7.500000000000000888 ) ) ;
#27653=CARTESIAN_POINT ( 'NONE',  ( 6.651296319737277862, 27.81603774131160023, 7.000000000000000000 ) ) ;
#27655=CIRCLE ( 'NONE', #27025, 0.5000000000000000000 ) ;
#27657=CIRCLE ( 'NONE', #30197, 6.000000000000003553 ) ;
#27659=CARTESIAN_POINT ( 'NONE',  ( -3.992867117591420545, 8.524771480177605554, 9.500000000000000000 ) ) ;
#27661=DIRECTION ( 'NONE',  ( -0.000000000000000000, -0.000000000000000000, 1.000000000000000000 ) ) ;
#27662=ORIENTED_EDGE ( 'NONE', *, *, #13011, .T. ) ;
#27672=CARTESIAN_POINT ( 'NONE',  ( 13.58430815669644254, 27.61478409596681516, 10.83333333333333215 ) ) ;
#27673=ORIENTED_EDGE ( 'NONE', *, *, #22653, .T. ) ;
#27677=ORIENTED_EDGE ( 'NONE', *, *, #19305, .F. ) ;
#27679=FACE_OUTER_BOUND ( 'NONE', #35296, .T. ) ;
#27680=CARTESIAN_POINT ( 'NONE',  ( 6.354454053420411697, 35.54304081427980577, 7.000000000000000000 ) ) ;
#27683=ORIENTED_EDGE ( 'NONE', *, *, #162, .T. ) ;
#27690=PLANE ( 'NONE',  #219 ) ;
#27694=EDGE_CURVE ( 'NONE', #6928, #9314, #26590, .T. ) ;
#27695=CARTESIAN_POINT ( 'NONE',  ( -6.651296319737220131, 27.81603774131167839, 9.000000000000001776 ) ) ;
#27697=ORIENTED_EDGE ( 'NONE', *, *, #36311, .F. ) ;
#27700=DIRECTION ( 'NONE',  ( -0.000000000000000000, -0.000000000000000000, -1.000000000000000000 ) ) ;
#27705=VERTEX_POINT ( 'NONE', #6847 ) ;
#27707=AXIS2_PLACEMENT_3D ( 'NONE', #32689, #7480, #1803 ) ;
#27709=DIRECTION ( 'NONE',  ( -1.000000000000000000, 0.000000000000000000, 0.000000000000000000 ) ) ;
#27711=ORIENTED_EDGE ( 'NONE', *, *, #24165, .T. ) ;
#27713=EDGE_LOOP ( 'NONE', ( #30660, #16244, #25925 ) ) ;
#27716=FACE_OUTER_BOUND ( 'NONE', #27424, .T. ) ;
#27717=B_SPLINE_CURVE_WITH_KNOTS ( 'NONE', 3,
 ( #21336, #11988, #21925, #36775, #3248, #30880 ),
 .UNSPECIFIED., .F., .F.,
 ( 4, 2, 4 ),
 ( 0.000000000000000000, 0.5000000000000000000, 1.000000000000000000 ),
 .UNSPECIFIED. ) ;
#27719=EDGE_CURVE ( 'NONE', #6401, #29611, #1073, .T. ) ;
#27720=DIRECTION ( 'NONE',  ( -0.000000000000000000, -0.000000000000000000, -1.000000000000000000 ) ) ;
#27721=VECTOR ( 'NONE', #1783, 1000.000000000000000 ) ;
#27724=CYLINDRICAL_SURFACE ( 'NONE', #31291, 6.000000000000001776 ) ;
#27727=ADVANCED_FACE ( 'NONE', ( #4211 ), #31643, .F. ) ;
#27729=DIRECTION ( 'NONE',  ( 0.9781476007338042455, -0.2079116908177663370, -0.000000000000000000 ) ) ;
#27731=CARTESIAN_POINT ( 'NONE',  ( -7.824485034907249670, 10.87986945260456295, 7.000000000000000000 ) ) ;
#27732=CARTESIAN_POINT ( 'NONE',  ( 4.524139159579314118, 31.43208625488810171, 10.49999999999999822 ) ) ;
#27736=EDGE_CURVE ( 'NONE', #4444, #27240, #16407, .T. ) ;
#27739=ORIENTED_EDGE ( 'NONE', *, *, #8420, .T. ) ;
#27743=VECTOR ( 'NONE', #35685, 1000.000000000000000 ) ;
#27744=ORIENTED_EDGE ( 'NONE', *, *, #13619, .T. ) ;
#27745=EDGE_CURVE ( 'NONE', #3843, #31103, #29198, .T. ) ;
#27748=EDGE_CURVE ( 'NONE', #19049, #26207, #32252, .T. ) ;
#27749=EDGE_CURVE ( 'NONE', #9605, #35819, #5189, .T. ) ;
#27754=CARTESIAN_POINT ( 'NONE',  ( 6.429307333185271034, 14.50146843380299977, 10.74999999999999289 ) ) ;
#27757=DIRECTION ( 'NONE',  ( -0.000000000000000000, -0.000000000000000000, -1.000000000000000000 ) ) ;
#27758=DIRECTION ( 'NONE',  ( 0.4067366430757884399, -0.9135454576426061957, 0.000000000000000000 ) ) ;
#27761=ORIENTED_EDGE ( 'NONE', *, *, #15860, .T. ) ;
#27763=DIRECTION ( 'NONE',  ( 1.000000000000000000, 0.000000000000000000, 0.000000000000000000 ) ) ;
#27769=ORIENTED_EDGE ( 'NONE', *, *, #10345, .T. ) ;
#27770=FACE_OUTER_BOUND ( 'NONE', #25011, .T. ) ;
#27772=ADVANCED_FACE ( 'NONE', ( #34895 ), #1306, .T. ) ;
#27774=AXIS2_PLACEMENT_3D ( 'NONE', #27386, #6051, #39777 ) ;
#27775=EDGE_CURVE ( 'NONE', #2697, #33983, #16817, .T. ) ;
#27785=ORIENTED_EDGE ( 'NONE', *, *, #23586, .T. ) ;
#27787=AXIS2_PLACEMENT_3D ( 'NONE', #34730, #20098, #16443 ) ;
#27789=ORIENTED_EDGE ( 'NONE', *, *, #18881, .T. ) ;
#27791=CARTESIAN_POINT ( 'NONE',  ( 13.48130249190479368, 27.93180293473185927, 10.49999999999999822 ) ) ;
#27795=DIRECTION ( 'NONE',  ( 0.000000000000000000, 0.000000000000000000, 1.000000000000000000 ) ) ;
#27797=DIRECTION ( 'NONE',  ( 0.7431448254773954654, 0.6691306063588569053, -0.000000000000000000 ) ) ;
#27800=AXIS2_PLACEMENT_3D ( 'NONE', #8707, #31235, #18058 ) ;
#27801=VECTOR ( 'NONE', #13637, 1000.000000000000114 ) ;
#27803=ORIENTED_EDGE ( 'NONE', *, *, #12564, .T. ) ;
#27805=DIRECTION ( 'NONE',  ( -1.000000000000000000, 0.000000000000000000, 0.000000000000000000 ) ) ;
#27806=CARTESIAN_POINT ( 'NONE',  ( -6.811226782241547539, 35.33967249274200384, 11.00000000000000000 ) ) ;
#27808=PLANE ( 'NONE',  #10456 ) ;
#27817=CARTESIAN_POINT ( 'NONE',  ( -1.000000000000000000, 37.00000000000000711, 9.500000000000000000 ) ) ;
#27823=ADVANCED_FACE ( 'NONE', ( #26558 ), #37246, .T. ) ;
#27824=DIRECTION ( 'NONE',  ( 0.9510565162951544194, 0.3090169943749451198, 0.000000000000000000 ) ) ;
#27825=ORIENTED_EDGE ( 'NONE', *, *, #37697, .T. ) ;
#27827=CARTESIAN_POINT ( 'NONE',  ( 0.5000000000000000000, 37.33905845025569903, 10.87262190630138292 ) ) ;
#27828=LINE ( 'NONE', #19084, #26298 ) ;
#27831=CARTESIAN_POINT ( 'NONE',  ( 7.659620408498160060, 26.92228390473674793, 7.000000000000000000 ) ) ;
#27832=ORIENTED_EDGE ( 'NONE', *, *, #20816, .F. ) ;
#27837=B_SPLINE_SURFACE_WITH_KNOTS ( 'NONE', 1, 3, ( 
 ( #716, #38083, #37691, #4156, #10256, #37883, #19807, #22436, #3560, #32199 ),
 ( #29150, #1318, #23049, #28338, #520, #13701, #38489, #10665, #34842, #6993 ) ),
 .UNSPECIFIED., .F., .F., .F.,
 ( 2, 2 ),
 ( 4, 2, 2, 2, 4 ),
 ( 0.000000000000000000, 1.000000000000000000 ),
 ( 4.145433333912467155, 4.538132415611192627, 4.930831497309917211, 5.323530579008641794, 5.716229660707366378 ),
 .UNSPECIFIED. ) ;
#27838=ORIENTED_EDGE ( 'NONE', *, *, #9512, .T. ) ;
#27840=DIRECTION ( 'NONE',  ( -0.000000000000000000, 0.000000000000000000, -1.000000000000000000 ) ) ;
#27841=ORIENTED_EDGE ( 'NONE', *, *, #6521, .T. ) ;
#27846=CARTESIAN_POINT ( 'NONE',  ( -0.6897330713185921836, 37.48434185086841808, 7.485646746502371940 ) ) ;
#27848=DIRECTION ( 'NONE',  ( -0.000000000000000000, 0.000000000000000000, 1.000000000000000000 ) ) ;
#27849=VERTEX_POINT ( 'NONE', #30205 ) ;
#27851=EDGE_CURVE ( 'NONE', #39330, #33798, #10925, .T. ) ;
#27852=CARTESIAN_POINT ( 'NONE',  ( -10.21799113078971466, 32.82168114676807136, 10.66666666666666252 ) ) ;
#27856=VECTOR ( 'NONE', #20423, 1000.000000000000000 ) ;
#27857=CARTESIAN_POINT ( 'NONE',  ( 3.607749162633204332, 7.931741834401770497, 10.49999999999999822 ) ) ;
#27858=ADVANCED_FACE ( 'NONE', ( #39541 ), #8059, .F. ) ;
#27860=PLANE ( 'NONE',  #30119 ) ;
#27861=AXIS2_PLACEMENT_3D ( 'NONE', #29447, #26197, #1626 ) ;
#27868=DIRECTION ( 'NONE',  ( 0.000000000000000000, 0.000000000000000000, 1.000000000000000000 ) ) ;
#27869=ORIENTED_EDGE ( 'NONE', *, *, #5799, .T. ) ;
#27870=ORIENTED_EDGE ( 'NONE', *, *, #13748, .T. ) ;
#27874=EDGE_LOOP ( 'NONE', ( #4240, #3916, #13541, #37088 ) ) ;
#27877=CARTESIAN_POINT ( 'NONE',  ( 0.4999999999999995559, 37.00000000000000711, 11.00000000000000000 ) ) ;
#27881=DIRECTION ( 'NONE',  ( 0.07391278520354631343, -0.7032331762534066444, 0.7071067811865472397 ) ) ;
#27882=EDGE_CURVE ( 'NONE', #23702, #4851, #29861, .T. ) ;
#27883=ORIENTED_EDGE ( 'NONE', *, *, #6542, .F. ) ;
#27887=VECTOR ( 'NONE', #34206, 1000.000000000000000 ) ;
#27892=AXIS2_PLACEMENT_3D ( 'NONE', #13553, #13148, #25539 ) ;
#27893=DIRECTION ( 'NONE',  ( -0.000000000000000000, -0.000000000000000000, 1.000000000000000000 ) ) ;
#27895=LINE ( 'NONE', #9415, #26542 ) ;
#27901=DIRECTION ( 'NONE',  ( 0.9945218953682730678, -0.1045284632676570929, 0.000000000000000000 ) ) ;
#27905=B_SPLINE_CURVE_WITH_KNOTS ( 'NONE', 3,
 ( #19621, #10896, #38512, #23279, #19221, #32015 ),
 .UNSPECIFIED., .F., .F.,
 ( 4, 2, 4 ),
 ( 0.000000000000000000, 0.5000000000000000000, 1.000000000000000000 ),
 .UNSPECIFIED. ) ;
#27906=CARTESIAN_POINT ( 'NONE',  ( -7.530592408761007661, 11.28437794979203090, 10.50000000000000000 ) ) ;
#27908=ORIENTED_EDGE ( 'NONE', *, *, #36353, .T. ) ;
#27911=CARTESIAN_POINT ( 'NONE',  ( 7.111215932167701759, 17.81698729810774751, 9.000000000000001776 ) ) ;
#27913=ORIENTED_EDGE ( 'NONE', *, *, #11994, .F. ) ;
#27914=PLANE ( 'NONE',  #25489 ) ;
#27916=ORIENTED_EDGE ( 'NONE', *, *, #36427, .F. ) ;
#27921=VERTEX_POINT ( 'NONE', #17828 ) ;
#27924=CARTESIAN_POINT ( 'NONE',  ( 10.06946225350410984, 32.23940090176269990, 7.499999999999997335 ) ) ;
#27926=ORIENTED_EDGE ( 'NONE', *, *, #1203, .F. ) ;
#27928=DIRECTION ( 'NONE',  ( 0.000000000000000000, 0.000000000000000000, -1.000000000000000000 ) ) ;
#27929=EDGE_CURVE ( 'NONE', #17936, #17600, #12348, .T. ) ;
#27930=CYLINDRICAL_SURFACE ( 'NONE', #12773, 0.4999999999999988898 ) ;
#27931=EDGE_CURVE ( 'NONE', #28556, #7248, #27255, .T. ) ;
#27933=ORIENTED_EDGE ( 'NONE', *, *, #22920, .T. ) ;
#27936=AXIS2_PLACEMENT_3D ( 'NONE', #5562, #21404, #12456 ) ;
#27937=CARTESIAN_POINT ( 'NONE',  ( -4.984135866956333594, 36.15314577889358105, 10.49999999999999822 ) ) ;
#27939=ORIENTED_EDGE ( 'NONE', *, *, #17749, .F. ) ;
#27941=PLANE ( 'NONE',  #30345 ) ;
#27942=EDGE_LOOP ( 'NONE', ( #12211, #2845, #15098, #39385 ) ) ;
#27943=CIRCLE ( 'NONE', #21483, 0.5000000000000007772 ) ;
#27944=DIRECTION ( 'NONE',  ( 0.5877852522924690293, -0.8090169943749503378, 0.000000000000000000 ) ) ;
#27949=CARTESIAN_POINT ( 'NONE',  ( 7.126083911573384277, 10.99048532364570185, 10.00000000000000000 ) ) ;
#27950=DIRECTION ( 'NONE',  ( -0.000000000000000000, -0.000000000000000000, -1.000000000000000000 ) ) ;
#27953=CARTESIAN_POINT ( 'NONE',  ( 11.54666566735224364, 32.07468077621332725, 7.499999999999997335 ) ) ;
#27956=DIRECTION ( 'NONE',  ( 0.3090169943749560000, 0.9510565162951507556, 0.000000000000000000 ) ) ;
#27957=ORIENTED_EDGE ( 'NONE', *, *, #8503, .T. ) ;
#27960=DIRECTION ( 'NONE',  ( 0.5877852522924690293, -0.8090169943749503378, 0.000000000000000000 ) ) ;
#27961=CARTESIAN_POINT ( 'NONE',  ( 13.10100158617407295, 15.51348347675824435, 10.87262190629279779 ) ) ;
#27967=ORIENTED_EDGE ( 'NONE', *, *, #5399, .F. ) ;
#27975=CARTESIAN_POINT ( 'NONE',  ( -9.197066986886744289, 11.25907462514039814, 10.66666666666666785 ) ) ;
#27978=ORIENTED_EDGE ( 'NONE', *, *, #34375, .T. ) ;
#27984=CARTESIAN_POINT ( 'NONE',  ( -6.282361020112263716, 14.70372268239681190, 10.50000000000000533 ) ) ;
#27988=VECTOR ( 'NONE', #24955, 1000.000000000000114 ) ;
#27989=AXIS2_PLACEMENT_3D ( 'NONE', #19101, #20311, #35546 ) ;
#27990=EDGE_LOOP ( 'NONE', ( #16574, #23197, #11877, #37542, #8954 ) ) ;
#27992=ORIENTED_EDGE ( 'NONE', *, *, #33340, .F. ) ;
#27993=FACE_OUTER_BOUND ( 'NONE', #11558, .T. ) ;
#27994=CARTESIAN_POINT ( 'NONE',  ( 8.315274455032099610, 10.01576150750513072, 7.000000000000000000 ) ) ;
#27995=EDGE_CURVE ( 'NONE', #11401, #1059, #12700, .T. ) ;
#27996=CARTESIAN_POINT ( 'NONE',  ( 0.5000000000000012212, 31.00000000000000355, 9.000000000000001776 ) ) ;
#27997=ORIENTED_EDGE ( 'NONE', *, *, #5416, .F. ) ;
#28000=CARTESIAN_POINT ( 'NONE',  ( -4.577399223880545875, 35.23960032125098252, 10.50000000000000000 ) ) ;
#28003=LINE ( 'NONE', #31255, #17625 ) ;
#28004=DIRECTION ( 'NONE',  ( 0.6691306063588671194, 0.7431448254773863615, -0.000000000000000000 ) ) ;
#28006=ORIENTED_EDGE ( 'NONE', *, *, #12854, .T. ) ;
#28007=EDGE_CURVE ( 'NONE', #31457, #37999, #22719, .T. ) ;
#28009=CARTESIAN_POINT ( 'NONE',  ( -14.78578095943786153, 19.97317811133652654, 7.339470489435494294 ) ) ;
#28011=CARTESIAN_POINT ( 'NONE',  ( -5.473344025737326035, 14.11593743010433677, 10.50000000000000178 ) ) ;
#28014=LINE ( 'NONE', #24969, #30424 ) ;
#28021=LINE ( 'NONE', #28219, #16384 ) ;
#28022=VERTEX_POINT ( 'NONE', #21648 ) ;
#28024=ADVANCED_FACE ( 'NONE', ( #31196 ), #34253, .T. ) ;
#28026=CARTESIAN_POINT ( 'NONE',  ( -13.05736835487441994, 16.11602540378456183, 10.49999999999999822 ) ) ;
#28027=ADVANCED_FACE ( 'NONE', ( #34052 ), #6210, .F. ) ;
#28028=DIRECTION ( 'NONE',  ( 0.8660254037844364872, -0.5000000000000038858, 0.000000000000000000 ) ) ;
#28031=CARTESIAN_POINT ( 'NONE',  ( 14.46401681939182993, 26.47472063362052808, 7.485699520496980952 ) ) ;
#28032=AXIS2_PLACEMENT_3D ( 'NONE', #5051, #32287, #4448 ) ;
#28033=CARTESIAN_POINT ( 'NONE',  ( 3.607749162633204332, 7.931741834401770497, 11.00000000000000000 ) ) ;
#28037=ORIENTED_EDGE ( 'NONE', *, *, #27299, .T. ) ;
#28041=LINE ( 'NONE', #3658, #4758 ) ;
#28042=LINE ( 'NONE', #28441, #37709 ) ;
#28045=CARTESIAN_POINT ( 'NONE',  ( -2.568190708544554557, 12.82247983807085134, 10.50000000000000533 ) ) ;
#28046=VERTEX_POINT ( 'NONE', #18811 ) ;
#28047=ADVANCED_FACE ( 'NONE', ( #3362 ), #15754, .F. ) ;
#28050=CARTESIAN_POINT ( 'NONE',  ( 12.51556656179726801, 14.23165457969784597, 7.381627713044569106 ) ) ;
#28051=CARTESIAN_POINT ( 'NONE',  ( -7.096882951594430722, 29.56287847632736288, 10.49999999999999822 ) ) ;
#28053=VECTOR ( 'NONE', #23992, 999.9999999999998863 ) ;
#28055=DIRECTION ( 'NONE',  ( 0.8660254037844363761, -0.5000000000000039968, -0.000000000000000000 ) ) ;
#28056=B_SPLINE_CURVE_WITH_KNOTS ( 'NONE', 3,
 ( #15786, #27975, #31620, #150 ),
 .UNSPECIFIED., .F., .F.,
 ( 4, 4 ),
 ( 0.000000000000000000, 1.000000000000000000 ),
 .UNSPECIFIED. ) ;
#28057=FACE_OUTER_BOUND ( 'NONE', #964, .T. ) ;
#28058=ORIENTED_EDGE ( 'NONE', *, *, #16400, .F. ) ;
#28060=VECTOR ( 'NONE', #4951, 1000.000000000000000 ) ;
#28063=DIRECTION ( 'NONE',  ( -0.2079116908177532363, 0.9781476007338070211, 0.000000000000000000 ) ) ;
#28064=VERTEX_POINT ( 'NONE', #36704 ) ;
#28068=SHAPE_REPRESENTATION ( 'Dual-Edge Stainless Steel Rotary Blade', ( #24238 ), #11913 ) ;
#28076=PLANE ( 'NONE',  #13495 ) ;
#28077=DIRECTION ( 'NONE',  ( -0.000000000000000000, -0.000000000000000000, -1.000000000000000000 ) ) ;
#28078=ADVANCED_FACE ( 'NONE', ( #21258 ), #5816, .F. ) ;
#28081=ORIENTED_EDGE ( 'NONE', *, *, #19484, .T. ) ;
#28085=ORIENTED_EDGE ( 'NONE', *, *, #4667, .F. ) ;
#28089=DIRECTION ( 'NONE',  ( 1.000000000000000000, 3.469446951953563307E-15, 0.000000000000000000 ) ) ;
#28092=DIRECTION ( 'NONE',  ( 0.5000000000000038858, 0.8660254037844363761, 0.000000000000000000 ) ) ;
#28098=CARTESIAN_POINT ( 'NONE',  ( 7.645071344821493753, 9.594463043616155318, 7.000000000000000000 ) ) ;
#28099=EDGE_CURVE ( 'NONE', #7567, #27126, #33860, .T. ) ;
#28100=CARTESIAN_POINT ( 'NONE',  ( -9.363324537585850038, 32.27640801132209702, 10.00000000000000000 ) ) ;
#28102=CARTESIAN_POINT ( 'NONE',  ( 9.665073660139013256, 25.11464168560187460, 10.50000000000000533 ) ) ;
#28104=AXIS2_PLACEMENT_3D ( 'NONE', #17287, #23569, #29857 ) ;
#28105=ORIENTED_EDGE ( 'NONE', *, *, #19818, .F. ) ;
#28108=MECHANICAL_DESIGN_GEOMETRIC_PRESENTATION_REPRESENTATION('',(#34607),#26844);
#28111=ORIENTED_EDGE ( 'NONE', *, *, #11757, .T. ) ;
#28112=CARTESIAN_POINT ( 'NONE',  ( 7.530592408760855783, 11.28437794979193498, 10.50000000000000000 ) ) ;
#28115=DIRECTION ( 'NONE',  ( 0.6691306063588571273, -0.7431448254773953543, 0.000000000000000000 ) ) ;
#28117=DIRECTION ( 'NONE',  ( 0.1045284632676570929, 0.9945218953682730678, 0.000000000000000000 ) ) ;
#28118=AXIS2_PLACEMENT_3D ( 'NONE', #30656, #27004, #11762 ) ;
#28119=ORIENTED_EDGE ( 'NONE', *, *, #36845, .T. ) ;
#28122=DIRECTION ( 'NONE',  ( 0.1045284632676415082, -0.9945218953682745111, 0.000000000000000000 ) ) ;
#28124=ORIENTED_EDGE ( 'NONE', *, *, #30939, .T. ) ;
#28127=CARTESIAN_POINT ( 'NONE',  ( -11.11016527260153630, 31.83082137946488643, 7.000000000000000000 ) ) ;
#28128=CARTESIAN_POINT ( 'NONE',  ( -8.339609403135948895, 11.87216320208451137, 9.500000000000000000 ) ) ;
#28130=ORIENTED_EDGE ( 'NONE', *, *, #3414, .F. ) ;
#28134=EDGE_CURVE ( 'NONE', #28389, #26241, #30805, .T. ) ;
#28136=ORIENTED_EDGE ( 'NONE', *, *, #1106, .F. ) ;
#28139=VECTOR ( 'NONE', #28601, 1000.000000000000000 ) ;
#28140=CARTESIAN_POINT ( 'NONE',  ( -17.05532387642082526, 7.816133769664412867, 11.00000000000000000 ) ) ;
#28141=ORIENTED_EDGE ( 'NONE', *, *, #14977, .F. ) ;
#28142=B_SPLINE_CURVE_WITH_KNOTS ( 'NONE', 3,
 ( #2854, #19090, #16041, #6682, #15844, #37378 ),
 .UNSPECIFIED., .F., .F.,
 ( 4, 2, 4 ),
 ( 0.000000000000000000, 0.5000000000000000000, 1.000000000000000000 ),
 .UNSPECIFIED. ) ;
#28148=EDGE_CURVE ( 'NONE', #6243, #38307, #16156, .T. ) ;
#28150=EDGE_CURVE ( 'NONE', #20144, #25142, #22237, .T. ) ;
#28151=CARTESIAN_POINT ( 'NONE',  ( 7.766013557953383106, 28.81973365084986938, 10.50000000000000178 ) ) ;
#28154=CARTESIAN_POINT ( 'NONE',  ( 8.238488885696289898, 24.65111619403943877, 9.000000000000001776 ) ) ;
#28156=DIRECTION ( 'NONE',  ( 0.9781476007338042455, -0.2079116908177663370, -0.000000000000000000 ) ) ;
#28157=ORIENTED_EDGE ( 'NONE', *, *, #9312, .F. ) ;
#28159=DIRECTION ( 'NONE',  ( 1.000000000000000000, -1.387778780781439522E-14, 0.000000000000000000 ) ) ;
#28160=VECTOR ( 'NONE', #7961, 1000.000000000000000 ) ;
#28161=CARTESIAN_POINT ( 'NONE',  ( 12.84742388243086175, 15.65988663227523325, 11.00000000000000000 ) ) ;
#28166=B_SPLINE_SURFACE_WITH_KNOTS ( 'NONE', 1, 3, ( 
 ( #26723, #8441, #24076, #11092, #33638, #29968, #5188, #21031, #17599, #8030 ),
 ( #39109, #17993, #5386, #33039, #20837, #21226, #14735, #27125, #26527, #36669 ) ),
 .UNSPECIFIED., .F., .F., .F.,
 ( 2, 2 ),
 ( 4, 2, 2, 2, 4 ),
 ( 0.000000000000000000, 1.000000000000000000 ),
 ( 4.638205445319954379, 5.030904527018678074, 5.423603608717401769, 5.816302690416126353, 6.209001772114850048 ),
 .UNSPECIFIED. ) ;
#28167=ORIENTED_EDGE ( 'NONE', *, *, #4304, .T. ) ;
#28168=CARTESIAN_POINT ( 'NONE',  ( 5.400683141673458643, 15.91724817395916070, 7.000000000000000000 ) ) ;
#28171=AXIS2_PLACEMENT_3D ( 'NONE', #23417, #35809, #33175 ) ;
#28177=VERTEX_POINT ( 'NONE', #13294 ) ;
#28179=EDGE_CURVE ( 'NONE', #24685, #37754, #25888, .T. ) ;
#28180=AXIS2_PLACEMENT_3D ( 'NONE', #15957, #34639, #34051 ) ;
#28182=ORIENTED_EDGE ( 'NONE', *, *, #17627, .F. ) ;
#28183=CARTESIAN_POINT ( 'NONE',  ( 1.853849799106296548, 7.614518279115737087, 7.102474990965861323 ) ) ;
#28184=DIRECTION ( 'NONE',  ( 0.2079116908177663370, 0.9781476007338042455, -0.000000000000000000 ) ) ;
#28190=ORIENTED_EDGE ( 'NONE', *, *, #14562, .F. ) ;
#28198=LINE ( 'NONE', #27806, #26041 ) ;
#28199=EDGE_CURVE ( 'NONE', #1436, #11472, #20129, .T. ) ;
#28202=LINE ( 'NONE', #31256, #39210 ) ;
#28203=LINE ( 'NONE', #4013, #21610 ) ;
#28205=AXIS2_PLACEMENT_3D ( 'NONE', #3953, #27058, #25887 ) ;
#28210=CARTESIAN_POINT ( 'NONE',  ( 14.57486473880226008, 26.18419839932902349, 10.49999999999999822 ) ) ;
#28213=CARTESIAN_POINT ( 'NONE',  ( -14.11133924723978161, 27.61078317377194224, 10.49999999999999822 ) ) ;
#28218=CARTESIAN_POINT ( 'NONE',  ( 14.11133924723984201, 27.61078317377175040, 10.49999999999999822 ) ) ;
#28219=CARTESIAN_POINT ( 'NONE',  ( -2.256323172317921788, 14.28970123917155277, 9.000000000000001776 ) ) ;
#28224=DIRECTION ( 'NONE',  ( 1.000000000000000000, 0.000000000000000000, 0.000000000000000000 ) ) ;
#28226=DIRECTION ( 'NONE',  ( 0.000000000000000000, 0.000000000000000000, 1.000000000000000000 ) ) ;
#28227=ORIENTED_EDGE ( 'NONE', *, *, #4814, .T. ) ;
#28229=ADVANCED_FACE ( 'NONE', ( #38288 ), #31586, .F. ) ;
#28231=ADVANCED_FACE ( 'NONE', ( #28541 ), #27837, .T. ) ;
#28234=AXIS2_PLACEMENT_3D ( 'NONE', #35671, #9634, #24466 ) ;
#28237=ORIENTED_EDGE ( 'NONE', *, *, #34744, .F. ) ;
#28239=VECTOR ( 'NONE', #22103, 999.9999999999998863 ) ;
#28240=EDGE_CURVE ( 'NONE', #36832, #23885, #19394, .T. ) ;
#28241=VECTOR ( 'NONE', #5294, 1000.000000000000000 ) ;
#28242=ORIENTED_EDGE ( 'NONE', *, *, #37077, .T. ) ;
#28248=ORIENTED_EDGE ( 'NONE', *, *, #13737, .F. ) ;
#28251=DIRECTION ( 'NONE',  ( 1.000000000000000000, 0.000000000000000000, 0.000000000000000000 ) ) ;
#28253=EDGE_CURVE ( 'NONE', #17719, #37972, #31798, .T. ) ;
#28255=ADVANCED_FACE ( 'NONE', ( #31992 ), #28940, .F. ) ;
#28260=CARTESIAN_POINT ( 'NONE',  ( 0.6894430450595149251, 37.48435367156681508, 7.485699520496978288 ) ) ;
#28261=EDGE_LOOP ( 'NONE', ( #28351, #7551, #4510, #15444, #38268 ) ) ;
#28263=AXIS2_PLACEMENT_3D ( 'NONE', #8692, #18042, #36726 ) ;
#28267=ORIENTED_EDGE ( 'NONE', *, *, #6545, .T. ) ;
#28271=EDGE_CURVE ( 'NONE', #8524, #11294, #139, .T. ) ;
#28272=CARTESIAN_POINT ( 'NONE',  ( 14.31603901957230462, 19.98981538725069740, 10.50000000000000533 ) ) ;
#28273=ORIENTED_EDGE ( 'NONE', *, *, #37956, .F. ) ;
#28276=CARTESIAN_POINT ( 'NONE',  ( -2.806807826039845022, 9.295007390093649846, 7.000000000000000000 ) ) ;
#28277=ORIENTED_EDGE ( 'NONE', *, *, #29518, .F. ) ;
#28280=CARTESIAN_POINT ( 'NONE',  ( 3.503793317224327186, 8.420815634768674229, 7.499999999999990230 ) ) ;
#28281=DIRECTION ( 'NONE',  ( 0.4067366430758010409, 0.9135454576426005335, -0.000000000000000000 ) ) ;
#28282=ORIENTED_EDGE ( 'NONE', *, *, #11486, .T. ) ;
#28288=ORIENTED_EDGE ( 'NONE', *, *, #13207, .F. ) ;
#28289=AXIS2_PLACEMENT_3D ( 'NONE', #32325, #18487, #1 ) ;
#28290=CARTESIAN_POINT ( 'NONE',  ( 14.44277748876681855, 26.55045409923015853, 7.500000000000000888 ) ) ;
#28292=VECTOR ( 'NONE', #24115, 1000.000000000000000 ) ;
#28293=AXIS2_PLACEMENT_3D ( 'NONE', #17850, #24329, #14788 ) ;
#28294=CARTESIAN_POINT ( 'NONE',  ( 14.26377478793847509, 19.49255443956654688, 7.000000000000000000 ) ) ;
#28295=AXIS2_PLACEMENT_3D ( 'NONE', #7064, #1186, #34709 ) ;
#28298=DIRECTION ( 'NONE',  ( 0.000000000000000000, 0.000000000000000000, -1.000000000000000000 ) ) ;
#28306=CARTESIAN_POINT ( 'NONE',  ( 10.79197459925287816, 32.88995393992981775, 10.68306085400109495 ) ) ;
#28308=ORIENTED_EDGE ( 'NONE', *, *, #3598, .T. ) ;
#28310=VERTEX_POINT ( 'NONE', #12216 ) ;
#28314=CARTESIAN_POINT ( 'NONE',  ( 12.71633695260870844, 14.58086916811563150, 10.68306085400105943 ) ) ;
#28315=AXIS2_PLACEMENT_3D ( 'NONE', #31814, #10483, #28566 ) ;
#28316=EDGE_LOOP ( 'NONE', ( #7383, #28528, #9464, #27609 ) ) ;
#28319=CARTESIAN_POINT ( 'NONE',  ( 15.00099999999999767, 36.00000000000000711, 9.500000000000000000 ) ) ;
#28321=ORIENTED_EDGE ( 'NONE', *, *, #352, .F. ) ;
#28323=CIRCLE ( 'NONE', #23137, 15.00000000000000000 ) ;
#28326=DIRECTION ( 'NONE',  ( -0.000000000000000000, -0.000000000000000000, -1.000000000000000000 ) ) ;
#28334=ORIENTED_EDGE ( 'NONE', *, *, #21690, .F. ) ;
#28335=PLANE ( 'NONE',  #1569 ) ;
#28337=AXIS2_PLACEMENT_3D ( 'NONE', #22409, #32381, #22210 ) ;
#28338=CARTESIAN_POINT ( 'NONE',  ( -11.61617238037479538, 31.85261655609473408, 10.49999999999999822 ) ) ;
#28339=CARTESIAN_POINT ( 'NONE',  ( 3.503793317224329851, 8.420815634768676006, 9.000000000000001776 ) ) ;
#28341=DIRECTION ( 'NONE',  ( 0.000000000000000000, 0.000000000000000000, 1.000000000000000000 ) ) ;
#28342=ADVANCED_FACE ( 'NONE', ( #33020 ), #1728, .T. ) ;
#28344=DIRECTION ( 'NONE',  ( 0.8660254037844363761, -0.5000000000000039968, 0.000000000000000000 ) ) ;
#28345=FACE_OUTER_BOUND ( 'NONE', #10223, .T. ) ;
#28347=DIRECTION ( 'NONE',  ( 0.000000000000000000, -0.7071067811865474617, -0.7071067811865474617 ) ) ;
#28350=CARTESIAN_POINT ( 'NONE',  ( 5.440908595777814050, 35.94977745735560859, 7.000000000000000000 ) ) ;
#28351=ORIENTED_EDGE ( 'NONE', *, *, #4512, .T. ) ;
#28353=CARTESIAN_POINT ( 'NONE',  ( 2.061816823438564761, 8.019625857903918131, 10.49999999999999822 ) ) ;
#28354=EDGE_CURVE ( 'NONE', #8840, #25521, #8421, .T. ) ;
#28355=CARTESIAN_POINT ( 'NONE',  ( 21.39877161664088590, 15.54711762656346075, 11.00000000000000000 ) ) ;
#28357=EDGE_CURVE ( 'NONE', #21780, #2164, #7606, .T. ) ;
#28361=EDGE_LOOP ( 'NONE', ( #17644, #16969, #18314, #23340 ) ) ;
#28362=CYLINDRICAL_SURFACE ( 'NONE', #4924, 6.000000000000003553 ) ;
#28370=LINE ( 'NONE', #3202, #19950 ) ;
#28372=ORIENTED_EDGE ( 'NONE', *, *, #32753, .T. ) ;
#28374=AXIS2_PLACEMENT_3D ( 'NONE', #6534, #28281, #19137 ) ;
#28375=AXIS2_PLACEMENT_3D ( 'NONE', #14594, #2405, #39369 ) ;
#28378=CARTESIAN_POINT ( 'NONE',  ( -9.997483185316569987, 21.95197631500770896, 10.49999999999999467 ) ) ;
#28380=DIRECTION ( 'NONE',  ( -0.1470157664651899898, 0.6916548014802332833, -0.7071067811865417996 ) ) ;
#28381=EDGE_CURVE ( 'NONE', #5904, #18376, #13909, .T. ) ;
#28388=ORIENTED_EDGE ( 'NONE', *, *, #28357, .F. ) ;
#28389=VERTEX_POINT ( 'NONE', #38696 ) ;
#28390=DIRECTION ( 'NONE',  ( 1.000000000000000000, 1.224646799147351235E-16, -0.000000000000000000 ) ) ;
#28392=CARTESIAN_POINT ( 'NONE',  ( -7.468455364333119739, 29.89744377950679421, 10.50000000000000000 ) ) ;
#28393=ORIENTED_EDGE ( 'NONE', *, *, #24546, .T. ) ;
#28396=FACE_OUTER_BOUND ( 'NONE', #35227, .T. ) ;
#28398=DIRECTION ( 'NONE',  ( -0.9781476007338070211, -0.2079116908177534029, 0.000000000000000000 ) ) ;
#28399=DIRECTION ( 'NONE',  ( -0.9135454576426004225, 0.4067366430758009854, 0.000000000000000000 ) ) ;
#28401=DIRECTION ( 'NONE',  ( -0.2185080122243950040, 0.6724985119639662612, 0.7071067811865437980 ) ) ;
#28402=CIRCLE ( 'NONE', #38793, 1.000000000000000888 ) ;
#28405=ORIENTED_EDGE ( 'NONE', *, *, #20314, .T. ) ;
#28407=CARTESIAN_POINT ( 'NONE',  ( -5.644276917315533382, 36.40655018617698602, 11.00000000000000000 ) ) ;
#28413=VECTOR ( 'NONE', #39819, 1000.000000000000000 ) ;
#28418=CARTESIAN_POINT ( 'NONE',  ( 13.86243997625764557, 27.52991089825170690, 10.94387467463490538 ) ) ;
#28419=CARTESIAN_POINT ( 'NONE',  ( 11.44473057578109199, 31.45924896672603310, 10.50000000000000178 ) ) ;
#28420=ORIENTED_EDGE ( 'NONE', *, *, #20615, .T. ) ;
#28422=CARTESIAN_POINT ( 'NONE',  ( 12.37435565298211415, 15.93301270189216545, 7.499999999999997335 ) ) ;
#28423=DIRECTION ( 'NONE',  ( -1.000000000000000000, 0.000000000000000000, 0.000000000000000000 ) ) ;
#28424=EDGE_LOOP ( 'NONE', ( #28227, #34385, #20024, #10580, #12052, #25308, #27136, #27476, #8304, #22412, #30229, #103, #762, #20556, #17108, #28485, #19515, #30463, #3792, #38614, #27978, #22130, #16378, #36583, #8889, #6021, #27602, #40170, #16979, #27533, #27803, #2100, #20465, #33104, #612, #1171, #809, #33582, #34249, #13149, #40119, #5147, #13259, #38804, #23029, #32634, #17994, #14365, #14088, #31673, #18846, #2, #31810, #18687, #35622, #17219, #20303, #38251, #29674, #14491, #38984, #21416, #32105, #18966, #5754, #29035, #13190, #18894, #11578, #6522, #22258, #12530, #39110, #2269, #16686, #19687, #20541, #27789, #26916, #18798, #1544, #23205, #6780, #37422, #6096, #16602, #24415, #28522, #17124, #37216, #21119, #21352, #36884, #14958, #15595, #17414, #24070, #9080, #27462, #29274, #30160 ) ) ;
#28428=CARTESIAN_POINT ( 'NONE',  ( 0.6108529249775871417, 37.48755679569043053, 7.500000000000000888 ) ) ;
#28430=VERTEX_POINT ( 'NONE', #27653 ) ;
#28435=AXIS2_PLACEMENT_3D ( 'NONE', #28831, #22328, #35333 ) ;
#28436=AXIS2_PLACEMENT_3D ( 'NONE', #36038, #8198, #11657 ) ;
#28441=CARTESIAN_POINT ( 'NONE',  ( 15.00099999999999767, 36.50000000000000711, 7.500000000000000888 ) ) ;
#28443=VECTOR ( 'NONE', #5253, 1000.000000000000114 ) ;
#28450=ADVANCED_FACE ( 'NONE', ( #23456 ), #8467, .T. ) ;
#28453=ORIENTED_EDGE ( 'NONE', *, *, #5599, .F. ) ;
#28456=CARTESIAN_POINT ( 'NONE',  ( 5.767236651883453469, 13.71142893291679954, 11.00000000000000000 ) ) ;
#28460=CONICAL_SURFACE ( 'NONE', #24555, 1.000000000000000888, 0.7853981633974552734 ) ;
#28463=CARTESIAN_POINT ( 'NONE',  ( 8.160254037844357100, 16.63397459621552699, 10.49999999999999822 ) ) ;
#28464=ORIENTED_EDGE ( 'NONE', *, *, #37409, .T. ) ;
#28465=VERTEX_POINT ( 'NONE', #20417 ) ;
#28466=AXIS2_PLACEMENT_3D ( 'NONE', #22190, #18561, #3310 ) ;
#28468=CARTESIAN_POINT ( 'NONE',  ( -13.95683075005229767, 28.08631143191951196, 11.00000000000000000 ) ) ;
#28472=DIRECTION ( 'NONE',  ( 0.4067366430758009299, 0.9135454576426005335, 0.000000000000000000 ) ) ;
#28476=LINE ( 'NONE', #19739, #4357 ) ;
#28477=ORIENTED_EDGE ( 'NONE', *, *, #12718, .F. ) ;
#28478=EDGE_CURVE ( 'NONE', #38994, #3204, #25967, .T. ) ;
#28481=EDGE_CURVE ( 'NONE', #3501, #35666, #4566, .T. ) ;
#28485=ORIENTED_EDGE ( 'NONE', *, *, #13491, .T. ) ;
#28489=VECTOR ( 'NONE', #27357, 1000.000000000000000 ) ;
#28491=DIRECTION ( 'NONE',  ( 0.6916548014802318400, -0.1470157664651868257, 0.7071067811865437980 ) ) ;
#28492=AXIS2_PLACEMENT_3D ( 'NONE', #6107, #12609, #37392 ) ;
#28494=EDGE_CURVE ( 'NONE', #19954, #4096, #37660, .T. ) ;
#28495=CARTESIAN_POINT ( 'NONE',  ( -11.20744270277957888, 31.91841037101610112, 10.99999999999999822 ) ) ;
#28500=DIRECTION ( 'NONE',  ( 1.224646799147351235E-16, -1.000000000000000000, 0.000000000000000000 ) ) ;
#28502=VERTEX_POINT ( 'NONE', #33955 ) ;
#28504=EDGE_CURVE ( 'NONE', #21190, #9720, #37792, .T. ) ;
#28506=DIRECTION ( 'NONE',  ( -0.9781476007338041345, 0.2079116908177664202, 0.000000000000000000 ) ) ;
#28508=EDGE_LOOP ( 'NONE', ( #28563, #38987, #38941, #36590, #32011 ) ) ;
#28510=DIRECTION ( 'NONE',  ( -0.000000000000000000, -0.000000000000000000, -1.000000000000000000 ) ) ;
#28513=DIRECTION ( 'NONE',  ( -0.4067366430758009299, -0.9135454576426005335, 0.000000000000000000 ) ) ;
#28515=DIRECTION ( 'NONE',  ( -0.000000000000000000, 0.000000000000000000, 1.000000000000000000 ) ) ;
#28516=AXIS2_PLACEMENT_3D ( 'NONE', #8219, #8624, #23861 ) ;
#28517=ORIENTED_EDGE ( 'NONE', *, *, #12061, .F. ) ;
#28522=ORIENTED_EDGE ( 'NONE', *, *, #20329, .T. ) ;
#28525=DIRECTION ( 'NONE',  ( -0.9945218953682729568, 0.1045284632676569680, 0.000000000000000000 ) ) ;
#28526=CARTESIAN_POINT ( 'NONE',  ( -10.44367147699325749, 33.07775263288209544, 10.49999999999999822 ) ) ;
#28528=ORIENTED_EDGE ( 'NONE', *, *, #3090, .T. ) ;
#28531=EDGE_CURVE ( 'NONE', #35565, #37355, #27261, .T. ) ;
#28534=ORIENTED_EDGE ( 'NONE', *, *, #29703, .F. ) ;
#28537=ORIENTED_EDGE ( 'NONE', *, *, #37481, .F. ) ;
#28538=B_SPLINE_CURVE_WITH_KNOTS ( 'NONE', 3,
 ( #17427, #33468, #8261, #5814, #39538, #21254, #11717, #23903 ),
 .UNSPECIFIED., .F., .F.,
 ( 4, 2, 2, 4 ),
 ( 0.000000000000000000, 0.0004726692273637239823, 0.0007090038410455826124, 0.0009453384547274412426 ),
 .UNSPECIFIED. ) ;
#28539=DIRECTION ( 'NONE',  ( 0.7431448254773848072, -0.6691306063588687847, -0.000000000000000000 ) ) ;
#28540=VECTOR ( 'NONE', #25055, 1000.000000000000000 ) ;
#28541=FACE_OUTER_BOUND ( 'NONE', #37870, .T. ) ;
#28544=EDGE_CURVE ( 'NONE', #38824, #5904, #18719, .T. ) ;
#28545=LINE ( 'NONE', #27949, #25012 ) ;
#28546=ORIENTED_EDGE ( 'NONE', *, *, #27524, .T. ) ;
#28547=CARTESIAN_POINT ( 'NONE',  ( -6.451376067920914892, 35.76073122304934060, 10.94387467463487873 ) ) ;
#28550=AXIS2_PLACEMENT_3D ( 'NONE', #33666, #11916, #25097 ) ;
#28551=CARTESIAN_POINT ( 'NONE',  ( -12.05736835487443237, 14.38397459621567442, 7.000000000000000000 ) ) ;
#28552=DIRECTION ( 'NONE',  ( -0.8090169943749504489, -0.5877852522924689183, 0.000000000000000000 ) ) ;
#28555=CARTESIAN_POINT ( 'NONE',  ( 2.525645716490518389, 8.212903943950921715, 7.000000000000000000 ) ) ;
#28556=VERTEX_POINT ( 'NONE', #31107 ) ;
#28558=CARTESIAN_POINT ( 'NONE',  ( 2.629601561899389761, 7.723830143584008212, 10.49999999999999822 ) ) ;
#28561=CARTESIAN_POINT ( 'NONE',  ( 12.30736835487432579, 14.81698729810772619, 7.000000000000000000 ) ) ;
#28563=ORIENTED_EDGE ( 'NONE', *, *, #34579, .F. ) ;
#28566=DIRECTION ( 'NONE',  ( 0.9510565162951544194, 0.3090169943749450643, 0.000000000000000000 ) ) ;
#28569=AXIS2_PLACEMENT_3D ( 'NONE', #27598, #9517, #3409 ) ;
#28573=ORIENTED_EDGE ( 'NONE', *, *, #17159, .F. ) ;
#28575=DIRECTION ( 'NONE',  ( 0.8090169943749510040, 0.5877852522924683631, 0.000000000000000000 ) ) ;
#28584=AXIS2_PLACEMENT_3D ( 'NONE', #31897, #16467, #7304 ) ;
#28588=ORIENTED_EDGE ( 'NONE', *, *, #34124, .T. ) ;
#28589=ORIENTED_EDGE ( 'NONE', *, *, #8528, .F. ) ;
#28590=FACE_OUTER_BOUND ( 'NONE', #18476, .T. ) ;
#28592=AXIS2_PLACEMENT_3D ( 'NONE', #10412, #16716, #35192 ) ;
#28596=AXIS2_PLACEMENT_3D ( 'NONE', #20473, #33273, #5223 ) ;
#28597=DIRECTION ( 'NONE',  ( -0.4999999999999920064, 0.8660254037844432595, 0.000000000000000000 ) ) ;
#28598=FACE_OUTER_BOUND ( 'NONE', #23589, .T. ) ;
#28599=CARTESIAN_POINT ( 'NONE',  ( -12.11016527260154163, 31.83082137946488643, 7.000000000000000000 ) ) ;
#28601=DIRECTION ( 'NONE',  ( -0.000000000000000000, -0.000000000000000000, -1.000000000000000000 ) ) ;
#28603=CARTESIAN_POINT ( 'NONE',  ( 13.63581098909226874, 27.45627467658428955, 7.500000000000000888 ) ) ;
#28606=DIRECTION ( 'NONE',  ( -0.000000000000000000, -0.000000000000000000, -1.000000000000000000 ) ) ;
#28608=ADVANCED_FACE ( 'NONE', ( #37604 ), #3866, .T. ) ;
#28610=DIRECTION ( 'NONE',  ( -0.000000000000000000, -0.000000000000000000, 1.000000000000000000 ) ) ;
#28614=CARTESIAN_POINT ( 'NONE',  ( 13.47830981910552239, 21.58612669357077607, 9.500000000000000000 ) ) ;
#28620=CARTESIAN_POINT ( 'NONE',  ( 14.31603901957230462, 19.98981538725069740, 11.00000000000000000 ) ) ;
#28622=ORIENTED_EDGE ( 'NONE', *, *, #29626, .F. ) ;
#28624=AXIS2_PLACEMENT_3D ( 'NONE', #22149, #6702, #16060 ) ;
#28625=CARTESIAN_POINT ( 'NONE',  ( 14.51883047965004891, 21.47676356526602959, 10.99999999999999289 ) ) ;
#28626=VERTEX_POINT ( 'NONE', #12810 ) ;
#28632=ORIENTED_EDGE ( 'NONE', *, *, #37178, .F. ) ;
#28639=CIRCLE ( 'NONE', #36450, 15.00000000000000000 ) ;
#28641=EDGE_CURVE ( 'NONE', #3294, #6428, #20158, .T. ) ;
#28642=FACE_OUTER_BOUND ( 'NONE', #13108, .T. ) ;
#28645=CARTESIAN_POINT ( 'NONE',  ( -0.5000000000000005551, 31.00000000000000355, 9.000000000000001776 ) ) ;
#28646=ORIENTED_EDGE ( 'NONE', *, *, #5903, .F. ) ;
#28647=DIRECTION ( 'NONE',  ( 0.9781476007338042455, -0.2079116908177656431, 0.000000000000000000 ) ) ;
#28649=CARTESIAN_POINT ( 'NONE',  ( -8.927394655428429360, 11.06314620770957013, 7.500000000000000888 ) ) ;
#28654=EDGE_CURVE ( 'NONE', #4036, #10907, #3471, .T. ) ;
#28655=EDGE_CURVE ( 'NONE', #12503, #5336, #25995, .T. ) ;
#28657=DIRECTION ( 'NONE',  ( 0.9135454576426004225, -0.4067366430758009854, 0.000000000000000000 ) ) ;
#28658=LINE ( 'NONE', #12621, #24521 ) ;
#28663=VECTOR ( 'NONE', #29679, 1000.000000000000227 ) ;
#28668=CARTESIAN_POINT ( 'NONE',  ( -12.99038105676664934, 15.00000000000012257, 7.000000000000000000 ) ) ;
#28671=LINE ( 'NONE', #16490, #35877 ) ;
#28672=ORIENTED_EDGE ( 'NONE', *, *, #4039, .T. ) ;
#28675=CARTESIAN_POINT ( 'NONE',  ( -14.44482798346716201, 26.50521816028930999, 7.499999999999993783 ) ) ;
#28676=ORIENTED_EDGE ( 'NONE', *, *, #35456, .T. ) ;
#28678=EDGE_CURVE ( 'NONE', #1082, #31776, #13673, .T. ) ;
#28679=CARTESIAN_POINT ( 'NONE',  ( 9.151574469205250750, 1.945227203041362207, 7.000000000000000000 ) ) ;
#28682=CARTESIAN_POINT ( 'NONE',  ( -4.577399223880544099, 35.23960032125098252, 10.00000000000000000 ) ) ;
#28683=AXIS2_PLACEMENT_3D ( 'NONE', #11032, #4727, #16927 ) ;
#28685=ORIENTED_EDGE ( 'NONE', *, *, #37332, .T. ) ;
#28687=ADVANCED_FACE ( 'NONE', ( #9574 ), #13006, .T. ) ;
#28688=DIRECTION ( 'NONE',  ( -0.000000000000000000, -0.000000000000000000, -1.000000000000000000 ) ) ;
#28690=DIRECTION ( 'NONE',  ( 1.000000000000000000, 0.000000000000000000, 0.000000000000000000 ) ) ;
#28691=CIRCLE ( 'NONE', #29341, 0.9999999999999970024 ) ;
#28692=CARTESIAN_POINT ( 'NONE',  ( -10.47804177580193041, 33.28010392086039104, 10.49999999999999822 ) ) ;
#28696=ADVANCED_FACE ( 'NONE', ( #13007 ), #36395, .T. ) ;
#28698=CARTESIAN_POINT ( 'NONE',  ( 13.46929972531963848, 26.35070966310165375, 9.500000000000000000 ) ) ;
#28705=CARTESIAN_POINT ( 'NONE',  ( 10.32110986824234544, 33.06327772184302205, 10.49999999999999822 ) ) ;
#28707=VERTEX_POINT ( 'NONE', #22150 ) ;
#28712=DIRECTION ( 'NONE',  ( -0.000000000000000000, -0.000000000000000000, -1.000000000000000000 ) ) ;
#28714=CARTESIAN_POINT ( 'NONE',  ( 9.151574469205250750, 1.945227203041362207, 11.00000000000000000 ) ) ;
#28726=EDGE_CURVE ( 'NONE', #18134, #15610, #37202, .T. ) ;
#28728=VECTOR ( 'NONE', #6724, 1000.000000000000000 ) ;
#28733=AXIS2_PLACEMENT_3D ( 'NONE', #9273, #22056, #34455 ) ;
#28736=ORIENTED_EDGE ( 'NONE', *, *, #9616, .T. ) ;
#28739=DIRECTION ( 'NONE',  ( 0.9135454576426059736, 0.4067366430757888285, 0.000000000000000000 ) ) ;
#28743=CARTESIAN_POINT ( 'NONE',  ( -14.47283171447380390, 21.48159823030330884, 7.000000000000000000 ) ) ;
#28745=CARTESIAN_POINT ( 'NONE',  ( -12.80736835487441816, 15.68301270189233243, 11.00000000000000000 ) ) ;
#28747=ADVANCED_FACE ( 'NONE', ( #13609 ), #4609, .T. ) ;
#28748=ADVANCED_FACE ( 'NONE', ( #35355 ), #1630, .F. ) ;
#28749=CARTESIAN_POINT ( 'NONE',  ( 8.633502029282041690, 11.46765470489692795, 7.000000000000000000 ) ) ;
#28750=DIRECTION ( 'NONE',  ( 0.9781476007338043566, -0.2079116908177657264, 0.000000000000000000 ) ) ;
#28753=CARTESIAN_POINT ( 'NONE',  ( 13.13294332834914790, 16.07239217250469920, 10.49999999999999645 ) ) ;
#28755=AXIS2_PLACEMENT_3D ( 'NONE', #34649, #3763, #10265 ) ;
#28757=CARTESIAN_POINT ( 'NONE',  ( -11.11016527260153808, 31.83082137946488643, 9.000000000000001776 ) ) ;
#28758=CARTESIAN_POINT ( 'NONE',  ( -13.31203413219588505, 15.58674249317294525, 7.489426592562537621 ) ) ;
#28766=LINE ( 'NONE', #22464, #8846 ) ;
#28771=VECTOR ( 'NONE', #121, 1000.000000000000114 ) ;
#28774=ORIENTED_EDGE ( 'NONE', *, *, #3542, .F. ) ;
#28778=ORIENTED_EDGE ( 'NONE', *, *, #38848, .F. ) ;
#28780=EDGE_CURVE ( 'NONE', #38309, #2164, #33160, .T. ) ;
#28781=VECTOR ( 'NONE', #31454, 999.9999999999998863 ) ;
#28792=PLANE ( 'NONE',  #8702 ) ;
#28795=ORIENTED_EDGE ( 'NONE', *, *, #11640, .T. ) ;
#28796=VECTOR ( 'NONE', #26252, 1000.000000000000114 ) ;
#28801=CARTESIAN_POINT ( 'NONE',  ( 8.315274455032101386, 10.01576150750513250, 7.500000000000000888 ) ) ;
#28802=LINE ( 'NONE', #18867, #28781 ) ;
#28805=DIRECTION ( 'NONE',  ( 1.000000000000000000, 0.000000000000000000, 0.000000000000000000 ) ) ;
#28808=CARTESIAN_POINT ( 'NONE',  ( -19.60875595791377535, 15.93339349895804169, 10.00000000000000000 ) ) ;
#28809=AXIS2_PLACEMENT_3D ( 'NONE', #9220, #27901, #21605 ) ;
#28813=CARTESIAN_POINT ( 'NONE',  ( -8.737320611644010526, -1.152986690174108819, 7.000000000000000000 ) ) ;
#28824=EDGE_LOOP ( 'NONE', ( #9513, #11207, #30281, #27277 ) ) ;
#28826=AXIS2_PLACEMENT_3D ( 'NONE', #4723, #17129, #29505 ) ;
#28827=FACE_OUTER_BOUND ( 'NONE', #2301, .T. ) ;
#28831=CARTESIAN_POINT ( 'NONE',  ( 13.95683075005237050, 28.08631143191933432, 11.00000000000000000 ) ) ;
#28832=ORIENTED_EDGE ( 'NONE', *, *, #12356, .F. ) ;
#28840=CARTESIAN_POINT ( 'NONE',  ( 0.000000000000000000, 22.50000000000000355, 7.000000000000000000 ) ) ;
#28841=DIRECTION ( 'NONE',  ( 0.9781476007338042455, -0.2079116908177664758, 0.000000000000000000 ) ) ;
#28842=LINE ( 'NONE', #1020, #24020 ) ;
#28845=CARTESIAN_POINT ( 'NONE',  ( -11.54200800595901555, 31.54683795827741122, 10.49999999999999645 ) ) ;
#28846=ORIENTED_EDGE ( 'NONE', *, *, #27356, .F. ) ;
#28847=SURFACE_SIDE_STYLE ('',( #16462 ) ) ;
#28848=CARTESIAN_POINT ( 'NONE',  ( 10.44103466624280507, 32.57396620494213124, 7.000000000000000000 ) ) ;
#28849=FACE_OUTER_BOUND ( 'NONE', #32083, .T. ) ;
#28850=CARTESIAN_POINT ( 'NONE',  ( 14.36830325120613594, 20.48707633493483371, 7.000000000000000000 ) ) ;
#28854=CARTESIAN_POINT ( 'NONE',  ( 0.5000000000000035527, 32.50000000000000000, 10.50000000000000178 ) ) ;
#28856=EDGE_CURVE ( 'NONE', #36455, #22772, #20119, .T. ) ;
#28858=DIRECTION ( 'NONE',  ( 1.000000000000000000, 0.000000000000000000, 0.000000000000000000 ) ) ;
#28860=CIRCLE ( 'NONE', #18493, 0.5000000000000004441 ) ;
#28861=ORIENTED_EDGE ( 'NONE', *, *, #8388, .F. ) ;
#28865=EDGE_CURVE ( 'NONE', #12427, #9089, #4868, .T. ) ;
#28866=DIRECTION ( 'NONE',  ( -0.8660254037844364872, 0.5000000000000038858, 0.000000000000000000 ) ) ;
#28869=ORIENTED_EDGE ( 'NONE', *, *, #189, .F. ) ;
#28875=CARTESIAN_POINT ( 'NONE',  ( -10.44103466624267185, 32.57396620494226624, 7.500000000000004441 ) ) ;
#28878=CARTESIAN_POINT ( 'NONE',  ( -6.572794801194226544, 16.58182897866500127, 9.000000000000001776 ) ) ;
#28879=DIRECTION ( 'NONE',  ( 0.5254827454987608393, 0.4731467892558162691, -0.7071067811865451302 ) ) ;
#28880=ORIENTED_EDGE ( 'NONE', *, *, #16466, .T. ) ;
#28887=ADVANCED_FACE ( 'NONE', ( #23155 ), #10568, .T. ) ;
#28888=ORIENTED_EDGE ( 'NONE', *, *, #33705, .F. ) ;
#28890=ADVANCED_FACE ( 'NONE', ( #25997 ), #13202, .T. ) ;
#28892=AXIS2_PLACEMENT_3D ( 'NONE', #18294, #11793, #37171 ) ;
#28894=DIRECTION ( 'NONE',  ( 0.000000000000000000, 0.000000000000000000, -1.000000000000000000 ) ) ;
#28895=DIRECTION ( 'NONE',  ( 0.000000000000000000, 0.000000000000000000, 1.000000000000000000 ) ) ;
#28896=CONICAL_SURFACE ( 'NONE', #2286, 1.000000000000004441, 0.7853981633974583820 ) ;
#28897=VECTOR ( 'NONE', #35045, 1000.000000000000114 ) ;
#28898=AXIS2_PLACEMENT_3D ( 'NONE', #40057, #36426, #24428 ) ;
#28903=PLANE ( 'NONE',  #12469 ) ;
#28904=ADVANCED_FACE ( 'NONE', ( #1027 ), #16876, .F. ) ;
#28909=DIRECTION ( 'NONE',  ( -1.000000000000000000, 0.000000000000000000, 0.000000000000000000 ) ) ;
#28911=ORIENTED_EDGE ( 'NONE', *, *, #21883, .T. ) ;
#28913=DIRECTION ( 'NONE',  ( -0.000000000000000000, -0.000000000000000000, -1.000000000000000000 ) ) ;
#28914=ORIENTED_EDGE ( 'NONE', *, *, #14335, .F. ) ;
#28916=FACE_OUTER_BOUND ( 'NONE', #16149, .T. ) ;
#28922=CARTESIAN_POINT ( 'NONE',  ( -4.984135866956331817, 36.15314577889358105, 10.50000000000000533 ) ) ;
#28926=PLANE ( 'NONE',  #4425 ) ;
#28927=DIRECTION ( 'NONE',  ( 0.9135454576426048634, 0.4067366430757912710, -6.938893903907218911E-15 ) ) ;
#28928=ORIENTED_EDGE ( 'NONE', *, *, #23415, .F. ) ;
#28934=ORIENTED_EDGE ( 'NONE', *, *, #28099, .F. ) ;
#28937=CARTESIAN_POINT ( 'NONE',  ( -13.94482798346716557, 26.50521816028930289, 11.00000000000000000 ) ) ;
#28938=CARTESIAN_POINT ( 'NONE',  ( 13.63396663385386454, 16.24580510161703728, 7.000000000000000000 ) ) ;
#28940=PLANE ( 'NONE',  #660 ) ;
#28941=CARTESIAN_POINT ( 'NONE',  ( -14.42035624161473883, 26.65972665747678860, 10.49999999999999822 ) ) ;
#28942=B_SPLINE_CURVE_WITH_KNOTS ( 'NONE', 3,
 ( #467, #37241, #3508, #21994, #9411, #3112, #3308, #18755 ),
 .UNSPECIFIED., .F., .F.,
 ( 4, 2, 2, 4 ),
 ( 0.000000000000000000, 0.0004488403289517302135, 0.0006732604934275947511, 0.0008976806579034594512 ),
 .UNSPECIFIED. ) ;
#28943=CARTESIAN_POINT ( 'NONE',  ( -14.57486473880221745, 26.18419839932921533, 10.50000000000000533 ) ) ;
#28944=ORIENTED_EDGE ( 'NONE', *, *, #39336, .F. ) ;
#28945=CARTESIAN_POINT ( 'NONE',  ( -6.392125613574828336, 35.62765252371742264, 10.99387789255782799 ) ) ;
#28946=CARTESIAN_POINT ( 'NONE',  ( -6.994507294956786581, 44.66003774390582493, 9.500000000000000000 ) ) ;
#28949=PLANE ( 'NONE',  #1515 ) ;
#28950=EDGE_CURVE ( 'NONE', #31599, #7885, #32102, .T. ) ;
#28952=DIRECTION ( 'NONE',  ( -0.9135454576426005335, 0.4067366430758009299, 0.000000000000000000 ) ) ;
#28953=ORIENTED_EDGE ( 'NONE', *, *, #37807, .T. ) ;
#28955=VECTOR ( 'NONE', #9641, 1000.000000000000000 ) ;
#28957=EDGE_CURVE ( 'NONE', #39268, #16887, #1426, .T. ) ;
#28961=CARTESIAN_POINT ( 'NONE',  ( 2.525645716490518389, 8.212903943950921715, 9.000000000000001776 ) ) ;
#28963=ORIENTED_EDGE ( 'NONE', *, *, #23233, .T. ) ;
#28965=VERTEX_POINT ( 'NONE', #11377 ) ;
#28970=EDGE_CURVE ( 'NONE', #37730, #9704, #24156, .T. ) ;
#28974=EDGE_LOOP ( 'NONE', ( #14636, #12450, #11148, #4189 ) ) ;
#28976=LINE ( 'NONE', #38321, #27743 ) ;
#28979=ORIENTED_EDGE ( 'NONE', *, *, #3169, .T. ) ;
#28981=DIRECTION ( 'NONE',  ( 0.3090169943749560000, 0.9510565162951507556, 0.000000000000000000 ) ) ;
#28982=ORIENTED_EDGE ( 'NONE', *, *, #12986, .T. ) ;
#28983=LINE ( 'NONE', #9899, #38090 ) ;
#28984=FACE_OUTER_BOUND ( 'NONE', #9260, .T. ) ;
#28985=EDGE_CURVE ( 'NONE', #31336, #22260, #8521, .T. ) ;
#28986=ADVANCED_FACE ( 'NONE', ( #15014 ), #15626, .T. ) ;
#28988=EDGE_CURVE ( 'NONE', #30940, #3918, #27943, .T. ) ;
#28991=ORIENTED_EDGE ( 'NONE', *, *, #16962, .F. ) ;
#28992=ORIENTED_EDGE ( 'NONE', *, *, #8046, .F. ) ;
#28999=FACE_OUTER_BOUND ( 'NONE', #25966, .T. ) ;
#29002=EDGE_CURVE ( 'NONE', #1935, #7593, #16290, .T. ) ;
#29003=CARTESIAN_POINT ( 'NONE',  ( 9.221287281574507944, 10.65863771052197784, 10.49999999999999822 ) ) ;
#29005=EDGE_CURVE ( 'NONE', #36981, #10090, #18076, .T. ) ;
#29006=DIRECTION ( 'NONE',  ( -2.168404344971006896E-16, 1.000000000000000000, 0.000000000000000000 ) ) ;
#29009=CARTESIAN_POINT ( 'NONE',  ( 4.984135866956515670, 36.15314577889351000, 11.00000000000000000 ) ) ;
#29010=DIRECTION ( 'NONE',  ( -0.7431448254773953543, -0.6691306063588570163, -0.000000000000000000 ) ) ;
#29011=EDGE_CURVE ( 'NONE', #14195, #10996, #20728, .T. ) ;
#29013=FACE_OUTER_BOUND ( 'NONE', #15289, .T. ) ;
#29017=CIRCLE ( 'NONE', #28374, 0.5000000000000011102 ) ;
#29018=CIRCLE ( 'NONE', #29658, 1.000000000000007772 ) ;
#29019=ADVANCED_FACE ( 'NONE', ( #33522 ), #8520, .T. ) ;
#29024=DIRECTION ( 'NONE',  ( 0.8386705679454296014, 0.5446390350150185355, -9.740544695154170490E-16 ) ) ;
#29026=VERTEX_POINT ( 'NONE', #23759 ) ;
#29029=VECTOR ( 'NONE', #32206, 999.9999999999998863 ) ;
#29030=CARTESIAN_POINT ( 'NONE',  ( 14.70981814587860903, 21.45668995266196433, 10.94387467463493557 ) ) ;
#29031=ORIENTED_EDGE ( 'NONE', *, *, #39241, .F. ) ;
#29033=CARTESIAN_POINT ( 'NONE',  ( 8.412270287199559604, 10.07085245822950981, 11.00000000000000000 ) ) ;
#29035=ORIENTED_EDGE ( 'NONE', *, *, #33018, .T. ) ;
#29039=ADVANCED_FACE ( 'NONE', ( #17482 ), #8924, .F. ) ;
#29040=VERTEX_POINT ( 'NONE', #26605 ) ;
#29042=CARTESIAN_POINT ( 'NONE',  ( -6.151085731882353969, 35.08626808545859888, 7.000000000000000000 ) ) ;
#29043=CARTESIAN_POINT ( 'NONE',  ( -4.059628295990764357, 8.059656032623825794, 7.338691926023208190 ) ) ;
#29046=FACE_OUTER_BOUND ( 'NONE', #31078, .T. ) ;
#29049=CARTESIAN_POINT ( 'NONE',  ( 12.80736835487433289, 15.68301270189216545, 11.00000000000000000 ) ) ;
#29051=CIRCLE ( 'NONE', #11551, 15.00000000000000000 ) ;
#29054=AXIS2_PLACEMENT_3D ( 'NONE', #20146, #31379, #23390 ) ;
#29056=ORIENTED_EDGE ( 'NONE', *, *, #27545, .T. ) ;
#29058=CARTESIAN_POINT ( 'NONE',  ( -1.000000000000000222, 37.13089969389957901, 10.49999999999999645 ) ) ;
#29061=PLANE ( 'NONE',  #35303 ) ;
#29062=CARTESIAN_POINT ( 'NONE',  ( -14.36830325120616081, 20.48707633493503977, 11.00000000000000000 ) ) ;
#29067=DIRECTION ( 'NONE',  ( -2.168404344971006896E-16, 1.000000000000000000, 0.000000000000000000 ) ) ;
#29068=VERTEX_POINT ( 'NONE', #14820 ) ;
#29069=VERTEX_POINT ( 'NONE', #26807 ) ;
#29071=FACE_OUTER_BOUND ( 'NONE', #16953, .T. ) ;
#29073=AXIS2_PLACEMENT_3D ( 'NONE', #34090, #34290, #14999 ) ;
#29076=CARTESIAN_POINT ( 'NONE',  ( -13.36146265112639675, 15.68301270189280672, 7.445905703748357141 ) ) ;
#29077=ORIENTED_EDGE ( 'NONE', *, *, #27736, .F. ) ;
#29080=CARTESIAN_POINT ( 'NONE',  ( 13.53057405073934838, 22.08338764125490528, 9.500000000000000000 ) ) ;
#29084=CARTESIAN_POINT ( 'NONE',  ( -5.002948306803596701, 36.19539921059739385, 10.49999999999999822 ) ) ;
#29085=ORIENTED_EDGE ( 'NONE', *, *, #16640, .F. ) ;
#29087=VECTOR ( 'NONE', #38174, 999.9999999999998863 ) ;
#29090=EDGE_CURVE ( 'NONE', #23552, #28064, #27011, .T. ) ;
#29091=VERTEX_POINT ( 'NONE', #14622 ) ;
#29093=ADVANCED_FACE ( 'NONE', ( #15218 ), #31229, .T. ) ;
#29095=CARTESIAN_POINT ( 'NONE',  ( -0.9999999999999997780, 36.00000000000000711, 9.500000000000000000 ) ) ;
#29098=CARTESIAN_POINT ( 'NONE',  ( 2.806807826039672715, 9.295007390093600108, 7.000000000000000000 ) ) ;
#29099=EDGE_CURVE ( 'NONE', #20131, #33341, #18471, .T. ) ;
#29106=CIRCLE ( 'NONE', #8989, 0.5000000000000004441 ) ;
#29107=DIRECTION ( 'NONE',  ( -0.2079116908177663647, -0.9781476007338042455, -3.469446951953611033E-15 ) ) ;
#29108=EDGE_LOOP ( 'NONE', ( #11665, #30533, #10436 ) ) ;
#29113=EDGE_CURVE ( 'NONE', #13649, #11592, #6266, .T. ) ;
#29114=CARTESIAN_POINT ( 'NONE',  ( 10.58109189495872116, 32.70007430011108340, 10.96580508970282963 ) ) ;
#29116=ORIENTED_EDGE ( 'NONE', *, *, #23922, .T. ) ;
#29119=ORIENTED_EDGE ( 'NONE', *, *, #12986, .F. ) ;
#29121=CARTESIAN_POINT ( 'NONE',  ( 8.249810963174727618, 9.972158775796183150, 7.485699520496982728 ) ) ;
#29123=CARTESIAN_POINT ( 'NONE',  ( -9.356056665764020508, 26.06569820189716324, 10.50000000000000533 ) ) ;
#29124=EDGE_LOOP ( 'NONE', ( #33069, #37909, #36393, #26593, #20438, #38124, #5404 ) ) ;
#29127=PLANE ( 'NONE',  #6647 ) ;
#29129=ORIENTED_EDGE ( 'NONE', *, *, #39045, .T. ) ;
#29133=EDGE_LOOP ( 'NONE', ( #5261, #1788, #25875 ) ) ;
#29135=AXIS2_PLACEMENT_3D ( 'NONE', #27459, #29911, #33775 ) ;
#29137=AXIS2_PLACEMENT_3D ( 'NONE', #15373, #15769, #27960 ) ;
#29139=ADVANCED_FACE ( 'NONE', ( #21901 ), #33819, .T. ) ;
#29141=AXIS2_PLACEMENT_3D ( 'NONE', #13247, #19961, #28690 ) ;
#29146=PLANE ( 'NONE',  #19356 ) ;
#29147=EDGE_CURVE ( 'NONE', #39240, #4057, #65, .T. ) ;
#29150=CARTESIAN_POINT ( 'NONE',  ( -11.48173768534023331, 32.16538668264431777, 10.49999999999999822 ) ) ;
#29151=LINE ( 'NONE', #19198, #3457 ) ;
#29152=DIRECTION ( 'NONE',  ( 0.000000000000000000, 0.000000000000000000, -1.000000000000000000 ) ) ;
#29153=ORIENTED_EDGE ( 'NONE', *, *, #39173, .T. ) ;
#29155=PLANE ( 'NONE',  #22023 ) ;
#29157=DIRECTION ( 'NONE',  ( -1.000000000000000000, 0.000000000000000000, 0.000000000000000000 ) ) ;
#29158=CARTESIAN_POINT ( 'NONE',  ( -7.096882951594429834, 29.56287847632736288, 10.49999999999999645 ) ) ;
#29160=CARTESIAN_POINT ( 'NONE',  ( 0.4999999999999995559, 37.00000000000000711, 11.00000000000000000 ) ) ;
#29161=AXIS2_PLACEMENT_3D ( 'NONE', #32819, #22847, #32618 ) ;
#29162=ORIENTED_EDGE ( 'NONE', *, *, #30308, .T. ) ;
#29167=EDGE_CURVE ( 'NONE', #11008, #5904, #21706, .T. ) ;
#29172=AXIS2_PLACEMENT_3D ( 'NONE', #26802, #20315, #5465 ) ;
#29173=B_SPLINE_SURFACE_WITH_KNOTS ( 'NONE', 1, 3, ( 
 ( #31964, #690, #16331, #13067, #38060, #9644, #22411, #22022, #4130, #31368 ),
 ( #37267, #9441, #28314, #34813, #6966, #21820, #19371, #34225, #7582, #5145 ) ),
 .UNSPECIFIED., .F., .F., .F.,
 ( 2, 2 ),
 ( 4, 2, 2, 2, 4 ),
 ( 0.000000000000000000, 1.000000000000000000 ),
 ( 1.958393013450087983, 2.351092095148810568, 2.743791176847532931, 3.136490258546255738, 3.529189340244978101 ),
 .UNSPECIFIED. ) ;
#29176=CARTESIAN_POINT ( 'NONE',  ( -13.94482798346716201, 26.50521816028930999, 7.499999999999993783 ) ) ;
#29182=EDGE_LOOP ( 'NONE', ( #6223, #5267, #28992, #17203 ) ) ;
#29184=DIRECTION ( 'NONE',  ( -0.000000000000000000, -0.000000000000000000, 1.000000000000000000 ) ) ;
#29185=CARTESIAN_POINT ( 'NONE',  ( -12.23327497914565853, 13.81973598992469121, 7.000000000000000000 ) ) ;
#29190=EDGE_LOOP ( 'NONE', ( #8712, #16657, #23245, #7977, #3133 ) ) ;
#29191=CARTESIAN_POINT ( 'NONE',  ( 8.137585970692075676, 29.15429895402930072, 10.50000000000000000 ) ) ;
#29192=DIRECTION ( 'NONE',  ( 1.000000000000000000, 0.000000000000000000, 0.000000000000000000 ) ) ;
#29193=EDGE_CURVE ( 'NONE', #3260, #34846, #37351, .T. ) ;
#29196=VECTOR ( 'NONE', #7111, 1000.000000000000000 ) ;
#29198=CIRCLE ( 'NONE', #12317, 0.5000000000000004441 ) ;
#29199=FACE_OUTER_BOUND ( 'NONE', #32461, .T. ) ;
#29202=VERTEX_POINT ( 'NONE', #16014 ) ;
#29205=CARTESIAN_POINT ( 'NONE',  ( -13.63581098909220479, 27.45627467658446008, 7.000000000000000000 ) ) ;
#29206=DIRECTION ( 'NONE',  ( -0.000000000000000000, -0.000000000000000000, -1.000000000000000000 ) ) ;
#29207=CARTESIAN_POINT ( 'NONE',  ( -14.50767453556301589, 21.81310552875940090, 10.66666666666666252 ) ) ;
#29208=LINE ( 'NONE', #38347, #39162 ) ;
#29210=DIRECTION ( 'NONE',  ( -1.000000000000000000, 0.000000000000000000, 0.000000000000000000 ) ) ;
#29211=VERTEX_POINT ( 'NONE', #18865 ) ;
#29212=AXIS2_PLACEMENT_3D ( 'NONE', #1623, #7710, #4054 ) ;
#29215=CARTESIAN_POINT ( 'NONE',  ( -14.08493436138092036, 27.60220370627969899, 10.68306085400105765 ) ) ;
#29220=CARTESIAN_POINT ( 'NONE',  ( -8.505700342264141511, 22.10876900990917804, 7.000000000000000000 ) ) ;
#29221=EDGE_CURVE ( 'NONE', #7567, #4300, #9919, .T. ) ;
#29226=CARTESIAN_POINT ( 'NONE',  ( -8.744117900323425729, 12.16605582823075338, 10.00000000000000000 ) ) ;
#29228=ORIENTED_EDGE ( 'NONE', *, *, #27501, .T. ) ;
#29230=EDGE_LOOP ( 'NONE', ( #3213, #13096, #5727, #29680 ) ) ;
#29232=CARTESIAN_POINT ( 'NONE',  ( 14.75621568350166335, 21.89813303538585032, 10.49999999999999822 ) ) ;
#29233=ORIENTED_EDGE ( 'NONE', *, *, #30488, .F. ) ;
#29237=ORIENTED_EDGE ( 'NONE', *, *, #33173, .F. ) ;
#29239=EDGE_CURVE ( 'NONE', #25837, #31884, #24098, .T. ) ;
#29240=ORIENTED_EDGE ( 'NONE', *, *, #25395, .T. ) ;
#29241=B_SPLINE_CURVE_WITH_KNOTS ( 'NONE', 3,
 ( #21104, #20906, #11760, #23353, #23750, #11366, #35750, #1823 ),
 .UNSPECIFIED., .F., .F.,
 ( 4, 2, 2, 4 ),
 ( 8.673617379884035472E-19, 0.0004726692273637059846, 0.0007090038410455666747, 0.0009453384547274274732 ),
 .UNSPECIFIED. ) ;
#29243=ADVANCED_FACE ( 'NONE', ( #22298 ), #21508, .F. ) ;
#29244=CIRCLE ( 'NONE', #4599, 0.5000000000000004441 ) ;
#29250=ADVANCED_FACE ( 'NONE', ( #3024 ), #27808, .F. ) ;
#29255=AXIS2_PLACEMENT_3D ( 'NONE', #28649, #15664, #18912 ) ;
#29256=DIRECTION ( 'NONE',  ( 0.000000000000000000, 0.000000000000000000, 1.000000000000000000 ) ) ;
#29263=DIRECTION ( 'NONE',  ( 0.8090169943749510040, 0.5877852522924683631, 0.000000000000000000 ) ) ;
#29264=EDGE_CURVE ( 'NONE', #39078, #36470, #3226, .T. ) ;
#29265=CYLINDRICAL_SURFACE ( 'NONE', #38648, 0.5000000000000004441 ) ;
#29266=EDGE_CURVE ( 'NONE', #12503, #15556, #28003, .T. ) ;
#29267=ORIENTED_EDGE ( 'NONE', *, *, #31190, .F. ) ;
#29269=CONICAL_SURFACE ( 'NONE', #24082, 0.9999999999999983347, 0.7853981633974498333 ) ;
#29273=FACE_OUTER_BOUND ( 'NONE', #10979, .T. ) ;
#29274=ORIENTED_EDGE ( 'NONE', *, *, #15871, .T. ) ;
#29275=ORIENTED_EDGE ( 'NONE', *, *, #13596, .T. ) ;
#29277=CYLINDRICAL_SURFACE ( 'NONE', #5512, 6.000000000000003553 ) ;
#29281=VERTEX_POINT ( 'NONE', #15814 ) ;
#29283=CARTESIAN_POINT ( 'NONE',  ( 13.37378135583786332, 20.59160479820249634, 9.500000000000000000 ) ) ;
#29286=ORIENTED_EDGE ( 'NONE', *, *, #10914, .T. ) ;
#29288=CARTESIAN_POINT ( 'NONE',  ( -5.027400250555931649, 36.23526740290156312, 10.49999999999999822 ) ) ;
#29295=ORIENTED_EDGE ( 'NONE', *, *, #23538, .T. ) ;
#29298=CARTESIAN_POINT ( 'NONE',  ( 13.94482798346721353, 26.50521816028912525, 11.00000000000000000 ) ) ;
#29300=AXIS2_PLACEMENT_3D ( 'NONE', #10769, #19708, #29652 ) ;
#29301=FACE_OUTER_BOUND ( 'NONE', #10669, .T. ) ;
#29302=AXIS2_PLACEMENT_3D ( 'NONE', #31296, #16051, #3461 ) ;
#29308=VECTOR ( 'NONE', #4496, 1000.000000000000227 ) ;
#29310=DIRECTION ( 'NONE',  ( 0.1045284632676570929, 0.9945218953682729568, 0.000000000000000000 ) ) ;
#29311=CARTESIAN_POINT ( 'NONE',  ( -13.28731253931435319, 15.83618351362805043, 10.49999999999999822 ) ) ;
#29312=ORIENTED_EDGE ( 'NONE', *, *, #7321, .T. ) ;
#29317=CARTESIAN_POINT ( 'NONE',  ( 4.475131784526629630, 8.183115020678576101, 7.000000000000000000 ) ) ;
#29321=EDGE_CURVE ( 'NONE', #24512, #17938, #22697, .T. ) ;
#29324=PLANE ( 'NONE',  #14054 ) ;
#29326=DIRECTION ( 'NONE',  ( 0.000000000000000000, 0.000000000000000000, -1.000000000000000000 ) ) ;
#29327=ORIENTED_EDGE ( 'NONE', *, *, #35101, .T. ) ;
#29334=CARTESIAN_POINT ( 'NONE',  ( 11.54666566735224364, 32.07468077621332725, 7.499999999999997335 ) ) ;
#29336=EDGE_LOOP ( 'NONE', ( #11637, #14239, #3478, #15072 ) ) ;
#29341=AXIS2_PLACEMENT_3D ( 'NONE', #7695, #1403, #38372 ) ;
#29344=LINE ( 'NONE', #38078, #491 ) ;
#29345=DIRECTION ( 'NONE',  ( -0.5877852522924791323, -0.8090169943749430104, 6.938893903907231533E-15 ) ) ;
#29349=ORIENTED_EDGE ( 'NONE', *, *, #4912, .T. ) ;
#29350=LINE ( 'NONE', #13097, #7839 ) ;
#29351=CARTESIAN_POINT ( 'NONE',  ( -6.654030453887870067, 35.94335816374513115, 7.000000000000000000 ) ) ;
#29353=FACE_OUTER_BOUND ( 'NONE', #9822, .T. ) ;
#29356=DIRECTION ( 'NONE',  ( 1.000000000000000000, 0.000000000000000000, -0.000000000000000000 ) ) ;
#29363=FACE_OUTER_BOUND ( 'NONE', #19407, .T. ) ;
#29365=ORIENTED_EDGE ( 'NONE', *, *, #11344, .F. ) ;
#29369=CARTESIAN_POINT ( 'NONE',  ( 14.42035624161478857, 26.65972665747657899, 10.59344459855564580 ) ) ;
#29372=VECTOR ( 'NONE', #38877, 1000.000000000000000 ) ;
#29379=DIRECTION ( 'NONE',  ( 0.000000000000000000, 0.000000000000000000, 1.000000000000000000 ) ) ;
#29381=ADVANCED_FACE ( 'NONE', ( #13357 ), #20070, .F. ) ;
#29383=ORIENTED_EDGE ( 'NONE', *, *, #24147, .F. ) ;
#29386=ORIENTED_EDGE ( 'NONE', *, *, #12593, .T. ) ;
#29388=CARTESIAN_POINT ( 'NONE',  ( 8.505700342264139735, 22.10876900990906435, 9.000000000000001776 ) ) ;
#29395=ADVANCED_FACE ( 'NONE', ( #771 ), #19452, .T. ) ;
#29397=CARTESIAN_POINT ( 'NONE',  ( -0.5000000000000007772, 32.75000000000000000, 10.75000000000000000 ) ) ;
#29402=CARTESIAN_POINT ( 'NONE',  ( -14.99771756515323418, 22.21226231334756562, 7.102474990965861323 ) ) ;
#29403=FACE_OUTER_BOUND ( 'NONE', #26543, .T. ) ;
#29405=DIRECTION ( 'NONE',  ( 0.000000000000000000, 0.000000000000000000, -1.000000000000000000 ) ) ;
#29406=CIRCLE ( 'NONE', #32671, 0.4999999999999989453 ) ;
#29407=DIRECTION ( 'NONE',  ( 1.000000000000000000, -3.469446951953598806E-15, 0.000000000000000000 ) ) ;
#29409=CARTESIAN_POINT ( 'NONE',  ( -12.42073081513906985, 14.75153745115810722, 10.99999999999999822 ) ) ;
#29412=DIRECTION ( 'NONE',  ( 1.000000000000000000, -1.387778780781449147E-14, 0.000000000000000000 ) ) ;
#29413=AXIS2_PLACEMENT_3D ( 'NONE', #37692, #35245, #19395 ) ;
#29414=CARTESIAN_POINT ( 'NONE',  ( -13.84312823610348708, 27.91543399189774632, 10.49999999999999822 ) ) ;
#29416=CARTESIAN_POINT ( 'NONE',  ( -12.74038105676665289, 14.56698729810790027, 10.49999999999999822 ) ) ;
#29421=VECTOR ( 'NONE', #11317, 1000.000000000000000 ) ;
#29426=DIRECTION ( 'NONE',  ( -0.000000000000000000, -0.000000000000000000, -1.000000000000000000 ) ) ;
#29427=ORIENTED_EDGE ( 'NONE', *, *, #5515, .F. ) ;
#29429=ORIENTED_EDGE ( 'NONE', *, *, #11364, .T. ) ;
#29430=DIRECTION ( 'NONE',  ( 0.9945218953682731788, -0.1045284632676559550, 0.000000000000000000 ) ) ;
#29431=EDGE_LOOP ( 'NONE', ( #1491, #22470, #9402, #11456 ) ) ;
#29432=LINE ( 'NONE', #16857, #14156 ) ;
#29433=CARTESIAN_POINT ( 'NONE',  ( -9.902837789212762587, 25.19189593419573114, 10.74999999999999822 ) ) ;
#29436=ORIENTED_EDGE ( 'NONE', *, *, #20581, .F. ) ;
#29438=VECTOR ( 'NONE', #521, 1000.000000000000000 ) ;
#29439=ORIENTED_EDGE ( 'NONE', *, *, #22556, .T. ) ;
#29441=CARTESIAN_POINT ( 'NONE',  ( -3.607749162633401507, 7.931741834401821123, 10.49999999999999822 ) ) ;
#29442=VERTEX_POINT ( 'NONE', #16412 ) ;
#29444=CARTESIAN_POINT ( 'NONE',  ( 11.30736835487432224, 14.81698729810772619, 7.000000000000000000 ) ) ;
#29445=CARTESIAN_POINT ( 'NONE',  ( -3.713592597587352717, 7.966960743906856379, 7.499999999999997335 ) ) ;
#29447=CARTESIAN_POINT ( 'NONE',  ( 13.63581098909226519, 27.45627467658428600, 7.000000000000000000 ) ) ;
#29454=AXIS2_PLACEMENT_3D ( 'NONE', #16404, #23305, #14159 ) ;
#29455=EDGE_LOOP ( 'NONE', ( #38726, #23188, #22887, #7924, #36085 ) ) ;
#29457=DIRECTION ( 'NONE',  ( 1.000000000000000000, 0.000000000000000000, -0.000000000000000000 ) ) ;
#29460=CARTESIAN_POINT ( 'NONE',  ( 8.137585970692077453, 29.15429895402930072, 10.50000000000000000 ) ) ;
#29467=ADVANCED_FACE ( 'NONE', ( #19868 ), #38142, .T. ) ;
#29468=EDGE_CURVE ( 'NONE', #32234, #29912, #31650, .T. ) ;
#29469=CARTESIAN_POINT ( 'NONE',  ( -13.05736835487441994, 16.11602540378456183, 11.00000000000000000 ) ) ;
#29470=EDGE_LOOP ( 'NONE', ( #34346, #19235, #6951, #8605 ) ) ;
#29473=FACE_OUTER_BOUND ( 'NONE', #22268, .T. ) ;
#29475=AXIS2_PLACEMENT_3D ( 'NONE', #20778, #8572, #35610 ) ;
#29478=CARTESIAN_POINT ( 'NONE',  ( 8.368303251206119953, 20.48707633493483371, 7.000000000000000000 ) ) ;
#29479=ORIENTED_EDGE ( 'NONE', *, *, #33257, .T. ) ;
#29481=DIRECTION ( 'NONE',  ( 0.000000000000000000, 0.000000000000000000, 1.000000000000000000 ) ) ;
#29482=CARTESIAN_POINT ( 'NONE',  ( -8.410254037844433483, 17.06698729810786475, 10.50000000000000000 ) ) ;
#29483=DIRECTION ( 'NONE',  ( -0.8090169943749426773, 0.5877852522924796874, 0.000000000000000000 ) ) ;
#29485=ORIENTED_EDGE ( 'NONE', *, *, #27694, .F. ) ;
#29487=DIRECTION ( 'NONE',  ( -0.9135454576426031981, 0.4067366430757951568, 0.000000000000000000 ) ) ;
#29488=EDGE_LOOP ( 'NONE', ( #35082, #27512, #26054, #37057 ) ) ;
#29490=AXIS2_PLACEMENT_3D ( 'NONE', #29049, #17072, #14212 ) ;
#29496=ADVANCED_FACE ( 'NONE', ( #1176 ), #25946, .F. ) ;
#29497=DIRECTION ( 'NONE',  ( 0.000000000000000000, 0.000000000000000000, 1.000000000000000000 ) ) ;
#29498=EDGE_CURVE ( 'NONE', #28465, #13835, #7459, .T. ) ;
#29500=CARTESIAN_POINT ( 'NONE',  ( 14.52509594610762278, 21.97885917798724620, 9.500000000000000000 ) ) ;
#29502=DIRECTION ( 'NONE',  ( 1.000000000000000000, 0.000000000000000000, 0.000000000000000000 ) ) ;
#29505=DIRECTION ( 'NONE',  ( -0.9135454576425986462, 0.4067366430758054263, 0.000000000000000000 ) ) ;
#29509=CONICAL_SURFACE ( 'NONE', #39883, 0.5000000000000039968, 0.7853981633974480570 ) ;
#29510=CARTESIAN_POINT ( 'NONE',  ( -13.24038105676665111, 15.43301270189234486, 10.49999999999999822 ) ) ;
#29511=DIRECTION ( 'NONE',  ( 0.8660254037844431485, 0.4999999999999921174, -0.000000000000000000 ) ) ;
#29513=EDGE_CURVE ( 'NONE', #23354, #20669, #30580, .T. ) ;
#29518=EDGE_CURVE ( 'NONE', #32217, #18134, #13759, .T. ) ;
#29521=ORIENTED_EDGE ( 'NONE', *, *, #17182, .T. ) ;
#29523=ORIENTED_EDGE ( 'NONE', *, *, #30760, .T. ) ;
#29525=CARTESIAN_POINT ( 'NONE',  ( 4.940908595777814938, 35.94977745735560859, 9.500000000000000000 ) ) ;
#29527=LINE ( 'NONE', #1702, #32213 ) ;
#29528=ORIENTED_EDGE ( 'NONE', *, *, #12015, .T. ) ;
#29531=CARTESIAN_POINT ( 'NONE',  ( -2.140527761532693418, 7.619874298175171035, 10.50000000000000355 ) ) ;
#29533=ORIENTED_EDGE ( 'NONE', *, *, #5690, .F. ) ;
#29537=ORIENTED_EDGE ( 'NONE', *, *, #2415, .T. ) ;
#29539=VECTOR ( 'NONE', #35111, 1000.000000000000000 ) ;
#29542=ORIENTED_EDGE ( 'NONE', *, *, #40176, .T. ) ;
#29544=AXIS2_PLACEMENT_3D ( 'NONE', #15127, #27516, #31164 ) ;
#29546=CARTESIAN_POINT ( 'NONE',  ( 7.824485034907088021, 10.87986945260446170, 10.00000000000000000 ) ) ;
#29547=VECTOR ( 'NONE', #39092, 1000.000000000000000 ) ;
#29548=AXIS2_PLACEMENT_3D ( 'NONE', #33345, #36180, #11794 ) ;
#29551=CARTESIAN_POINT ( 'NONE',  ( 13.63581098909226874, 27.45627467658428955, 7.000000000000000000 ) ) ;
#29552=CARTESIAN_POINT ( 'NONE',  ( 8.007761790012084546, 9.776959832083274904, 10.49999999999999822 ) ) ;
#29555=DIRECTION ( 'NONE',  ( 0.8660254037844363761, -0.5000000000000039968, -0.000000000000000000 ) ) ;
#29559=CARTESIAN_POINT ( 'NONE',  ( -14.86556419889030067, 20.43481210330121556, 10.49999999999999822 ) ) ;
#29568=ORIENTED_EDGE ( 'NONE', *, *, #23072, .F. ) ;
#29570=EDGE_LOOP ( 'NONE', ( #35688, #18635, #33504, #31680 ) ) ;
#29572=LINE ( 'NONE', #33242, #25704 ) ;
#29580=ORIENTED_EDGE ( 'NONE', *, *, #15807, .T. ) ;
#29584=DIRECTION ( 'NONE',  ( -0.5877852522924796874, -0.8090169943749426773, 0.000000000000000000 ) ) ;
#29589=DIRECTION ( 'NONE',  ( -1.000000000000000000, 0.000000000000000000, 0.000000000000000000 ) ) ;
#29590=PLANE ( 'NONE',  #5412 ) ;
#29592=DIRECTION ( 'NONE',  ( 0.6691306063588560171, -0.7431448254773962425, 0.000000000000000000 ) ) ;
#29593=EDGE_CURVE ( 'NONE', #31884, #26227, #26416, .T. ) ;
#29594=ORIENTED_EDGE ( 'NONE', *, *, #33758, .T. ) ;
#29598=CARTESIAN_POINT ( 'NONE',  ( 6.373266493267778721, 35.58529424598359725, 11.00000000000000000 ) ) ;
#29602=DIRECTION ( 'NONE',  ( -0.000000000000000000, -0.000000000000000000, -1.000000000000000000 ) ) ;
#29604=DIRECTION ( 'NONE',  ( -0.000000000000000000, -0.000000000000000000, -1.000000000000000000 ) ) ;
#29605=EDGE_CURVE ( 'NONE', #35208, #32427, #5651, .T. ) ;
#29607=CARTESIAN_POINT ( 'NONE',  ( 12.69371393710733642, 14.59393057220526835, 10.76099332938164288 ) ) ;
#29608=DIRECTION ( 'NONE',  ( 1.000000000000000000, 0.000000000000000000, 0.000000000000000000 ) ) ;
#29611=VERTEX_POINT ( 'NONE', #20678 ) ;
#29616=CARTESIAN_POINT ( 'NONE',  ( -13.76030399595643239, 27.49672490655791535, 11.00000000000000000 ) ) ;
#29620=FACE_OUTER_BOUND ( 'NONE', #25444, .T. ) ;
#29626=EDGE_CURVE ( 'NONE', #7910, #27538, #17834, .T. ) ;
#29627=ORIENTED_EDGE ( 'NONE', *, *, #38183, .T. ) ;
#29629=ORIENTED_EDGE ( 'NONE', *, *, #35571, .T. ) ;
#29631=CONICAL_SURFACE ( 'NONE', #34815, 1.000000000000004441, 0.7853981633974482790 ) ;
#29632=DIRECTION ( 'NONE',  ( -0.9781476007338067991, -0.2079116908177533474, 0.000000000000000000 ) ) ;
#29633=VERTEX_POINT ( 'NONE', #30010 ) ;
#29634=PLANE ( 'NONE',  #2506 ) ;
#29635=CARTESIAN_POINT ( 'NONE',  ( 9.381390373406876648, 11.27850996657544513, 10.49999999999999822 ) ) ;
#29636=VERTEX_POINT ( 'NONE', #33075 ) ;
#29640=ORIENTED_EDGE ( 'NONE', *, *, #36427, .T. ) ;
#29642=CARTESIAN_POINT ( 'NONE',  ( -10.14060191828654212, 25.26915018278947755, 10.00000000000000000 ) ) ;
#29643=ORIENTED_EDGE ( 'NONE', *, *, #3911, .T. ) ;
#29644=DIRECTION ( 'NONE',  ( -0.9135454576426005335, 0.4067366430758010409, 0.000000000000000000 ) ) ;
#29646=EDGE_CURVE ( 'NONE', #21311, #38258, #35907, .T. ) ;
#29649=ORIENTED_EDGE ( 'NONE', *, *, #19664, .T. ) ;
#29650=SHAPE_REPRESENTATION_RELATIONSHIP ( 'NONE' , 'NONE' ,  #28068, #36190 ) ;
#29651=CARTESIAN_POINT ( 'NONE',  ( 9.941034666242806850, 32.57396620494213124, 7.499999999999997335 ) ) ;
#29652=DIRECTION ( 'NONE',  ( -0.9510565162951503115, 0.3090169943749572767, 0.000000000000000000 ) ) ;
#29653=EDGE_CURVE ( 'NONE', #34264, #23249, #10207, .T. ) ;
#29654=DIRECTION ( 'NONE',  ( -1.000000000000000000, 0.000000000000000000, 0.000000000000000000 ) ) ;
#29656=VECTOR ( 'NONE', #25180, 1000.000000000000227 ) ;
#29658=AXIS2_PLACEMENT_3D ( 'NONE', #15990, #18643, #37127 ) ;
#29659=VERTEX_POINT ( 'NONE', #5024 ) ;
#29665=CARTESIAN_POINT ( 'NONE',  ( -14.81197284684445670, 20.44044478137485399, 10.76099332938164288 ) ) ;
#29666=CIRCLE ( 'NONE', #16037, 6.000000000000014211 ) ;
#29670=EDGE_CURVE ( 'NONE', #37999, #34064, #29666, .T. ) ;
#29671=DIRECTION ( 'NONE',  ( -0.5877852522924791323, -0.8090169943749430104, 0.000000000000000000 ) ) ;
#29672=ADVANCED_FACE ( 'NONE', ( #32669 ), #29808, .F. ) ;
#29673=EDGE_LOOP ( 'NONE', ( #6152, #35985, #28588, #33451 ) ) ;
#29674=ORIENTED_EDGE ( 'NONE', *, *, #22044, .T. ) ;
#29676=DIRECTION ( 'NONE',  ( 1.000000000000000000, 0.000000000000000000, 0.000000000000000000 ) ) ;
#29677=DIRECTION ( 'NONE',  ( -0.000000000000000000, -0.000000000000000000, -1.000000000000000000 ) ) ;
#29679=DIRECTION ( 'NONE',  ( -0.1045284632676436176, 0.9945218953682742891, 0.000000000000000000 ) ) ;
#29680=ORIENTED_EDGE ( 'NONE', *, *, #27748, .F. ) ;
#29683=DIRECTION ( 'NONE',  ( -0.000000000000000000, -0.000000000000000000, -1.000000000000000000 ) ) ;
#29687=CARTESIAN_POINT ( 'NONE',  ( 11.94134295108989896, 16.18301270189217433, 9.500000000000000000 ) ) ;
#29688=EDGE_LOOP ( 'NONE', ( #36543, #39082, #25806 ) ) ;
#29690=CIRCLE ( 'NONE', #30960, 0.5000000000000000000 ) ;
#29692=ORIENTED_EDGE ( 'NONE', *, *, #19694, .T. ) ;
#29694=CONICAL_SURFACE ( 'NONE', #18678, 0.9999999999999974465, 0.7853981633974554954 ) ;
#29696=DIRECTION ( 'NONE',  ( -0.000000000000000000, -0.000000000000000000, -1.000000000000000000 ) ) ;
#29702=CARTESIAN_POINT ( 'NONE',  ( -13.00577423375715114, 27.77729443754455829, 10.50000000000000000 ) ) ;
#29703=EDGE_CURVE ( 'NONE', #22904, #21130, #8067, .T. ) ;
#29705=LINE ( 'NONE', #8376, #11302 ) ;
#29709=AXIS2_PLACEMENT_3D ( 'NONE', #19117, #18920, #31308 ) ;
#29710=DIRECTION ( 'NONE',  ( 0.000000000000000000, 0.000000000000000000, 1.000000000000000000 ) ) ;
#29711=CARTESIAN_POINT ( 'NONE',  ( 2.231660708550581962, 7.803782283739836956, 10.49999999999999822 ) ) ;
#29715=ORIENTED_EDGE ( 'NONE', *, *, #32753, .F. ) ;
#29719=CARTESIAN_POINT ( 'NONE',  ( 4.058514655873871391, 8.059341904692812975, 7.339470489435487188 ) ) ;
#29721=VERTEX_POINT ( 'NONE', #36112 ) ;
#29723=ORIENTED_EDGE ( 'NONE', *, *, #1407, .F. ) ;
#29724=VECTOR ( 'NONE', #3015, 1000.000000000000000 ) ;
#29726=LINE ( 'NONE', #5340, #1743 ) ;
#29728=DIRECTION ( 'NONE',  ( 0.4539904997395342034, -0.8910065241883743381, -1.196099074440426220E-16 ) ) ;
#29737=CARTESIAN_POINT ( 'NONE',  ( -8.229154955995012344, 10.32288908946084760, 10.96580508970281187 ) ) ;
#29739=EDGE_LOOP ( 'NONE', ( #6047, #1534, #6775, #39727 ) ) ;
#29747=DIRECTION ( 'NONE',  ( 0.4999999999999920619, -0.8660254037844432595, 0.000000000000000000 ) ) ;
#29748=VECTOR ( 'NONE', #1814, 999.9999999999998863 ) ;
#29749=AXIS2_PLACEMENT_3D ( 'NONE', #11006, #39225, #35786 ) ;
#29750=DIRECTION ( 'NONE',  ( 1.000000000000000000, 0.000000000000000000, 0.000000000000000000 ) ) ;
#29751=ADVANCED_FACE ( 'NONE', ( #7864 ), #24111, .T. ) ;
#29753=VECTOR ( 'NONE', #9306, 1000.000000000000227 ) ;
#29756=CARTESIAN_POINT ( 'NONE',  ( 0.000000000000000000, 22.50000000000000355, 7.000000000000000000 ) ) ;
#29757=DIRECTION ( 'NONE',  ( -0.000000000000000000, -0.000000000000000000, -1.000000000000000000 ) ) ;
#29758=VERTEX_POINT ( 'NONE', #20875 ) ;
#29761=DIRECTION ( 'NONE',  ( -1.000000000000000000, 0.000000000000000000, 0.000000000000000000 ) ) ;
#29763=CARTESIAN_POINT ( 'NONE',  ( -8.927394655428429360, 11.06314620770957013, 7.000000000000000000 ) ) ;
#29764=CARTESIAN_POINT ( 'NONE',  ( -14.50704651774856835, 20.00412295564782283, 10.49999999999999822 ) ) ;
#29770=CARTESIAN_POINT ( 'NONE',  ( -7.824485034907249670, 10.87986945260456295, 7.499999999999999112 ) ) ;
#29772=ORIENTED_EDGE ( 'NONE', *, *, #17772, .F. ) ;
#29773=FACE_OUTER_BOUND ( 'NONE', #13198, .T. ) ;
#29774=ORIENTED_EDGE ( 'NONE', *, *, #11997, .T. ) ;
#29777=EDGE_CURVE ( 'NONE', #39013, #7898, #17369, .T. ) ;
#29780=ADVANCED_FACE ( 'NONE', ( #12908 ), #22518, .T. ) ;
#29787=DIRECTION ( 'NONE',  ( 0.000000000000000000, 0.000000000000000000, -1.000000000000000000 ) ) ;
#29789=CARTESIAN_POINT ( 'NONE',  ( 2.036571916123615100, 8.108948098542045457, 10.49999999999999467 ) ) ;
#29796=EDGE_CURVE ( 'NONE', #18134, #11440, #15403, .T. ) ;
#29798=EDGE_CURVE ( 'NONE', #2507, #26077, #36170, .T. ) ;
#29799=VERTEX_POINT ( 'NONE', #9075 ) ;
#29801=CIRCLE ( 'NONE', #28516, 1.000000000000000888 ) ;
#29802=DIRECTION ( 'NONE',  ( -0.9135454576426006446, 0.4067366430758009299, 0.000000000000000000 ) ) ;
#29803=CARTESIAN_POINT ( 'NONE',  ( -9.997483185316569987, 21.95197631500770896, 10.49999999999999467 ) ) ;
#29807=VECTOR ( 'NONE', #18313, 999.9999999999998863 ) ;
#29808=PLANE ( 'NONE',  #20610 ) ;
#29812=PLANE ( 'NONE',  #26997 ) ;
#29813=ORIENTED_EDGE ( 'NONE', *, *, #20537, .T. ) ;
#29815=LINE ( 'NONE', #39358, #5763 ) ;
#29816=CARTESIAN_POINT ( 'NONE',  ( -0.4999999999999998890, 37.39061994947694245, 10.82238861112329076 ) ) ;
#29818=CARTESIAN_POINT ( 'NONE',  ( 5.490944681523308724, 34.83286367817510154, 7.000000000000000000 ) ) ;
#29820=DIRECTION ( 'NONE',  ( 0.000000000000000000, 0.000000000000000000, -1.000000000000000000 ) ) ;
#29821=CARTESIAN_POINT ( 'NONE',  ( -8.593266739736659332, 16.38397459621564067, 10.49999999999999822 ) ) ;
#29828=VERTEX_POINT ( 'NONE', #2775 ) ;
#29830=VERTEX_POINT ( 'NONE', #27557 ) ;
#29832=CARTESIAN_POINT ( 'NONE',  ( 14.61656768153249786, 21.96308928146552120, 10.49999999999999822 ) ) ;
#29835=CARTESIAN_POINT ( 'NONE',  ( 9.417813166173738537, 10.93662330136606009, 10.49999999999999822 ) ) ;
#29839=ORIENTED_EDGE ( 'NONE', *, *, #23558, .F. ) ;
#29841=ORIENTED_EDGE ( 'NONE', *, *, #24797, .F. ) ;
#29843=CARTESIAN_POINT ( 'NONE',  ( -0.4999999999999998890, 37.13089969389958611, 11.00000000000000178 ) ) ;
#29844=ORIENTED_EDGE ( 'NONE', *, *, #18199, .T. ) ;
#29845=LINE ( 'NONE', #10762, #32694 ) ;
#29846=DIRECTION ( 'NONE',  ( 1.000000000000000000, 0.000000000000000000, 0.000000000000000000 ) ) ;
#29851=DIRECTION ( 'NONE',  ( 0.000000000000000000, 0.000000000000000000, -1.000000000000000000 ) ) ;
#29857=DIRECTION ( 'NONE',  ( -1.000000000000000000, 0.000000000000000000, 0.000000000000000000 ) ) ;
#29858=DIRECTION ( 'NONE',  ( -0.000000000000000000, -0.000000000000000000, -1.000000000000000000 ) ) ;
#29861=CIRCLE ( 'NONE', #27291, 0.5000000000000000000 ) ;
#29862=LINE ( 'NONE', #14424, #5588 ) ;
#29868=VERTEX_POINT ( 'NONE', #15964 ) ;
#29869=EDGE_LOOP ( 'NONE', ( #8597, #19713, #29594, #20182 ) ) ;
#29871=DIRECTION ( 'NONE',  ( 0.000000000000000000, 0.000000000000000000, 1.000000000000000000 ) ) ;
#29873=AXIS2_PLACEMENT_3D ( 'NONE', #19446, #25939, #32457 ) ;
#29876=EDGE_LOOP ( 'NONE', ( #30632, #14838, #19691, #1370, #4080, #39176, #31825, #1497 ) ) ;
#29878=ADVANCED_FACE ( 'NONE', ( #15566 ), #6410, .T. ) ;
#29879=AXIS2_PLACEMENT_3D ( 'NONE', #15563, #27950, #124 ) ;
#29880=CARTESIAN_POINT ( 'NONE',  ( 11.44169217588633636, 32.12932954397578555, 10.76099332938163755 ) ) ;
#29881=PLANE ( 'NONE',  #29749 ) ;
#29883=ADVANCED_FACE ( 'NONE', ( #28345 ), #22055, .F. ) ;
#29884=EDGE_LOOP ( 'NONE', ( #27662, #33515, #26537, #11232 ) ) ;
#29886=FACE_OUTER_BOUND ( 'NONE', #30299, .T. ) ;
#29887=ORIENTED_EDGE ( 'NONE', *, *, #20812, .T. ) ;
#29894=CARTESIAN_POINT ( 'NONE',  ( -3.000488737322915878, 30.46850471150003159, 9.000000000000001776 ) ) ;
#29896=CARTESIAN_POINT ( 'NONE',  ( 13.81877807188817364, 20.04207961888452871, 10.50000000000000000 ) ) ;
#29898=EDGE_CURVE ( 'NONE', #28064, #3290, #33865, .T. ) ;
#29900=EDGE_CURVE ( 'NONE', #42, #15406, #37105, .T. ) ;
#29901=DIRECTION ( 'NONE',  ( 0.000000000000000000, 0.000000000000000000, 1.000000000000000000 ) ) ;
#29902=EDGE_CURVE ( 'NONE', #13055, #29941, #21854, .T. ) ;
#29905=LINE ( 'NONE', #26856, #39840 ) ;
#29907=VECTOR ( 'NONE', #36397, 1000.000000000000000 ) ;
#29909=CYLINDRICAL_SURFACE ( 'NONE', #1583, 0.5000000000000004441 ) ;
#29911=DIRECTION ( 'NONE',  ( -0.2113248654051873565, 0.7886751345948044278, 0.5773502691896372774 ) ) ;
#29912=VERTEX_POINT ( 'NONE', #21655 ) ;
#29917=CARTESIAN_POINT ( 'NONE',  ( 4.360713706315008764, 8.147350538441772372, 7.102637441331451029 ) ) ;
#29923=FACE_OUTER_BOUND ( 'NONE', #5353, .T. ) ;
#29925=EDGE_CURVE ( 'NONE', #32427, #15193, #18224, .T. ) ;
#29927=EDGE_LOOP ( 'NONE', ( #3607, #29286, #18108 ) ) ;
#29935=EDGE_LOOP ( 'NONE', ( #2732, #25507, #8961, #7285, #11986 ) ) ;
#29938=VECTOR ( 'NONE', #5867, 1000.000000000000114 ) ;
#29940=AXIS2_PLACEMENT_3D ( 'NONE', #30255, #2031, #23753 ) ;
#29941=VERTEX_POINT ( 'NONE', #31010 ) ;
#29944=DIRECTION ( 'NONE',  ( -0.000000000000000000, -0.000000000000000000, 1.000000000000000000 ) ) ;
#29946=VECTOR ( 'NONE', #28028, 1000.000000000000000 ) ;
#29948=EDGE_CURVE ( 'NONE', #22045, #12690, #126, .T. ) ;
#29950=CARTESIAN_POINT ( 'NONE',  ( 6.354454053420413473, 35.54304081427980577, 11.00000000000000000 ) ) ;
#29951=CARTESIAN_POINT ( 'NONE',  ( 14.91782843052409646, 20.93207305098514581, 7.000000000000000000 ) ) ;
#29952=ORIENTED_EDGE ( 'NONE', *, *, #10345, .F. ) ;
#29954=CARTESIAN_POINT ( 'NONE',  ( -13.46929972531958697, 26.35070966310183138, 7.499999999999993783 ) ) ;
#29957=DIRECTION ( 'NONE',  ( -0.9510565162951543083, -0.3090169943749450088, 0.000000000000000000 ) ) ;
#29958=DIRECTION ( 'NONE',  ( -0.000000000000000000, -0.000000000000000000, -1.000000000000000000 ) ) ;
#29961=ORIENTED_EDGE ( 'NONE', *, *, #15471, .F. ) ;
#29962=AXIS2_PLACEMENT_3D ( 'NONE', #34697, #6459, #19250 ) ;
#29968=CARTESIAN_POINT ( 'NONE',  ( -14.75621568350166513, 21.89813303538607059, 10.49999999999999822 ) ) ;
#29971=CARTESIAN_POINT ( 'NONE',  ( -12.30736835487442882, 14.81698729810789672, 9.500000000000000000 ) ) ;
#29973=ADVANCED_FACE ( 'NONE', ( #37299 ), #31202, .T. ) ;
#29979=ORIENTED_EDGE ( 'NONE', *, *, #22458, .F. ) ;
#29980=EDGE_CURVE ( 'NONE', #22931, #36670, #21264, .T. ) ;
#29983=AXIS2_PLACEMENT_3D ( 'NONE', #26838, #8359, #17515 ) ;
#29984=EDGE_CURVE ( 'NONE', #35419, #37631, #16774, .T. ) ;
#29995=PRESENTATION_STYLE_ASSIGNMENT (( #5212 ) ) ;
#29996=FACE_OUTER_BOUND ( 'NONE', #19176, .T. ) ;
#29997=CIRCLE ( 'NONE', #19599, 0.5000000000000004441 ) ;
#29998=EDGE_LOOP ( 'NONE', ( #25870, #8667, #20031, #36387 ) ) ;
#29999=EDGE_CURVE ( 'NONE', #17070, #29633, #19403, .T. ) ;
#30000=DIRECTION ( 'NONE',  ( 0.4999999999999920064, -0.8660254037844432595, 0.000000000000000000 ) ) ;
#30002=ADVANCED_FACE ( 'NONE', ( #29353 ), #1327, .F. ) ;
#30004=FACE_OUTER_BOUND ( 'NONE', #14598, .T. ) ;
#30006=DIRECTION ( 'NONE',  ( 1.000000000000000000, 0.000000000000000000, 0.000000000000000000 ) ) ;
#30007=LINE ( 'NONE', #21067, #25345 ) ;
#30008=AXIS2_PLACEMENT_3D ( 'NONE', #14853, #40019, #12001 ) ;
#30010=CARTESIAN_POINT ( 'NONE',  ( 8.633502029282041690, 11.46765470489692795, 7.499999999999999112 ) ) ;
#30014=DIRECTION ( 'NONE',  ( 1.000000000000000000, 0.000000000000000000, 0.000000000000000000 ) ) ;
#30015=EDGE_LOOP ( 'NONE', ( #17030, #21890, #6122 ) ) ;
#30016=CIRCLE ( 'NONE', #15744, 0.4999999999999997780 ) ;
#30019=CARTESIAN_POINT ( 'NONE',  ( -13.72527515842276280, 27.95206079998173365, 10.49999999999999822 ) ) ;
#30021=B_SPLINE_CURVE_WITH_KNOTS ( 'NONE', 3,
 ( #37488, #34245, #34047, #9064 ),
 .UNSPECIFIED., .F., .F.,
 ( 4, 4 ),
 ( 0.000000000000000000, 1.000000000000000000 ),
 .UNSPECIFIED. ) ;
#30022=CARTESIAN_POINT ( 'NONE',  ( -3.610593701936590350, 31.83882289796395426, 10.50000000000000533 ) ) ;
#30026=ADVANCED_FACE ( 'NONE', ( #26099 ), #19926, .T. ) ;
#30028=VECTOR ( 'NONE', #30521, 999.9999999999998863 ) ;
#30031=EDGE_CURVE ( 'NONE', #3751, #24567, #9200, .T. ) ;
#30033=DIRECTION ( 'NONE',  ( 0.7431448254773954654, 0.6691306063588570163, 0.000000000000000000 ) ) ;
#30037=AXIS2_PLACEMENT_3D ( 'NONE', #1431, #39204, #13813 ) ;
#30041=CIRCLE ( 'NONE', #33953, 1.000000000000004441 ) ;
#30043=ORIENTED_EDGE ( 'NONE', *, *, #33211, .F. ) ;
#30045=ORIENTED_EDGE ( 'NONE', *, *, #29605, .F. ) ;
#30047=ORIENTED_EDGE ( 'NONE', *, *, #29984, .T. ) ;
#30048=DIRECTION ( 'NONE',  ( 0.5877852522924696954, -0.8090169943749500048, 0.000000000000000000 ) ) ;
#30050=CARTESIAN_POINT ( 'NONE',  ( 14.97009266215792778, 21.42933399866928568, 10.49999999999999822 ) ) ;
#30051=FACE_OUTER_BOUND ( 'NONE', #18591, .T. ) ;
#30052=AXIS2_PLACEMENT_3D ( 'NONE', #24313, #27757, #39943 ) ;
#30053=DIRECTION ( 'NONE',  ( 0.5877852522924690293, -0.8090169943749503378, 0.000000000000000000 ) ) ;
#30054=ORIENTED_EDGE ( 'NONE', *, *, #9966, .F. ) ;
#30058=CARTESIAN_POINT ( 'NONE',  ( -14.47283171447380390, 21.48159823030330884, 11.00000000000000000 ) ) ;
#30059=VECTOR ( 'NONE', #11859, 1000.000000000000227 ) ;
#30060=DIRECTION ( 'NONE',  ( -0.8660254037844431485, -0.4999999999999921174, 0.000000000000000000 ) ) ;
#30065=CARTESIAN_POINT ( 'NONE',  ( 10.77256156952748256, 32.87247436945319379, 10.76099332938163933 ) ) ;
#30066=DIRECTION ( 'NONE',  ( 0.000000000000000000, 0.000000000000000000, 1.000000000000000000 ) ) ;
#30071=CARTESIAN_POINT ( 'NONE',  ( -9.080802685385670259, 10.85199816882132673, 10.94611345180490503 ) ) ;
#30075=CARTESIAN_POINT ( 'NONE',  ( 11.54426418658508879, 32.09594396785328740, 10.49999999999999822 ) ) ;
#30076=ORIENTED_EDGE ( 'NONE', *, *, #3219, .F. ) ;
#30077=ORIENTED_EDGE ( 'NONE', *, *, #10108, .T. ) ;
#30079=FACE_OUTER_BOUND ( 'NONE', #9393, .T. ) ;
#30080=DIRECTION ( 'NONE',  ( -0.9135454576426059736, -0.4067366430757888285, 0.000000000000000000 ) ) ;
#30083=VERTEX_POINT ( 'NONE', #10065 ) ;
#30086=PLANE ( 'NONE',  #9013 ) ;
#30087=CARTESIAN_POINT ( 'NONE',  ( -19.48557158514982390, 33.75000000000009948, 7.000000000000000000 ) ) ;
#30088=ORIENTED_EDGE ( 'NONE', *, *, #16972, .T. ) ;
#30090=DIRECTION ( 'NONE',  ( 0.5906904945688790098, 0.000000000000000000, 0.8068982213550685012 ) ) ;
#30099=B_SPLINE_CURVE_WITH_KNOTS ( 'NONE', 3,
 ( #18795, #6194, #12687, #2953, #12295, #15545, #37868, #30790 ),
 .UNSPECIFIED., .F., .F.,
 ( 4, 2, 2, 4 ),
 ( 0.000000000000000000, 0.0002364868538934310324, 0.0004729737077868620648, 0.0009459474155737337790 ),
 .UNSPECIFIED. ) ;
#30101=VECTOR ( 'NONE', #9909, 1000.000000000000000 ) ;
#30102=CARTESIAN_POINT ( 'NONE',  ( 5.237540274239913529, 35.49300472853430222, 9.500000000000000000 ) ) ;
#30104=EDGE_CURVE ( 'NONE', #39958, #14016, #4574, .T. ) ;
#30105=CARTESIAN_POINT ( 'NONE',  ( 11.87435565298210882, 15.06698729810772619, 7.499999999999997335 ) ) ;
#30106=PLANE ( 'NONE',  #33169 ) ;
#30108=PLANE ( 'NONE',  #26891 ) ;
#30112=EDGE_CURVE ( 'NONE', #39108, #29636, #724, .T. ) ;
#30115=CARTESIAN_POINT ( 'NONE',  ( -14.44277748876678302, 26.55045409923029354, 7.000000000000000000 ) ) ;
#30116=CARTESIAN_POINT ( 'NONE',  ( 2.623829155769261678, 7.750987179267949223, 10.68306085400107008 ) ) ;
#30117=EDGE_LOOP ( 'NONE', ( #14864, #35615, #14067 ) ) ;
#30119=AXIS2_PLACEMENT_3D ( 'NONE', #12817, #13014, #37800 ) ;
#30120=EDGE_LOOP ( 'NONE', ( #10742, #2149, #18063, #15090, #16143 ) ) ;
#30123=FACE_OUTER_BOUND ( 'NONE', #31433, .T. ) ;
#30127=ORIENTED_EDGE ( 'NONE', *, *, #34556, .F. ) ;
#30137=ORIENTED_EDGE ( 'NONE', *, *, #5658, .F. ) ;
#30139=DIRECTION ( 'NONE',  ( -0.6847716512521441201, 0.4446959099295496043, 0.5773502691896332806 ) ) ;
#30140=ADVANCED_FACE ( 'NONE', ( #31594 ), #34853, .T. ) ;
#30142=ADVANCED_FACE ( 'NONE', ( #25304 ), #37698, .T. ) ;
#30145=ORIENTED_EDGE ( 'NONE', *, *, #36685, .F. ) ;
#30150=DIRECTION ( 'NONE',  ( -0.9945218953682744001, -0.1045284632676437842, 0.000000000000000000 ) ) ;
#30152=LINE ( 'NONE', #20209, #519 ) ;
#30153=DIRECTION ( 'NONE',  ( 0.000000000000000000, 0.000000000000000000, 1.000000000000000000 ) ) ;
#30154=DIRECTION ( 'NONE',  ( -0.000000000000000000, 0.000000000000000000, 1.000000000000000000 ) ) ;
#30155=VECTOR ( 'NONE', #14972, 1000.000000000000000 ) ;
#30156=ADVANCED_FACE ( 'NONE', ( #38091 ), #2810, .T. ) ;
#30157=CIRCLE ( 'NONE', #23009, 0.4999999999999995559 ) ;
#30158=CARTESIAN_POINT ( 'NONE',  ( -15.64741614794215252, 37.44040872933206288, 7.500000000000004441 ) ) ;
#30160=ORIENTED_EDGE ( 'NONE', *, *, #23125, .T. ) ;
#30162=CARTESIAN_POINT ( 'NONE',  ( 0.000000000000000000, 22.50000000000000355, 7.000000000000000000 ) ) ;
#30163=DIRECTION ( 'NONE',  ( 0.000000000000000000, -0.6037757019622743693, -0.7971542521494587863 ) ) ;
#30172=DIRECTION ( 'NONE',  ( -0.6123724356957963577, -0.3535533905932721210, -0.7071067811865466846 ) ) ;
#30174=EDGE_LOOP ( 'NONE', ( #35358, #8539, #24986, #25778 ) ) ;
#30175=CARTESIAN_POINT ( 'NONE',  ( 8.505700342264139735, 22.10876900990906435, 7.000000000000000000 ) ) ;
#30176=ORIENTED_EDGE ( 'NONE', *, *, #27545, .F. ) ;
#30178=CARTESIAN_POINT ( 'NONE',  ( -3.503793317224517700, 8.420815634768727520, 7.499999999999997335 ) ) ;
#30179=B_SPLINE_CURVE_WITH_KNOTS ( 'NONE', 3,
 ( #12586, #40010, #31278, #37372, #6284, #30684 ),
 .UNSPECIFIED., .F., .F.,
 ( 4, 2, 4 ),
 ( 0.000000000000000000, 0.5000000000000000000, 1.000000000000000000 ),
 .UNSPECIFIED. ) ;
#30191=ADVANCED_FACE ( 'NONE', ( #22645 ), #1128, .T. ) ;
#30193=VECTOR ( 'NONE', #17798, 1000.000000000000000 ) ;
#30194=EDGE_LOOP ( 'NONE', ( #28405, #27315, #26623 ) ) ;
#30197=AXIS2_PLACEMENT_3D ( 'NONE', #11049, #10435, #32384 ) ;
#30198=DIRECTION ( 'NONE',  ( 0.000000000000000000, 0.000000000000000000, -1.000000000000000000 ) ) ;
#30200=DIRECTION ( 'NONE',  ( -0.4156269377774519103, 0.5720614028176885801, -0.7071067811865450192 ) ) ;
#30202=ORIENTED_EDGE ( 'NONE', *, *, #10619, .T. ) ;
#30203=CARTESIAN_POINT ( 'NONE',  ( -11.69134295108998245, 15.75000000000011191, 7.000000000000000000 ) ) ;
#30204=EDGE_CURVE ( 'NONE', #3600, #257, #22250, .T. ) ;
#30205=CARTESIAN_POINT ( 'NONE',  ( 8.339609403135803234, 11.87216320208440834, 7.000000000000000000 ) ) ;
#30206=ORIENTED_EDGE ( 'NONE', *, *, #32515, .F. ) ;
#30207=ADVANCED_FACE ( 'NONE', ( #17183 ), #26710, .T. ) ;
#30209=LINE ( 'NONE', #30612, #3611 ) ;
#30213=AXIS2_PLACEMENT_3D ( 'NONE', #10630, #26467, #35620 ) ;
#30214=CARTESIAN_POINT ( 'NONE',  ( 8.118377661053324701, 10.47536095541698486, 7.500000000000000888 ) ) ;
#30218=CARTESIAN_POINT ( 'NONE',  ( -7.353987181296344211, 35.57359447655193208, 7.000000000000000000 ) ) ;
#30219=VECTOR ( 'NONE', #10258, 1000.000000000000114 ) ;
#30224=CARTESIAN_POINT ( 'NONE',  ( 12.83926296998457950, 26.67172942406175906, 7.000000000000000000 ) ) ;
#30225=CARTESIAN_POINT ( 'NONE',  ( 0.5000000000000002220, 36.50000000000000711, 7.500000000000000888 ) ) ;
#30229=ORIENTED_EDGE ( 'NONE', *, *, #13084, .T. ) ;
#30230=FACE_OUTER_BOUND ( 'NONE', #4888, .T. ) ;
#30231=DIRECTION ( 'NONE',  ( -0.3535533905932740084, -0.6123724356957886972, -0.7071067811865524577 ) ) ;
#30236=CARTESIAN_POINT ( 'NONE',  ( -6.576253646258510166, 14.29921418520934040, 10.00000000000000000 ) ) ;
#30238=EDGE_CURVE ( 'NONE', #7488, #18790, #8222, .T. ) ;
#30239=ORIENTED_EDGE ( 'NONE', *, *, #38771, .T. ) ;
#30240=ADVANCED_FACE ( 'NONE', ( #11280 ), #36267, .T. ) ;
#30242=VERTEX_POINT ( 'NONE', #14319 ) ;
#30243=FACE_OUTER_BOUND ( 'NONE', #33383, .T. ) ;
#30244=CARTESIAN_POINT ( 'NONE',  ( -8.380596568873706076, 10.11444759148765549, 10.76099332938163577 ) ) ;
#30245=AXIS2_PLACEMENT_3D ( 'NONE', #36771, #14836, #30877 ) ;
#30248=AXIS2_PLACEMENT_3D ( 'NONE', #32674, #26966, #24709 ) ;
#30249=AXIS2_PLACEMENT_3D ( 'NONE', #15777, #24923, #33880 ) ;
#30254=DIRECTION ( 'NONE',  ( -0.5877852522924796874, -0.8090169943749426773, 0.000000000000000000 ) ) ;
#30255=CARTESIAN_POINT ( 'NONE',  ( 2.140527761532493134, 7.619874298175136396, 10.49999999999999467 ) ) ;
#30256=EDGE_CURVE ( 'NONE', #2610, #37186, #1510, .T. ) ;
#30258=ORIENTED_EDGE ( 'NONE', *, *, #24188, .F. ) ;
#30261=DIRECTION ( 'NONE',  ( 0.9945218953682729568, -0.1045284632676569680, 0.000000000000000000 ) ) ;
#30263=CARTESIAN_POINT ( 'NONE',  ( 2.518583951651050867, 7.712953814960687104, 7.499999999999990230 ) ) ;
#30268=EDGE_CURVE ( 'NONE', #2021, #37780, #8018, .T. ) ;
#30270=PLANE ( 'NONE',  #39771 ) ;
#30271=CARTESIAN_POINT ( 'NONE',  ( -14.79690083935193989, 20.03899165096060386, 7.382773698552470343 ) ) ;
#30273=DIRECTION ( 'NONE',  ( -0.1045284632676436315, 0.9945218953682742891, 0.000000000000000000 ) ) ;
#30274=CARTESIAN_POINT ( 'NONE',  ( -9.189613563248645534, 10.70223284378013062, 10.76099332938163577 ) ) ;
#30280=CARTESIAN_POINT ( 'NONE',  ( 11.56190694343555947, 31.61076883254013126, 10.49999999999999822 ) ) ;
#30281=ORIENTED_EDGE ( 'NONE', *, *, #3071, .T. ) ;
#30282=ORIENTED_EDGE ( 'NONE', *, *, #16486, .F. ) ;
#30285=LINE ( 'NONE', #38819, #13304 ) ;
#30286=LINE ( 'NONE', #2253, #10728 ) ;
#30288=CARTESIAN_POINT ( 'NONE',  ( -9.426561227484903327, 11.13126706419782508, 10.49999999999999822 ) ) ;
#30289=ORIENTED_EDGE ( 'NONE', *, *, #7760, .F. ) ;
#30291=LINE ( 'NONE', #35987, #25169 ) ;
#30292=DIRECTION ( 'NONE',  ( 0.9135454576426048634, 0.4067366430757912710, 0.000000000000000000 ) ) ;
#30293=ORIENTED_EDGE ( 'NONE', *, *, #23075, .T. ) ;
#30295=DIRECTION ( 'NONE',  ( 0.6123724356957959136, 0.3535533905932670140, 0.7071067811865496822 ) ) ;
#30299=EDGE_LOOP ( 'NONE', ( #32573, #1882, #36557 ) ) ;
#30302=CARTESIAN_POINT ( 'NONE',  ( 7.929471891321336230, 25.60217271033461373, 9.000000000000001776 ) ) ;
#30305=AXIS2_PLACEMENT_3D ( 'NONE', #26581, #13781, #1198 ) ;
#30308=EDGE_CURVE ( 'NONE', #13430, #12503, #10582, .T. ) ;
#30309=DIRECTION ( 'NONE',  ( -0.9510565162951503115, 0.3090169943749573878, -0.000000000000000000 ) ) ;
#30310=DIRECTION ( 'NONE',  ( 0.9781476007338067991, 0.2079116908177533474, -0.000000000000000000 ) ) ;
#30311=AXIS2_PLACEMENT_3D ( 'NONE', #6016, #6217, #21460 ) ;
#30316=DIRECTION ( 'NONE',  ( -0.000000000000000000, -0.000000000000000000, -1.000000000000000000 ) ) ;
#30317=CARTESIAN_POINT ( 'NONE',  ( -9.665073660138977729, 25.11464168560200250, 10.00000000000000000 ) ) ;
#30318=CARTESIAN_POINT ( 'NONE',  ( -4.794796183862964689, 36.71301971979259804, 7.000000000000000000 ) ) ;
#30319=ORIENTED_EDGE ( 'NONE', *, *, #27745, .T. ) ;
#30321=ORIENTED_EDGE ( 'NONE', *, *, #21849, .T. ) ;
#30324=CARTESIAN_POINT ( 'NONE',  ( -3.513409677696690991, 8.375574215747771945, 10.99999999999999289 ) ) ;
#30328=VERTEX_POINT ( 'NONE', #10880 ) ;
#30330=CARTESIAN_POINT ( 'NONE',  ( 7.899339922805233449, 10.02167583667219830, 10.49999999999999822 ) ) ;
#30332=CARTESIAN_POINT ( 'NONE',  ( 13.63581098909226519, 27.45627467658428600, 11.00000000000000000 ) ) ;
#30333=CIRCLE ( 'NONE', #22509, 0.5000000000000001110 ) ;
#30342=CARTESIAN_POINT ( 'NONE',  ( -8.087160441415543133, 9.969847506823033001, 10.49999999999999822 ) ) ;
#30344=EDGE_CURVE ( 'NONE', #32472, #6988, #20335, .T. ) ;
#30345=AXIS2_PLACEMENT_3D ( 'NONE', #21841, #36698, #117 ) ;
#30346=ORIENTED_EDGE ( 'NONE', *, *, #15317, .F. ) ;
#30348=VERTEX_POINT ( 'NONE', #38703 ) ;
#30350=VECTOR ( 'NONE', #11106, 1000.000000000000227 ) ;
#30355=LINE ( 'NONE', #9011, #22272 ) ;
#30356=DIRECTION ( 'NONE',  ( -0.4067366430757889395, 0.9135454576426058626, 0.000000000000000000 ) ) ;
#30360=VECTOR ( 'NONE', #6883, 1000.000000000000000 ) ;
#30363=FACE_OUTER_BOUND ( 'NONE', #10304, .T. ) ;
#30364=EDGE_LOOP ( 'NONE', ( #39584, #2685, #5483, #5953 ) ) ;
#30367=ADVANCED_FACE ( 'NONE', ( #20221 ), #19680, .T. ) ;
#30371=DIRECTION ( 'NONE',  ( -1.000000000000000000, 0.000000000000000000, 0.000000000000000000 ) ) ;
#30374=B_SPLINE_CURVE_WITH_KNOTS ( 'NONE', 3,
 ( #15713, #37055, #21608, #13255, #16723, #15917 ),
 .UNSPECIFIED., .F., .F.,
 ( 4, 2, 4 ),
 ( 0.3333333336416847703, 0.6666666668208423019, 1.000000000000000000 ),
 .UNSPECIFIED. ) ;
#30384=PLANE ( 'NONE',  #12087 ) ;
#30386=CARTESIAN_POINT ( 'NONE',  ( -12.05736835487443237, 14.38397459621567442, 7.000000000000000000 ) ) ;
#30391=ORIENTED_EDGE ( 'NONE', *, *, #1712, .T. ) ;
#30393=EDGE_CURVE ( 'NONE', #2857, #28430, #4053, .T. ) ;
#30396=DIRECTION ( 'NONE',  ( -0.000000000000000000, -0.000000000000000000, -1.000000000000000000 ) ) ;
#30399=EDGE_CURVE ( 'NONE', #10635, #35497, #28041, .T. ) ;
#30400=AXIS2_PLACEMENT_3D ( 'NONE', #22479, #4403, #35286 ) ;
#30402=CIRCLE ( 'NONE', #12855, 0.5000000000000004441 ) ;
#30403=CARTESIAN_POINT ( 'NONE',  ( 5.034171952702011232, 35.03623199971301005, 9.500000000000000000 ) ) ;
#30404=ADVANCED_FACE ( 'NONE', ( #19100 ), #218, .T. ) ;
#30407=AXIS2_PLACEMENT_3D ( 'NONE', #15802, #27795, #37340 ) ;
#30410=AXIS2_PLACEMENT_3D ( 'NONE', #28378, #31234, #19043 ) ;
#30411=VERTEX_POINT ( 'NONE', #12998 ) ;
#30413=CARTESIAN_POINT ( 'NONE',  ( 13.63581098909226874, 27.45627467658428955, 9.000000000000001776 ) ) ;
#30414=CARTESIAN_POINT ( 'NONE',  ( -7.354454053420251824, 35.54304081427989814, 7.000000000000000000 ) ) ;
#30416=FACE_OUTER_BOUND ( 'NONE', #10278, .T. ) ;
#30418=DIRECTION ( 'NONE',  ( 0.9781476007338072431, 0.2079116908177519041, 0.000000000000000000 ) ) ;
#30420=CARTESIAN_POINT ( 'NONE',  ( -13.05736835487441994, 16.11602540378456183, 11.00000000000000000 ) ) ;
#30423=DIRECTION ( 'NONE',  ( -0.000000000000000000, 0.000000000000000000, -1.000000000000000000 ) ) ;
#30424=VECTOR ( 'NONE', #3430, 1000.000000000000000 ) ;
#30426=LINE ( 'NONE', #18032, #28292 ) ;
#30428=EDGE_LOOP ( 'NONE', ( #16812, #5901, #39825, #3863 ) ) ;
#30430=DIRECTION ( 'NONE',  ( -0.9510565162951543083, -0.3090169943749450088, 0.000000000000000000 ) ) ;
#30431=CARTESIAN_POINT ( 'NONE',  ( -14.00731263743711885, 27.57698287931463454, 10.82238861112334760 ) ) ;
#30436=EDGE_LOOP ( 'NONE', ( #12266, #35791, #31178, #28321 ) ) ;
#30437=DIRECTION ( 'NONE',  ( -0.7071067811865451302, -0.7071067811865499042, 1.559530880411979857E-16 ) ) ;
#30438=DIRECTION ( 'NONE',  ( 0.3535533905932750631, -0.6123724356958023529, -0.7071067811865401342 ) ) ;
#30445=ORIENTED_EDGE ( 'NONE', *, *, #27220, .T. ) ;
#30448=ORIENTED_EDGE ( 'NONE', *, *, #15825, .T. ) ;
#30449=DIRECTION ( 'NONE',  ( 0.1045284632676436315, -0.9945218953682742891, 0.000000000000000000 ) ) ;
#30452=ADVANCED_FACE ( 'NONE', ( #9957 ), #4105, .T. ) ;
#30454=CIRCLE ( 'NONE', #10986, 0.5000000000000004441 ) ;
#30456=ORIENTED_EDGE ( 'NONE', *, *, #19932, .T. ) ;
#30457=SHAPE_DEFINITION_REPRESENTATION ( #272, #28068 ) ;
#30459=ORIENTED_EDGE ( 'NONE', *, *, #3542, .T. ) ;
#30461=CARTESIAN_POINT ( 'NONE',  ( -11.19134295108999311, 14.88397459621566554, 9.500000000000000000 ) ) ;
#30462=DIRECTION ( 'NONE',  ( 0.000000000000000000, 0.000000000000000000, 1.000000000000000000 ) ) ;
#30463=ORIENTED_EDGE ( 'NONE', *, *, #24459, .T. ) ;
#30465=CARTESIAN_POINT ( 'NONE',  ( -6.151085731882353969, 35.08626808545859888, 7.500000000000000888 ) ) ;
#30466=DIRECTION ( 'NONE',  ( -0.9945218953682744001, -0.1045284632676437564, 0.000000000000000000 ) ) ;
#30468=EDGE_CURVE ( 'NONE', #26406, #22335, #10160, .T. ) ;
#30471=ORIENTED_EDGE ( 'NONE', *, *, #22084, .F. ) ;
#30474=CARTESIAN_POINT ( 'NONE',  ( -14.75241816305527642, 19.78287871224842220, 7.203056206335838318 ) ) ;
#30479=AXIS2_PLACEMENT_3D ( 'NONE', #13098, #6798, #28344 ) ;
#30482=FACE_OUTER_BOUND ( 'NONE', #24235, .T. ) ;
#30485=AXIS2_PLACEMENT_3D ( 'NONE', #3810, #9914, #35501 ) ;
#30488=EDGE_CURVE ( 'NONE', #25929, #29830, #16256, .T. ) ;
#30489=DIRECTION ( 'NONE',  ( 1.000000000000000000, 0.000000000000000000, 0.000000000000000000 ) ) ;
#30490=CARTESIAN_POINT ( 'NONE',  ( -9.353067506536522302, 10.78869951827630302, 10.49999999999999822 ) ) ;
#30491=EDGE_LOOP ( 'NONE', ( #19372, #16280, #33814, #11355 ) ) ;
#30495=CARTESIAN_POINT ( 'NONE',  ( 0.5000000000000002220, 36.50000000000000711, 7.500000000000000888 ) ) ;
#30496=ORIENTED_EDGE ( 'NONE', *, *, #1205, .F. ) ;
#30498=CARTESIAN_POINT ( 'NONE',  ( 14.36830325120613239, 20.48707633493483371, 11.00000000000000000 ) ) ;
#30501=ADVANCED_FACE ( 'NONE', ( #28642 ), #12552, .T. ) ;
#30503=VERTEX_POINT ( 'NONE', #37596 ) ;
#30506=CARTESIAN_POINT ( 'NONE',  ( -5.237540274239745663, 35.49300472853438038, 9.500000000000000000 ) ) ;
#30509=CARTESIAN_POINT ( 'NONE',  ( 4.003810537522394242, 8.420815593655317954, 10.49999999999999822 ) ) ;
#30512=DIRECTION ( 'NONE',  ( 0.1564344650402373915, 0.9876883405951366601, 1.143885345364396926E-15 ) ) ;
#30514=ADVANCED_FACE ( 'NONE', ( #21946 ), #22142, .T. ) ;
#30515=EDGE_CURVE ( 'NONE', #7567, #16860, #1019, .T. ) ;
#30521=DIRECTION ( 'NONE',  ( -0.6691306063588678965, -0.7431448254773855844, 0.000000000000000000 ) ) ;
#30523=ORIENTED_EDGE ( 'NONE', *, *, #21762, .F. ) ;
#30525=ORIENTED_EDGE ( 'NONE', *, *, #16636, .F. ) ;
#30527=CIRCLE ( 'NONE', #34400, 1.000000000000016431 ) ;
#30532=ORIENTED_EDGE ( 'NONE', *, *, #28950, .F. ) ;
#30533=ORIENTED_EDGE ( 'NONE', *, *, #8280, .T. ) ;
#30535=CARTESIAN_POINT ( 'NONE',  ( -6.677405195726899834, 35.94657184102484138, 10.49999999999999822 ) ) ;
#30538=DIRECTION ( 'NONE',  ( 0.3090169943749451198, -0.9510565162951544194, 0.000000000000000000 ) ) ;
#30545=EDGE_CURVE ( 'NONE', #4057, #17936, #3262, .T. ) ;
#30546=DIRECTION ( 'NONE',  ( -0.5000000000000039968, -0.8660254037844363761, 0.000000000000000000 ) ) ;
#30548=AXIS2_PLACEMENT_3D ( 'NONE', #12616, #15866, #24608 ) ;
#30549=ORIENTED_EDGE ( 'NONE', *, *, #3550, .F. ) ;
#30554=EDGE_LOOP ( 'NONE', ( #25074, #8012, #629, #1512 ) ) ;
#30557=CARTESIAN_POINT ( 'NONE',  ( 4.984135866956514782, 36.15314577889351000, 10.49999999999999467 ) ) ;
#30558=CIRCLE ( 'NONE', #36, 6.000000000000003553 ) ;
#30559=FACE_OUTER_BOUND ( 'NONE', #4380, .T. ) ;
#30564=ORIENTED_EDGE ( 'NONE', *, *, #23023, .T. ) ;
#30567=PLANE ( 'NONE',  #628 ) ;
#30569=EDGE_CURVE ( 'NONE', #32217, #25659, #35232, .T. ) ;
#30570=VECTOR ( 'NONE', #16217, 1000.000000000000000 ) ;
#30571=DIRECTION ( 'NONE',  ( 0.3535533905932713994, -0.6123724356958013537, -0.7071067811865427988 ) ) ;
#30577=DIRECTION ( 'NONE',  ( 0.000000000000000000, 0.000000000000000000, -1.000000000000000000 ) ) ;
#30580=B_SPLINE_CURVE_WITH_KNOTS ( 'NONE', 3,
 ( #26150, #38548, #23511, #21069 ),
 .UNSPECIFIED., .F., .F.,
 ( 4, 4 ),
 ( 0.000000000000000000, 1.000000000000000000 ),
 .UNSPECIFIED. ) ;
#30582=EDGE_LOOP ( 'NONE', ( #4042, #27153, #34629 ) ) ;
#30584=CARTESIAN_POINT ( 'NONE',  ( 13.32151712420403555, 20.09434385051836358, 10.00000000000000000 ) ) ;
#30586=CARTESIAN_POINT ( 'NONE',  ( -14.06524961900331760, 27.71236540882611621, 7.499999999999993783 ) ) ;
#30590=CARTESIAN_POINT ( 'NONE',  ( -5.767236651883567156, 13.71142893291686171, 10.50000000000000000 ) ) ;
#30594=CIRCLE ( 'NONE', #19548, 1.000000000000000888 ) ;
#30595=DIRECTION ( 'NONE',  ( -0.000000000000000000, 0.000000000000000000, -1.000000000000000000 ) ) ;
#30596=CARTESIAN_POINT ( 'NONE',  ( -8.910254037844422825, 17.93301270189230223, 10.49999999999999822 ) ) ;
#30597=CARTESIAN_POINT ( 'NONE',  ( -9.941034666242671847, 32.57396620494226624, 11.00000000000000000 ) ) ;
#30601=CARTESIAN_POINT ( 'NONE',  ( 5.034171952702011232, 35.03623199971301005, 9.500000000000000000 ) ) ;
#30605=ORIENTED_EDGE ( 'NONE', *, *, #36449, .T. ) ;
#30606=FACE_OUTER_BOUND ( 'NONE', #30364, .T. ) ;
#30608=CARTESIAN_POINT ( 'NONE',  ( 23.60287484585659001, 26.76891282270896610, 9.500000000000000000 ) ) ;
#30609=CARTESIAN_POINT ( 'NONE',  ( 9.677076426724163127, 26.69573495723207657, 10.50000000000000000 ) ) ;
#30612=CARTESIAN_POINT ( 'NONE',  ( -12.53024597560957609, 27.62278594035707968, 10.00000000000000000 ) ) ;
#30613=EDGE_CURVE ( 'NONE', #35248, #11406, #1418, .T. ) ;
#30614=CARTESIAN_POINT ( 'NONE',  ( 9.697889840765411051, 31.90483559858327212, 10.00000000000000000 ) ) ;
#30615=DIRECTION ( 'NONE',  ( 0.000000000000000000, -0.000000000000000000, 1.000000000000000000 ) ) ;
#30616=DIRECTION ( 'NONE',  ( 0.9135454576426005335, -0.4067366430758009299, 0.000000000000000000 ) ) ;
#30617=CARTESIAN_POINT ( 'NONE',  ( -9.593266739736646898, 18.11602540378452986, 11.00000000000000000 ) ) ;
#30618=CARTESIAN_POINT ( 'NONE',  ( -9.997483185316569987, 21.95197631500770896, 10.49999999999999467 ) ) ;
#30620=CARTESIAN_POINT ( 'NONE',  ( -4.940908595777636414, 35.94977745735568675, 7.500000000000000888 ) ) ;
#30623=FACE_OUTER_BOUND ( 'NONE', #7334, .T. ) ;
#30628=EDGE_CURVE ( 'NONE', #36251, #6243, #17066, .T. ) ;
#30632=ORIENTED_EDGE ( 'NONE', *, *, #19203, .F. ) ;
#30633=CYLINDRICAL_SURFACE ( 'NONE', #34134, 6.000000000000001776 ) ;
#30634=DIRECTION ( 'NONE',  ( 0.8660254037844431485, 0.4999999999999921174, -0.000000000000000000 ) ) ;
#30640=CARTESIAN_POINT ( 'NONE',  ( -8.315274455032252376, 10.01576150750523375, 7.500000000000000888 ) ) ;
#30646=CARTESIAN_POINT ( 'NONE',  ( -14.47283171447380390, 21.48159823030330884, 7.500000000000004441 ) ) ;
#30647=EDGE_CURVE ( 'NONE', #14093, #32234, #11164, .T. ) ;
#30648=DIRECTION ( 'NONE',  ( -0.3090169943749449533, 0.9510565162951544194, 0.000000000000000000 ) ) ;
#30652=VERTEX_POINT ( 'NONE', #14004 ) ;
#30653=VECTOR ( 'NONE', #24096, 1000.000000000000114 ) ;
#30654=CARTESIAN_POINT ( 'NONE',  ( 13.63581098909226519, 27.45627467658428600, 7.500000000000000888 ) ) ;
#30656=CARTESIAN_POINT ( 'NONE',  ( -5.400683141673551901, 15.91724817395922997, 9.000000000000001776 ) ) ;
#30660=ORIENTED_EDGE ( 'NONE', *, *, #33302, .T. ) ;
#30664=DIRECTION ( 'NONE',  ( -0.5000000000000038858, -0.8660254037844364872, 0.000000000000000000 ) ) ;
#30671=AXIS2_PLACEMENT_3D ( 'NONE', #37452, #39701, #21215 ) ;
#30672=DIRECTION ( 'NONE',  ( 0.5000000000000026645, 0.8660254037844372643, 0.000000000000000000 ) ) ;
#30674=DIRECTION ( 'NONE',  ( 0.3535533905932903287, 0.6123724356957876980, 0.7071067811865451302 ) ) ;
#30675=DIRECTION ( 'NONE',  ( 0.000000000000000000, 0.000000000000000000, -1.000000000000000000 ) ) ;
#30680=FACE_OUTER_BOUND ( 'NONE', #36988, .T. ) ;
#30681=ORIENTED_EDGE ( 'NONE', *, *, #37651, .T. ) ;
#30682=EDGE_LOOP ( 'NONE', ( #1656, #10937, #18290, #16592, #32750 ) ) ;
#30684=CARTESIAN_POINT ( 'NONE',  ( 1.000000000000000000, 37.00000000000000711, 10.50000000000000178 ) ) ;
#30685=AXIS2_PLACEMENT_3D ( 'NONE', #9194, #27286, #14897 ) ;
#30686=CARTESIAN_POINT ( 'NONE',  ( -7.111215932167764819, 17.81698729810783988, 9.000000000000001776 ) ) ;
#30687=ORIENTED_EDGE ( 'NONE', *, *, #33477, .T. ) ;
#30690=DIRECTION ( 'NONE',  ( -0.000000000000000000, 0.000000000000000000, 1.000000000000000000 ) ) ;
#30691=EDGE_CURVE ( 'NONE', #802, #39848, #29845, .T. ) ;
#30698=ORIENTED_EDGE ( 'NONE', *, *, #9857, .T. ) ;
#30703=VECTOR ( 'NONE', #20257, 1000.000000000000000 ) ;
#30704=LINE ( 'NONE', #21, #29807 ) ;
#30706=DIRECTION ( 'NONE',  ( -1.000000000000000000, 0.000000000000000000, 0.000000000000000000 ) ) ;
#30707=VECTOR ( 'NONE', #37262, 1000.000000000000000 ) ;
#30709=DIRECTION ( 'NONE',  ( 1.000000000000000000, 0.000000000000000000, 0.000000000000000000 ) ) ;
#30710=ADVANCED_FACE ( 'NONE', ( #13600 ), #19048, .T. ) ;
#30712=VECTOR ( 'NONE', #19495, 1000.000000000000000 ) ;
#30714=DIRECTION ( 'NONE',  ( 0.9781476007338067991, 0.2079116908177533474, -0.000000000000000000 ) ) ;
#30715=ADVANCED_FACE ( 'NONE', ( #23356 ), #23147, .T. ) ;
#30718=CARTESIAN_POINT ( 'NONE',  ( -12.97058434440066677, 15.58877990640330857, 10.96580508970284384 ) ) ;
#30719=PLANE ( 'NONE',  #35544 ) ;
#30723=EDGE_CURVE ( 'NONE', #8916, #38300, #25988, .T. ) ;
#30726=CARTESIAN_POINT ( 'NONE',  ( -3.553336972204574007, 8.187731063815915533, 10.94387467463493913 ) ) ;
#30735=DIRECTION ( 'NONE',  ( -0.000000000000000000, -0.000000000000000000, -1.000000000000000000 ) ) ;
#30738=CARTESIAN_POINT ( 'NONE',  ( -21.39877161664097827, 15.54711762656374141, 7.000000000000000000 ) ) ;
#30740=ADVANCED_FACE ( 'NONE', ( #35545 ), #25532, .T. ) ;
#30742=ADVANCED_FACE ( 'NONE', ( #38990 ), #4859, .T. ) ;
#30747=AXIS2_PLACEMENT_3D ( 'NONE', #2620, #5462, #5264 ) ;
#30753=DIRECTION ( 'NONE',  ( -0.000000000000000000, -0.000000000000000000, -1.000000000000000000 ) ) ;
#30754=AXIS2_PLACEMENT_3D ( 'NONE', #12902, #13093, #34643 ) ;
#30758=AXIS2_PLACEMENT_3D ( 'NONE', #6511, #8775, #33571 ) ;
#30760=EDGE_CURVE ( 'NONE', #15620, #9244, #17492, .T. ) ;
#30762=ORIENTED_EDGE ( 'NONE', *, *, #2234, .F. ) ;
#30770=AXIS2_PLACEMENT_3D ( 'NONE', #37291, #21843, #22046 ) ;
#30776=CARTESIAN_POINT ( 'NONE',  ( 0.000000000000000000, 22.50000000000000355, 0.000000000000000000 ) ) ;
#30779=FACE_OUTER_BOUND ( 'NONE', #37557, .T. ) ;
#30781=CARTESIAN_POINT ( 'NONE',  ( -8.796116341590805021, 23.42450908139092647, 9.000000000000001776 ) ) ;
#30783=VECTOR ( 'NONE', #32258, 1000.000000000000114 ) ;
#30785=DIRECTION ( 'NONE',  ( -0.000000000000000000, -0.000000000000000000, 1.000000000000000000 ) ) ;
#30787=VERTEX_POINT ( 'NONE', #16866 ) ;
#30789=DIRECTION ( 'NONE',  ( -0.2079116908177663647, -0.9781476007338042455, 0.000000000000000000 ) ) ;
#30790=CARTESIAN_POINT ( 'NONE',  ( 7.353987181296509412, 35.57359447655183970, 7.000000000000000000 ) ) ;
#30791=CARTESIAN_POINT ( 'NONE',  ( -10.73859285986284640, 31.49625607628545154, 7.500000000000004441 ) ) ;
#30794=EDGE_CURVE ( 'NONE', #3290, #36352, #32037, .T. ) ;
#30795=AXIS2_PLACEMENT_3D ( 'NONE', #35563, #17290, #4680 ) ;
#30797=LINE ( 'NONE', #11709, #30653 ) ;
#30799=ORIENTED_EDGE ( 'NONE', *, *, #38183, .F. ) ;
#30802=VECTOR ( 'NONE', #4356, 1000.000000000000000 ) ;
#30804=FACE_OUTER_BOUND ( 'NONE', #7322, .T. ) ;
#30805=LINE ( 'NONE', #2970, #3903 ) ;
#30806=LINE ( 'NONE', #6404, #8660 ) ;
#30808=ADVANCED_FACE ( 'NONE', ( #18266 ), #2227, .F. ) ;
#30811=CARTESIAN_POINT ( 'NONE',  ( 6.404490139165906371, 34.42612703509930583, 10.00000000000000000 ) ) ;
#30812=CARTESIAN_POINT ( 'NONE',  ( 7.118377661053320260, 10.47536095541698486, 7.000000000000000000 ) ) ;
#30814=DIRECTION ( 'NONE',  ( 1.000000000000000000, 0.000000000000000000, 0.000000000000000000 ) ) ;
#30815=AXIS2_PLACEMENT_3D ( 'NONE', #6663, #37758, #25164 ) ;
#30818=ORIENTED_EDGE ( 'NONE', *, *, #5915, .F. ) ;
#30821=CARTESIAN_POINT ( 'NONE',  ( 13.21633695260872976, 15.44689457190012227, 10.68306085400107541 ) ) ;
#30826=ORIENTED_EDGE ( 'NONE', *, *, #710, .F. ) ;
#30830=VECTOR ( 'NONE', #2973, 1000.000000000000114 ) ;
#30835=CARTESIAN_POINT ( 'NONE',  ( -1.653273178848928050E-15, 36.00000000000000711, 7.000000000000000000 ) ) ;
#30837=ORIENTED_EDGE ( 'NONE', *, *, #19484, .F. ) ;
#30840=ORIENTED_EDGE ( 'NONE', *, *, #25740, .T. ) ;
#30842=EDGE_CURVE ( 'NONE', #18489, #29040, #27596, .T. ) ;
#30846=AXIS2_PLACEMENT_3D ( 'NONE', #17096, #17901, #36179 ) ;
#30847=ADVANCED_FACE ( 'NONE', ( #36349 ), #27202, .T. ) ;
#30850=EDGE_LOOP ( 'NONE', ( #35222, #25019, #11705, #15847 ) ) ;
#30851=ADVANCED_FACE ( 'NONE', ( #36149 ), #17676, .F. ) ;
#30852=CARTESIAN_POINT ( 'NONE',  ( 11.11016527260166420, 31.83082137946473367, 9.000000000000001776 ) ) ;
#30853=AXIS2_PLACEMENT_3D ( 'NONE', #6812, #25709, #10477 ) ;
#30855=CIRCLE ( 'NONE', #1652, 15.00000000000000000 ) ;
#30856=AXIS2_PLACEMENT_3D ( 'NONE', #8590, #36820, #15284 ) ;
#30857=CARTESIAN_POINT ( 'NONE',  ( 13.95683075005237050, 28.08631143191933432, 10.50000000000000533 ) ) ;
#30860=CARTESIAN_POINT ( 'NONE',  ( -1.000000000000000888, 36.50000000000000711, 9.500000000000000000 ) ) ;
#30862=CARTESIAN_POINT ( 'NONE',  ( 3.161220354320216863, 12.43736188311278212, 10.49999999999999289 ) ) ;
#30866=ORIENTED_EDGE ( 'NONE', *, *, #16849, .T. ) ;
#30868=FACE_OUTER_BOUND ( 'NONE', #31183, .T. ) ;
#30877=DIRECTION ( 'NONE',  ( -0.4067366430757891060, 0.9135454576426058626, 1.734723475976806700E-15 ) ) ;
#30880=CARTESIAN_POINT ( 'NONE',  ( -14.86556419889029534, 20.43481210330121556, 10.49999999999999822 ) ) ;
#30881=CARTESIAN_POINT ( 'NONE',  ( -12.89070168820775386, 15.82735026918974341, 10.83333333333333037 ) ) ;
#30882=CONICAL_SURFACE ( 'NONE', #28263, 0.5000000000000002220, 0.7853981633974524978 ) ;
#30883=DIRECTION ( 'NONE',  ( -0.9945218953682745111, -0.1045284632676425907, 0.000000000000000000 ) ) ;
#30884=VERTEX_POINT ( 'NONE', #24148 ) ;
#30889=ORIENTED_EDGE ( 'NONE', *, *, #11888, .F. ) ;
#30891=ADVANCED_FACE ( 'NONE', ( #9113 ), #18461, .T. ) ;
#30892=DIRECTION ( 'NONE',  ( -0.000000000000000000, -0.000000000000000000, 1.000000000000000000 ) ) ;
#30893=ORIENTED_EDGE ( 'NONE', *, *, #24059, .T. ) ;
#30895=EDGE_LOOP ( 'NONE', ( #20333, #795, #28979 ) ) ;
#30902=EDGE_LOOP ( 'NONE', ( #33943, #19979, #7699, #35701 ) ) ;
#30904=CARTESIAN_POINT ( 'NONE',  ( -10.44103466624267185, 32.57396620494226624, 11.00000000000000000 ) ) ;
#30905=CARTESIAN_POINT ( 'NONE',  ( 3.713592597587208832, 7.966960743906818188, 7.000000000000000000 ) ) ;
#30906=VECTOR ( 'NONE', #38215, 1000.000000000000114 ) ;
#30909=VECTOR ( 'NONE', #8033, 1000.000000000000000 ) ;
#30910=CARTESIAN_POINT ( 'NONE',  ( 6.354454053420414361, 35.54304081427980577, 7.000000000000000000 ) ) ;
#30912=EDGE_CURVE ( 'NONE', #4851, #31336, #3017, .T. ) ;
#30913=EDGE_CURVE ( 'NONE', #37715, #15690, #31369, .T. ) ;
#30915=CARTESIAN_POINT ( 'NONE',  ( 8.306370210276320165, 9.993911548625739272, 10.49999999999999645 ) ) ;
#30916=DIRECTION ( 'NONE',  ( 0.4067366430758010409, 0.9135454576426005335, -0.000000000000000000 ) ) ;
#30917=CARTESIAN_POINT ( 'NONE',  ( 0.9028139003476853830, 37.47297129542256755, 7.381627713044571770 ) ) ;
#30922=CARTESIAN_POINT ( 'NONE',  ( -4.002483478063582290, 8.479530061156673071, 10.49999999999999822 ) ) ;
#30923=ORIENTED_EDGE ( 'NONE', *, *, #29321, .F. ) ;
#30932=CARTESIAN_POINT ( 'NONE',  ( -9.303655249773276736, 10.73386218874833631, 7.500000000000000888 ) ) ;
#30933=ORIENTED_EDGE ( 'NONE', *, *, #3071, .F. ) ;
#30935=DIRECTION ( 'NONE',  ( 0.000000000000000000, 1.000000000000000000, 0.000000000000000000 ) ) ;
#30936=CARTESIAN_POINT ( 'NONE',  ( 3.992867117591230919, 8.524771480177550487, 10.49999999999999289 ) ) ;
#30937=VERTEX_POINT ( 'NONE', #11566 ) ;
#30939=EDGE_CURVE ( 'NONE', #1970, #18869, #5860, .T. ) ;
#30940=VERTEX_POINT ( 'NONE', #39588 ) ;
#30942=CIRCLE ( 'NONE', #14081, 0.5000000000000004441 ) ;
#30947=LINE ( 'NONE', #15699, #8509 ) ;
#30949=CARTESIAN_POINT ( 'NONE',  ( 8.401171878996485987, 21.11424711454080594, 7.000000000000000000 ) ) ;
#30950=CARTESIAN_POINT ( 'NONE',  ( -13.63581098909220479, 27.45627467658446008, 9.500000000000000000 ) ) ;
#30955=DIRECTION ( 'NONE',  ( 1.000000000000000000, -6.938893903907197612E-15, 0.000000000000000000 ) ) ;
#30957=DIRECTION ( 'NONE',  ( 0.6724985119639553810, -0.2185080122244117407, -0.7071067811865489050 ) ) ;
#30958=EDGE_CURVE ( 'NONE', #15928, #4057, #18066, .T. ) ;
#30960=AXIS2_PLACEMENT_3D ( 'NONE', #25232, #457, #12839 ) ;
#30964=CARTESIAN_POINT ( 'NONE',  ( -4.475131784526824141, 8.183115020678636498, 7.000000000000000000 ) ) ;
#30967=CARTESIAN_POINT ( 'NONE',  ( 13.28503138821879581, 15.53523575316139649, 7.000000000000000000 ) ) ;
#30968=ORIENTED_EDGE ( 'NONE', *, *, #19438, .F. ) ;
#30969=AXIS2_PLACEMENT_3D ( 'NONE', #5053, #39177, #35937 ) ;
#30971=DIRECTION ( 'NONE',  ( -0.6724985119639492748, 0.2185080122244156264, -0.7071067811865536790 ) ) ;
#30973=CARTESIAN_POINT ( 'NONE',  ( -12.49038105676665644, 14.13397459621567798, 10.50000000000000000 ) ) ;
#30974=VECTOR ( 'NONE', #33276, 1000.000000000000000 ) ;
#30975=VERTEX_POINT ( 'NONE', #14612 ) ;
#30978=CARTESIAN_POINT ( 'NONE',  ( 1.525645716490520387, 8.212903943950921715, 7.000000000000000000 ) ) ;
#30983=DIRECTION ( 'NONE',  ( -0.1045284632676566766, -0.9945218953682730678, 0.000000000000000000 ) ) ;
#30985=ORIENTED_EDGE ( 'NONE', *, *, #4164, .F. ) ;
#30989=CARTESIAN_POINT ( 'NONE',  ( 1.278175571583998860, 14.08178954835375940, 7.000000000000000000 ) ) ;
#30990=EDGE_CURVE ( 'NONE', #15434, #16182, #6079, .T. ) ;
#30992=ORIENTED_EDGE ( 'NONE', *, *, #26995, .T. ) ;
#30996=VECTOR ( 'NONE', #36483, 1000.000000000000000 ) ;
#30999=B_SPLINE_CURVE_WITH_KNOTS ( 'NONE', 3,
 ( #3080, #28260, #6910, #30917, #21758, #37801, #12420, #6120 ),
 .UNSPECIFIED., .F., .F.,
 ( 4, 2, 2, 4 ),
 ( 0.000000000000000000, 0.0002364868538934269395, 0.0004729737077868538791, 0.0009459474155737077582 ),
 .UNSPECIFIED. ) ;
#31002=AXIS2_PLACEMENT_3D ( 'NONE', #8144, #23786, #5694 ) ;
#31004=DIRECTION ( 'NONE',  ( 0.000000000000000000, 0.000000000000000000, 1.000000000000000000 ) ) ;
#31007=CARTESIAN_POINT ( 'NONE',  ( 14.75678334372855538, 20.44624543189430099, 10.82238861112334760 ) ) ;
#31008=LINE ( 'NONE', #28151, #16853 ) ;
#31010=CARTESIAN_POINT ( 'NONE',  ( 9.665073660139013256, 25.11464168560187460, 10.50000000000000533 ) ) ;
#31012=DIRECTION ( 'NONE',  ( -0.5877852522924807976, -0.8090169943749417891, 0.000000000000000000 ) ) ;
#31019=CARTESIAN_POINT ( 'NONE',  ( 11.87435565298210882, 15.06698729810772619, 7.499999999999997335 ) ) ;
#31024=EDGE_LOOP ( 'NONE', ( #28888, #13629, #28237, #28869 ) ) ;
#31028=VECTOR ( 'NONE', #19237, 1000.000000000000000 ) ;
#31034=DIRECTION ( 'NONE',  ( 0.8090169943749504489, 0.5877852522924690293, -0.000000000000000000 ) ) ;
#31036=VECTOR ( 'NONE', #12056, 1000.000000000000000 ) ;
#31037=VERTEX_POINT ( 'NONE', #16207 ) ;
#31040=ADVANCED_FACE ( 'NONE', ( #40185 ), #18660, .F. ) ;
#31041=AXIS2_PLACEMENT_3D ( 'NONE', #8547, #15040, #33350 ) ;
#31044=EDGE_CURVE ( 'NONE', #34387, #22937, #31052, .T. ) ;
#31045=CARTESIAN_POINT ( 'NONE',  ( -1.278175571584109660, 14.08178954835378427, 7.000000000000000000 ) ) ;
#31050=FACE_OUTER_BOUND ( 'NONE', #1986, .T. ) ;
#31052=LINE ( 'NONE', #18855, #11286 ) ;
#31055=LINE ( 'NONE', #30857, #38277 ) ;
#31056=ORIENTED_EDGE ( 'NONE', *, *, #37830, .T. ) ;
#31058=CARTESIAN_POINT ( 'NONE',  ( -9.221287281574667816, 10.65863771052209863, 10.49999999999999822 ) ) ;
#31059=CARTESIAN_POINT ( 'NONE',  ( 13.14827996435953494, 25.72067290776660897, 9.500000000000000000 ) ) ;
#31060=AXIS2_PLACEMENT_3D ( 'NONE', #10662, #16763, #29750 ) ;
#31061=CARTESIAN_POINT ( 'NONE',  ( 13.49038105676655164, 15.86602540378438064, 11.00000000000000000 ) ) ;
#31065=VERTEX_POINT ( 'NONE', #12751 ) ;
#31067=CARTESIAN_POINT ( 'NONE',  ( -8.007761790012255076, 9.776959832083379709, 11.00000000000000000 ) ) ;
#31069=FACE_OUTER_BOUND ( 'NONE', #3697, .T. ) ;
#31070=ADVANCED_FACE ( 'NONE', ( #3217 ), #3408, .F. ) ;
#31077=CARTESIAN_POINT ( 'NONE',  ( 5.644276917315955266, 36.40655018617680838, 10.59344459855566534 ) ) ;
#31078=EDGE_LOOP ( 'NONE', ( #9559, #27491, #9448, #5052, #37414, #34072, #26276, #5306, #4704, #7449, #31837, #29162, #22354, #24133, #37796, #31056, #28911, #7378, #23685, #8753, #19210, #33903, #24522, #13179, #38217, #20559, #27769, #26989, #10293, #17094, #1996, #23858, #28282, #12157, #24934, #20940, #12748, #11851, #31512, #32707, #32305, #27595, #3662, #14375, #33576, #9888 ) ) ;
#31080=FACE_OUTER_BOUND ( 'NONE', #11285, .T. ) ;
#31081=DIRECTION ( 'NONE',  ( 0.000000000000000000, 0.000000000000000000, 1.000000000000000000 ) ) ;
#31083=AXIS2_PLACEMENT_3D ( 'NONE', #5435, #33082, #5031 ) ;
#31084=LINE ( 'NONE', #30686, #6590 ) ;
#31089=AXIS2_PLACEMENT_3D ( 'NONE', #5712, #14662, #2275 ) ;
#31090=B_SPLINE_SURFACE_WITH_KNOTS ( 'NONE', 1, 3, ( 
 ( #790, #22320, #13173, #25568, #12976, #28418, #9741, #594, #39665, #22123 ),
 ( #28218, #398, #37767, #19079, #39858, #22514, #34924, #36818, #25366, #12779 ) ),
 .UNSPECIFIED., .F., .F., .F.,
 ( 2, 2 ),
 ( 4, 2, 2, 2, 4 ),
 ( 0.000000000000000000, 1.000000000000000000 ),
 ( 1.796630036486493109, 2.189329118185220580, 2.582028199883947828, 2.974727281582675076, 3.367426363281402768 ),
 .UNSPECIFIED. ) ;
#31091=VERTEX_POINT ( 'NONE', #25144 ) ;
#31093=LINE ( 'NONE', #21539, #32628 ) ;
#31096=VERTEX_POINT ( 'NONE', #21894 ) ;
#31098=ADVANCED_FACE ( 'NONE', ( #34689 ), #31838, .T. ) ;
#31100=CARTESIAN_POINT ( 'NONE',  ( -1.000000000000000000, 37.50000000000000711, 7.000000000000000000 ) ) ;
#31103=VERTEX_POINT ( 'NONE', #15407 ) ;
#31104=CARTESIAN_POINT ( 'NONE',  ( 3.542977516905554847, 8.236468469132553594, 10.96580508970283141 ) ) ;
#31107=CARTESIAN_POINT ( 'NONE',  ( 13.77067693704748308, 28.44713853003850801, 7.000000000000000000 ) ) ;
#31109=AXIS2_PLACEMENT_3D ( 'NONE', #22243, #326, #37501 ) ;
#31110=ADVANCED_FACE ( 'NONE', ( #28590 ), #12556, .F. ) ;
#31112=CARTESIAN_POINT ( 'NONE',  ( -7.929471891321299815, 25.60217271033470965, 9.000000000000001776 ) ) ;
#31113=CARTESIAN_POINT ( 'NONE',  ( -12.74038105676665289, 14.56698729810790027, 10.49999999999999822 ) ) ;
#31115=ORIENTED_EDGE ( 'NONE', *, *, #3618, .F. ) ;
#31119=EDGE_CURVE ( 'NONE', #15928, #17936, #35291, .T. ) ;
#31120=CARTESIAN_POINT ( 'NONE',  ( 4.003793312560324225, 8.307369216259063549, 10.49999999999999645 ) ) ;
#31123=ORIENTED_EDGE ( 'NONE', *, *, #2643, .T. ) ;
#31127=VERTEX_POINT ( 'NONE', #34297 ) ;
#31135=ORIENTED_EDGE ( 'NONE', *, *, #5610, .T. ) ;
#31137=VERTEX_POINT ( 'NONE', #3806 ) ;
#31139=CIRCLE ( 'NONE', #36336, 0.4999999999999988898 ) ;
#31143=ADVANCED_FACE ( 'NONE', ( #27993 ), #37936, .T. ) ;
#31144=ORIENTED_EDGE ( 'NONE', *, *, #36568, .F. ) ;
#31146=EDGE_CURVE ( 'NONE', #22179, #36577, #34497, .T. ) ;
#31147=AXIS2_PLACEMENT_3D ( 'NONE', #15409, #8919, #34301 ) ;
#31148=CARTESIAN_POINT ( 'NONE',  ( 5.440908595777814050, 35.94977745735560859, 9.000000000000001776 ) ) ;
#31149=CARTESIAN_POINT ( 'NONE',  ( 14.36830325120613239, 20.48707633493483371, 7.000000000000000000 ) ) ;
#31150=CARTESIAN_POINT ( 'NONE',  ( 3.399837471815457590, 8.909889435135580626, 7.499999999999991118 ) ) ;
#31151=CARTESIAN_POINT ( 'NONE',  ( -8.927394655428429360, 11.06314620770957013, 11.00000000000000000 ) ) ;
#31152=DIRECTION ( 'NONE',  ( 1.000000000000000000, 0.000000000000000000, 0.000000000000000000 ) ) ;
#31158=CARTESIAN_POINT ( 'NONE',  ( -12.53024597560957787, 27.62278594035707613, 10.50000000000000000 ) ) ;
#31164=DIRECTION ( 'NONE',  ( 1.000000000000000000, 0.000000000000000000, 0.000000000000000000 ) ) ;
#31167=DIRECTION ( 'NONE',  ( -0.2079116908177663647, -0.9781476007338042455, 0.000000000000000000 ) ) ;
#31173=ORIENTED_EDGE ( 'NONE', *, *, #33022, .T. ) ;
#31176=DIRECTION ( 'NONE',  ( 0.6916548014802308408, 0.1470157664651821627, 0.7071067811865456854 ) ) ;
#31178=ORIENTED_EDGE ( 'NONE', *, *, #29670, .T. ) ;
#31180=DIRECTION ( 'NONE',  ( -0.000000000000000000, -0.000000000000000000, -1.000000000000000000 ) ) ;
#31181=FACE_OUTER_BOUND ( 'NONE', #35963, .T. ) ;
#31182=DIRECTION ( 'NONE',  ( -0.9781476007338069101, -0.2079116908177532363, 0.000000000000000000 ) ) ;
#31183=EDGE_LOOP ( 'NONE', ( #34567, #11011, #28119, #5859, #15285 ) ) ;
#31188=CONICAL_SURFACE ( 'NONE', #28596, 0.4999999999999970024, 0.7853981633974447263 ) ;
#31189=EDGE_LOOP ( 'NONE', ( #738, #7994, #14001 ) ) ;
#31190=EDGE_CURVE ( 'NONE', #35341, #22029, #22487, .T. ) ;
#31192=CARTESIAN_POINT ( 'NONE',  ( 13.32151712420403555, 20.09434385051835292, 10.50000000000000000 ) ) ;
#31193=EDGE_LOOP ( 'NONE', ( #36530, #37015, #29961, #1854 ) ) ;
#31196=FACE_OUTER_BOUND ( 'NONE', #1804, .T. ) ;
#31197=CARTESIAN_POINT ( 'NONE',  ( 14.09933648065468503, 26.02968990214155198, 10.50000000000000533 ) ) ;
#31199=CARTESIAN_POINT ( 'NONE',  ( -6.354454053420242943, 35.54304081427989814, 11.00000000000000000 ) ) ;
#31201=DIRECTION ( 'NONE',  ( -0.3583679495453109265, -0.9335804264971976352, 5.551115123125782702E-17 ) ) ;
#31202=PLANE ( 'NONE',  #38094 ) ;
#31203=DIRECTION ( 'NONE',  ( 0.5877852522924796874, 0.8090169943749426773, -0.000000000000000000 ) ) ;
#31205=DIRECTION ( 'NONE',  ( 1.000000000000000000, 0.000000000000000000, 0.000000000000000000 ) ) ;
#31207=DIRECTION ( 'NONE',  ( 0.000000000000000000, 0.000000000000000000, -1.000000000000000000 ) ) ;
#31208=EDGE_LOOP ( 'NONE', ( #19925, #33111, #8394, #5892, #34459, #26059, #7513 ) ) ;
#31209=CIRCLE ( 'NONE', #705, 0.4999999999999986122 ) ;
#31211=CARTESIAN_POINT ( 'NONE',  ( -5.490944681523145299, 34.83286367817517259, 7.000000000000000000 ) ) ;
#31212=DIRECTION ( 'NONE',  ( 0.9945218953682729568, -0.1045284632676569958, 0.000000000000000000 ) ) ;
#31213=ADVANCED_FACE ( 'NONE', ( #20061 ), #38538, .T. ) ;
#31219=ORIENTED_EDGE ( 'NONE', *, *, #35003, .T. ) ;
#31220=DIRECTION ( 'NONE',  ( 1.000000000000000000, 0.000000000000000000, 0.000000000000000000 ) ) ;
#31223=ADVANCED_FACE ( 'NONE', ( #13549 ), #26348, .F. ) ;
#31228=DIRECTION ( 'NONE',  ( -0.000000000000000000, -0.000000000000000000, -1.000000000000000000 ) ) ;
#31229=CONICAL_SURFACE ( 'NONE', #9161, 0.9999999999999981126, 0.7853981633974562726 ) ;
#31230=ORIENTED_EDGE ( 'NONE', *, *, #20179, .F. ) ;
#31233=ORIENTED_EDGE ( 'NONE', *, *, #7069, .F. ) ;
#31234=DIRECTION ( 'NONE',  ( 0.5138379476002949975, 0.6345370204113977008, 0.5773502691896332806 ) ) ;
#31235=DIRECTION ( 'NONE',  ( 0.000000000000000000, 0.000000000000000000, 1.000000000000000000 ) ) ;
#31236=EDGE_CURVE ( 'NONE', #21311, #2857, #27513, .T. ) ;
#31240=EDGE_CURVE ( 'NONE', #19274, #21780, #8058, .T. ) ;
#31244=ORIENTED_EDGE ( 'NONE', *, *, #9844, .T. ) ;
#31246=VERTEX_POINT ( 'NONE', #20261 ) ;
#31247=CARTESIAN_POINT ( 'NONE',  ( 10.47804177580207607, 33.28010392086025604, 11.00000000000000000 ) ) ;
#31248=CARTESIAN_POINT ( 'NONE',  ( -0.4999999999999995559, 37.00000000000000711, 11.00000000000000000 ) ) ;
#31249=DIRECTION ( 'NONE',  ( -0.6691306063588662312, -0.7431448254773869166, 0.000000000000000000 ) ) ;
#31254=AXIS2_PLACEMENT_3D ( 'NONE', #35581, #7739, #20143 ) ;
#31255=CARTESIAN_POINT ( 'NONE',  ( -8.411683849014160330, 19.76687823897114882, 9.000000000000001776 ) ) ;
#31256=CARTESIAN_POINT ( 'NONE',  ( 10.36408355391611913, 20.65655971416340009, 10.75000000000000888 ) ) ;
#31258=DIRECTION ( 'NONE',  ( -0.9945218953682730678, 0.1045284632676569819, 0.000000000000000000 ) ) ;
#31263=EDGE_CURVE ( 'NONE', #15556, #12231, #9368, .T. ) ;
#31265=DIRECTION ( 'NONE',  ( 0.9781476007338069101, 0.2079116908177532641, 0.000000000000000000 ) ) ;
#31268=DIRECTION ( 'NONE',  ( 0.4067366430757905493, -0.9135454576426051965, 0.000000000000000000 ) ) ;
#31273=DIRECTION ( 'NONE',  ( 0.000000000000000000, 0.000000000000000000, 1.000000000000000000 ) ) ;
#31274=CARTESIAN_POINT ( 'NONE',  ( 5.440908595777817602, 35.94977745735560859, 11.00000000000000000 ) ) ;
#31275=B_SPLINE_CURVE_WITH_KNOTS ( 'NONE', 3,
 ( #30218, #2389, #14779, #34653, #37896, #9478, #31404, #19014 ),
 .UNSPECIFIED., .F., .F.,
 ( 4, 2, 2, 4 ),
 ( 0.000000000000000000, 0.0004726692273637104840, 0.0007090038410455680841, 0.0009453384547274256301 ),
 .UNSPECIFIED. ) ;
#31276=ORIENTED_EDGE ( 'NONE', *, *, #31386, .F. ) ;
#31278=CARTESIAN_POINT ( 'NONE',  ( 0.7609933293816413258, 37.44611345180491213, 10.49999999999999822 ) ) ;
#31279=DIRECTION ( 'NONE',  ( 1.000000000000000000, 0.000000000000000000, 0.000000000000000000 ) ) ;
#31280=DIRECTION ( 'NONE',  ( 1.000000000000000000, 0.000000000000000000, 0.000000000000000000 ) ) ;
#31284=AXIS2_PLACEMENT_3D ( 'NONE', #15347, #20859, #39731 ) ;
#31286=VERTEX_POINT ( 'NONE', #25738 ) ;
#31291=AXIS2_PLACEMENT_3D ( 'NONE', #8849, #15733, #22027 ) ;
#31292=CIRCLE ( 'NONE', #13769, 0.5000000000000004441 ) ;
#31293=ORIENTED_EDGE ( 'NONE', *, *, #5012, .F. ) ;
#31296=CARTESIAN_POINT ( 'NONE',  ( -1.591208726688853492, -0.2560543600718806490, 10.00000000000000000 ) ) ;
#31298=DIRECTION ( 'NONE',  ( -1.000000000000000000, 0.000000000000000000, 0.000000000000000000 ) ) ;
#31299=ORIENTED_EDGE ( 'NONE', *, *, #16593, .F. ) ;
#31300=AXIS2_PLACEMENT_3D ( 'NONE', #39051, #27065, #20779 ) ;
#31301=CARTESIAN_POINT ( 'NONE',  ( 3.992867117591230919, 8.524771480177550487, 11.00000000000000000 ) ) ;
#31303=CARTESIAN_POINT ( 'NONE',  ( 9.343266739736582949, 17.68301270189218855, 10.00000000000000000 ) ) ;
#31307=CARTESIAN_POINT ( 'NONE',  ( 6.151085731882510288, 35.08626808545850650, 9.500000000000000000 ) ) ;
#31308=DIRECTION ( 'NONE',  ( -1.000000000000000000, 0.000000000000000000, 0.000000000000000000 ) ) ;
#31309=ORIENTED_EDGE ( 'NONE', *, *, #1870, .F. ) ;
#31311=CIRCLE ( 'NONE', #30685, 0.5000000000000004441 ) ;
#31314=CARTESIAN_POINT ( 'NONE',  ( 2.568190708544436429, 12.82247983807081226, 10.00000000000000000 ) ) ;
#31316=ORIENTED_EDGE ( 'NONE', *, *, #29321, .T. ) ;
#31320=EDGE_LOOP ( 'NONE', ( #10599, #8499, #31676, #31299 ) ) ;
#31323=DIRECTION ( 'NONE',  ( -1.000000000000000000, 0.000000000000000000, 0.000000000000000000 ) ) ;
#31326=DIRECTION ( 'NONE',  ( -0.000000000000000000, -0.000000000000000000, -1.000000000000000000 ) ) ;
#31327=DIRECTION ( 'NONE',  ( 0.000000000000000000, 0.000000000000000000, -1.000000000000000000 ) ) ;
#31330=ORIENTED_EDGE ( 'NONE', *, *, #21652, .F. ) ;
#31333=DIRECTION ( 'NONE',  ( 1.000000000000000000, 3.469446951953622866E-15, 0.000000000000000000 ) ) ;
#31336=VERTEX_POINT ( 'NONE', #23501 ) ;
#31337=AXIS2_PLACEMENT_3D ( 'NONE', #30776, #21815, #37463 ) ;
#31339=LINE ( 'NONE', #15508, #36407 ) ;
#31343=CARTESIAN_POINT ( 'NONE',  ( 2.525645716490518833, 8.212903943950921715, 11.00000000000000000 ) ) ;
#31346=DIRECTION ( 'NONE',  ( -0.9781476007338041345, 0.2079116908177664202, 0.000000000000000000 ) ) ;
#31349=CARTESIAN_POINT ( 'NONE',  ( 7.111215932167701759, 17.81698729810774751, 9.000000000000001776 ) ) ;
#31354=VERTEX_POINT ( 'NONE', #10507 ) ;
#31357=ADVANCED_FACE ( 'NONE', ( #22888 ), #28792, .T. ) ;
#31358=COLOUR_RGB ( '', 0.09019608, 0.27058824, 0.51372549) ;
#31360=PLANE ( 'NONE',  #24379 ) ;
#31362=ORIENTED_EDGE ( 'NONE', *, *, #22155, .T. ) ;
#31364=ORIENTED_EDGE ( 'NONE', *, *, #8626, .F. ) ;
#31366=DIRECTION ( 'NONE',  ( 0.8090169943749505599, 0.5877852522924689183, 0.000000000000000000 ) ) ;
#31368=CARTESIAN_POINT ( 'NONE',  ( 12.05736835487432401, 14.38397459621550389, 10.49999999999999822 ) ) ;
#31369=CIRCLE ( 'NONE', #232, 0.4999999999999995559 ) ;
#31373=CARTESIAN_POINT ( 'NONE',  ( -12.30736835487442704, 14.81698729810789672, 9.000000000000001776 ) ) ;
#31375=ORIENTED_EDGE ( 'NONE', *, *, #3116, .T. ) ;
#31377=CYLINDRICAL_SURFACE ( 'NONE', #8930, 0.4999999999999986122 ) ;
#31378=DIRECTION ( 'NONE',  ( -0.8090169943749426773, 0.5877852522924796874, 0.000000000000000000 ) ) ;
#31379=DIRECTION ( 'NONE',  ( 0.000000000000000000, -0.000000000000000000, -1.000000000000000000 ) ) ;
#31380=VERTEX_POINT ( 'NONE', #19857 ) ;
#31383=CIRCLE ( 'NONE', #13864, 0.5000000000000004441 ) ;
#31386=EDGE_CURVE ( 'NONE', #1970, #36443, #32248, .T. ) ;
#31388=AXIS2_PLACEMENT_3D ( 'NONE', #33478, #30423, #9077 ) ;
#31389=CARTESIAN_POINT ( 'NONE',  ( 14.86556419889027048, 20.43481210330100240, 10.49999999999999822 ) ) ;
#31391=ORIENTED_EDGE ( 'NONE', *, *, #30268, .F. ) ;
#31392=DIRECTION ( 'NONE',  ( 0.5254827454987569535, 0.4731467892558117172, -0.7071067811865512365 ) ) ;
#31397=DIRECTION ( 'NONE',  ( -0.4067366430757888840, 0.9135454576426058626, 0.000000000000000000 ) ) ;
#31398=FACE_OUTER_BOUND ( 'NONE', #39631, .T. ) ;
#31401=CARTESIAN_POINT ( 'NONE',  ( -10.29511041547402073, 24.79362192464190073, 10.50000000000000533 ) ) ;
#31404=CARTESIAN_POINT ( 'NONE',  ( -6.724783417411255293, 35.90833771957834131, 7.485646746502371940 ) ) ;
#31407=CARTESIAN_POINT ( 'NONE',  ( -13.94482798346716201, 26.50521816028930999, 7.000000000000000000 ) ) ;
#31408=CIRCLE ( 'NONE', #13900, 1.000000000000002665 ) ;
#31409=CARTESIAN_POINT ( 'NONE',  ( -12.03571151536224271, 31.45218678977246896, 7.000000000000000000 ) ) ;
#31410=ADVANCED_FACE ( 'NONE', ( #29199 ), #13751, .F. ) ;
#31425=ORIENTED_EDGE ( 'NONE', *, *, #20205, .F. ) ;
#31429=ORIENTED_EDGE ( 'NONE', *, *, #11723, .T. ) ;
#31433=EDGE_LOOP ( 'NONE', ( #302, #32782, #38707, #13118 ) ) ;
#31434=CARTESIAN_POINT ( 'NONE',  ( 3.713592597587160871, 7.966960743906808418, 7.499999999999990230 ) ) ;
#31435=DIRECTION ( 'NONE',  ( 1.000000000000000000, 0.000000000000000000, 0.000000000000000000 ) ) ;
#31437=ADVANCED_FACE ( 'NONE', ( #27155 ), #33665, .F. ) ;
#31442=ORIENTED_EDGE ( 'NONE', *, *, #11269, .T. ) ;
#31444=CARTESIAN_POINT ( 'NONE',  ( 15.00099999999999767, 36.50000000000000711, 7.000000000000000000 ) ) ;
#31446=AXIS2_PLACEMENT_3D ( 'NONE', #25956, #22504, #19666 ) ;
#31447=CARTESIAN_POINT ( 'NONE',  ( 13.62380822250710999, 25.87518140495407692, 10.50000000000000000 ) ) ;
#31448=ORIENTED_EDGE ( 'NONE', *, *, #33524, .T. ) ;
#31451=LINE ( 'NONE', #33911, #9205 ) ;
#31452=DIRECTION ( 'NONE',  ( 0.2079116908177534029, -0.9781476007338067991, 0.000000000000000000 ) ) ;
#31453=DIRECTION ( 'NONE',  ( 0.07391278520358296467, 0.7032331762533997610, -0.7071067811865502373 ) ) ;
#31454=DIRECTION ( 'NONE',  ( -0.9945218953682730678, 0.1045284632676569819, 0.000000000000000000 ) ) ;
#31457=VERTEX_POINT ( 'NONE', #14561 ) ;
#31461=CARTESIAN_POINT ( 'NONE',  ( -13.16028273094462975, 27.30176617939698147, 10.00000000000000000 ) ) ;
#31463=EDGE_CURVE ( 'NONE', #15902, #14950, #39201, .T. ) ;
#31465=DIRECTION ( 'NONE',  ( 0.8090169943749426773, -0.5877852522924797984, 0.000000000000000000 ) ) ;
#31471=CARTESIAN_POINT ( 'NONE',  ( 8.229154955994852472, 10.32288908946079076, 10.96580508970283141 ) ) ;
#31472=CARTESIAN_POINT ( 'NONE',  ( 5.465749975257575777, 36.45564430483320706, 10.49999999999999822 ) ) ;
#31473=VERTEX_POINT ( 'NONE', #14960 ) ;
#31475=DIRECTION ( 'NONE',  ( -0.4156269377774530760, 0.5720614028176880250, -0.7071067811865446862 ) ) ;
#31477=CARTESIAN_POINT ( 'NONE',  ( -11.81630298851966288, 31.79381426990562787, 10.50000000000000000 ) ) ;
#31480=CARTESIAN_POINT ( 'NONE',  ( 4.591666147298500533, 15.32946292166668556, 9.000000000000001776 ) ) ;
#31481=CARTESIAN_POINT ( 'NONE',  ( -7.766013557953294288, 28.81973365084998306, 10.50000000000000000 ) ) ;
#31483=VECTOR ( 'NONE', #30172, 1000.000000000000000 ) ;
#31487=VERTEX_POINT ( 'NONE', #8668 ) ;
#31489=CONICAL_SURFACE ( 'NONE', #374, 1.000000000000014655, 0.7853981633974520538 ) ;
#31491=EDGE_CURVE ( 'NONE', #30787, #24743, #36701, .T. ) ;
#31494=DIRECTION ( 'NONE',  ( -0.5254827454987639479, -0.4731467892558146593, -0.7071067811865439090 ) ) ;
#31500=DIRECTION ( 'NONE',  ( 0.9781476007338069101, 0.2079116908177532641, -0.000000000000000000 ) ) ;
#31502=CARTESIAN_POINT ( 'NONE',  ( 5.440908595777814050, 35.94977745735560859, 7.000000000000000000 ) ) ;
#31503=DIRECTION ( 'NONE',  ( -1.000000000000000000, 0.000000000000000000, 0.000000000000000000 ) ) ;
#31506=ORIENTED_EDGE ( 'NONE', *, *, #24897, .T. ) ;
#31510=CARTESIAN_POINT ( 'NONE',  ( -14.02783499842349002, 22.03112340962126581, 10.50000000000000000 ) ) ;
#31511=EDGE_CURVE ( 'NONE', #10646, #37532, #28538, .T. ) ;
#31512=ORIENTED_EDGE ( 'NONE', *, *, #39373, .T. ) ;
#31513=AXIS2_PLACEMENT_3D ( 'NONE', #14374, #7672, #38956 ) ;
#31518=DIRECTION ( 'NONE',  ( 0.000000000000000000, 0.000000000000000000, 1.000000000000000000 ) ) ;
#31519=ORIENTED_EDGE ( 'NONE', *, *, #3846, .T. ) ;
#31520=ORIENTED_EDGE ( 'NONE', *, *, #1677, .T. ) ;
#31522=CARTESIAN_POINT ( 'NONE',  ( -7.659620408498105881, 26.92228390473685096, 9.000000000000001776 ) ) ;
#31526=CARTESIAN_POINT ( 'NONE',  ( -20.23249103036706842, 12.99895069675662640, 9.500000000000000000 ) ) ;
#31527=ORIENTED_EDGE ( 'NONE', *, *, #15478, .F. ) ;
#31529=DIRECTION ( 'NONE',  ( 0.000000000000000000, 0.000000000000000000, 1.000000000000000000 ) ) ;
#31530=LINE ( 'NONE', #33796, #24494 ) ;
#31531=ORIENTED_EDGE ( 'NONE', *, *, #34357, .T. ) ;
#31533=ORIENTED_EDGE ( 'NONE', *, *, #38926, .T. ) ;
#31537=EDGE_CURVE ( 'NONE', #28022, #29830, #24102, .T. ) ;
#31538=ORIENTED_EDGE ( 'NONE', *, *, #367, .T. ) ;
#31539=CIRCLE ( 'NONE', #18583, 0.4999999999999997780 ) ;
#31542=CARTESIAN_POINT ( 'NONE',  ( -7.929471891321299815, 25.60217271033470965, 9.000000000000001776 ) ) ;
#31543=AXIS2_PLACEMENT_3D ( 'NONE', #19069, #16020, #12767 ) ;
#31544=CARTESIAN_POINT ( 'NONE',  ( -2.916683454136887121, 12.38538396040838840, 10.75000000000001776 ) ) ;
#31551=ORIENTED_EDGE ( 'NONE', *, *, #688, .F. ) ;
#31554=DIRECTION ( 'NONE',  ( 1.000000000000000000, 0.000000000000000000, 0.000000000000000000 ) ) ;
#31556=ORIENTED_EDGE ( 'NONE', *, *, #36199, .T. ) ;
#31557=ADVANCED_FACE ( 'NONE', ( #30606 ), #39933, .F. ) ;
#31558=CARTESIAN_POINT ( 'NONE',  ( -13.97557076678966403, 21.53386246193713305, 7.500000000000004441 ) ) ;
#31559=EDGE_LOOP ( 'NONE', ( #13946, #17687, #8944, #10446 ) ) ;
#31561=CARTESIAN_POINT ( 'NONE',  ( 14.97283171447379146, 21.48159823030311344, 7.000000000000000000 ) ) ;
#31564=CIRCLE ( 'NONE', #17324, 0.5000000000000004441 ) ;
#31565=ORIENTED_EDGE ( 'NONE', *, *, #17341, .F. ) ;
#31568=CARTESIAN_POINT ( 'NONE',  ( -5.288651019503864958, 36.01756689786831345, 10.83333333333333215 ) ) ;
#31570=ORIENTED_EDGE ( 'NONE', *, *, #26713, .F. ) ;
#31572=CARTESIAN_POINT ( 'NONE',  ( -21.39877161664097827, 15.54711762656374141, 7.000000000000000000 ) ) ;
#31573=FACE_OUTER_BOUND ( 'NONE', #26007, .T. ) ;
#31575=ORIENTED_EDGE ( 'NONE', *, *, #1712, .F. ) ;
#31579=EDGE_LOOP ( 'NONE', ( #2545, #11827, #1201, #26787, #30176, #28136, #34682, #13460 ) ) ;
#31582=VERTEX_POINT ( 'NONE', #39737 ) ;
#31586=PLANE ( 'NONE',  #7798 ) ;
#31591=LINE ( 'NONE', #6407, #9148 ) ;
#31594=FACE_OUTER_BOUND ( 'NONE', #22100, .T. ) ;
#31595=DIRECTION ( 'NONE',  ( -1.000000000000000000, 0.000000000000000000, 0.000000000000000000 ) ) ;
#31597=AXIS2_PLACEMENT_3D ( 'NONE', #30214, #14164, #11328 ) ;
#31598=PLANE ( 'NONE',  #2262 ) ;
#31599=VERTEX_POINT ( 'NONE', #39136 ) ;
#31609=EDGE_LOOP ( 'NONE', ( #3888, #2708, #38422 ) ) ;
#31610=CARTESIAN_POINT ( 'NONE',  ( -14.86556419889029534, 20.43481210330121556, 11.00000000000000000 ) ) ;
#31611=EDGE_CURVE ( 'NONE', #14430, #2539, #2869, .T. ) ;
#31618=ORIENTED_EDGE ( 'NONE', *, *, #33612, .F. ) ;
#31620=CARTESIAN_POINT ( 'NONE',  ( -9.062230821157587712, 11.16111041642498591, 10.83333333333333215 ) ) ;
#31621=EDGE_CURVE ( 'NONE', #21433, #172, #24898, .T. ) ;
#31622=B_SPLINE_CURVE_WITH_KNOTS ( 'NONE', 3,
 ( #7309, #20921, #30065, #17887, #8333, #33124 ),
 .UNSPECIFIED., .F., .F.,
 ( 4, 2, 4 ),
 ( 0.000000000000000000, 0.5000000000000000000, 1.000000000000000000 ),
 .UNSPECIFIED. ) ;
#31627=CIRCLE ( 'NONE', #13462, 0.5000000000000004441 ) ;
#31629=EDGE_LOOP ( 'NONE', ( #28273, #25624, #12674, #37223, #35851 ) ) ;
#31630=DIRECTION ( 'NONE',  ( -0.000000000000000000, -0.000000000000000000, -1.000000000000000000 ) ) ;
#31632=AXIS2_PLACEMENT_3D ( 'NONE', #34837, #16555, #3748 ) ;
#31636=VECTOR ( 'NONE', #16036, 999.9999999999998863 ) ;
#31638=EDGE_CURVE ( 'NONE', #26640, #21617, #22235, .T. ) ;
#31639=ORIENTED_EDGE ( 'NONE', *, *, #892, .T. ) ;
#31643=PLANE ( 'NONE',  #33103 ) ;
#31646=CARTESIAN_POINT ( 'NONE',  ( -19.34689456777905292, 35.00980436007201746, 10.00000000000000000 ) ) ;
#31647=DIRECTION ( 'NONE',  ( -0.5720614028176770338, 0.4156269377774552409, 0.7071067811865524577 ) ) ;
#31648=B_SPLINE_CURVE_WITH_KNOTS ( 'NONE', 3,
 ( #14863, #24002, #32963, #30509 ),
 .UNSPECIFIED., .F., .F.,
 ( 4, 4 ),
 ( 0.000000000000000000, 0.1333333595060078314 ),
 .UNSPECIFIED. ) ;
#31650=LINE ( 'NONE', #10118, #30570 ) ;
#31651=DIRECTION ( 'NONE',  ( -0.000000000000000000, -0.000000000000000000, -1.000000000000000000 ) ) ;
#31652=CARTESIAN_POINT ( 'NONE',  ( 2.552861293176707402, 8.084864722426264194, 11.00000000000000355 ) ) ;
#31655=LINE ( 'NONE', #38147, #20509 ) ;
#31656=AXIS2_PLACEMENT_3D ( 'NONE', #18986, #24483, #12488 ) ;
#31657=ORIENTED_EDGE ( 'NONE', *, *, #37797, .F. ) ;
#31659=CARTESIAN_POINT ( 'NONE',  ( -12.22403502154109667, 14.67264973081049284, 10.83333333333333037 ) ) ;
#31662=LINE ( 'NONE', #28210, #2913 ) ;
#31665=ADVANCED_FACE ( 'NONE', ( #30804 ), #8056, .T. ) ;
#31666=DIRECTION ( 'NONE',  ( 0.7431448254773953543, 0.6691306063588570163, 0.000000000000000000 ) ) ;
#31671=CARTESIAN_POINT ( 'NONE',  ( 8.336672018935502138, 10.01592710129210850, 10.49999999999999822 ) ) ;
#31672=CARTESIAN_POINT ( 'NONE',  ( 5.517564457587568860, 36.12194934191559526, 10.96580508970282608 ) ) ;
#31673=ORIENTED_EDGE ( 'NONE', *, *, #19587, .T. ) ;
#31675=CARTESIAN_POINT ( 'NONE',  ( -13.87104230352202094, 20.53934056656885687, 7.500000000000004441 ) ) ;
#31676=ORIENTED_EDGE ( 'NONE', *, *, #33999, .F. ) ;
#31678=CARTESIAN_POINT ( 'NONE',  ( 8.927394655428274817, 11.06314620770945290, 7.500000000000000888 ) ) ;
#31680=ORIENTED_EDGE ( 'NONE', *, *, #5943, .F. ) ;
#31682=CARTESIAN_POINT ( 'NONE',  ( -7.530592408761007661, 11.28437794979203090, 10.00000000000000000 ) ) ;
#31683=ORIENTED_EDGE ( 'NONE', *, *, #25025, .T. ) ;
#31685=VECTOR ( 'NONE', #28380, 1000.000000000000000 ) ;
#31686=AXIS2_PLACEMENT_3D ( 'NONE', #1304, #38475, #27089 ) ;
#31691=DIRECTION ( 'NONE',  ( -0.5877852522924690293, 0.8090169943749503378, 0.000000000000000000 ) ) ;
#31692=CARTESIAN_POINT ( 'NONE',  ( -0.7619526660190145684, 37.48079653017162371, 7.455686640544901600 ) ) ;
#31693=EDGE_CURVE ( 'NONE', #5336, #24444, #16155, .T. ) ;
#31695=VECTOR ( 'NONE', #1771, 1000.000000000000000 ) ;
#31696=CYLINDRICAL_SURFACE ( 'NONE', #18797, 0.5000000000000004441 ) ;
#31700=CARTESIAN_POINT ( 'NONE',  ( 12.67493120981675325, 14.45362483784307983, 10.49999999999999645 ) ) ;
#31706=LINE ( 'NONE', #37209, #21277 ) ;
#31708=CIRCLE ( 'NONE', #568, 1.000000000000002665 ) ;
#31709=ORIENTED_EDGE ( 'NONE', *, *, #3564, .F. ) ;
#31711=AXIS2_PLACEMENT_3D ( 'NONE', #29482, #36186, #4902 ) ;
#31714=EDGE_CURVE ( 'NONE', #27240, #18790, #20395, .T. ) ;
#31715=DIRECTION ( 'NONE',  ( 1.000000000000000000, 0.000000000000000000, 0.000000000000000000 ) ) ;
#31717=VERTEX_POINT ( 'NONE', #320 ) ;
#31718=AXIS2_PLACEMENT_3D ( 'NONE', #13654, #38036, #11023 ) ;
#31722=EDGE_CURVE ( 'NONE', #39789, #13016, #6792, .T. ) ;
#31724=CYLINDRICAL_SURFACE ( 'NONE', #25474, 0.5000000000000011102 ) ;
#31727=CARTESIAN_POINT ( 'NONE',  ( 14.19304739008519256, 26.58586953448655521, 10.94611345180491035 ) ) ;
#31728=CARTESIAN_POINT ( 'NONE',  ( 14.97277451176449325, 21.48159783397873923, 10.49999999999999822 ) ) ;
#31732=ORIENTED_EDGE ( 'NONE', *, *, #18761, .F. ) ;
#31734=CARTESIAN_POINT ( 'NONE',  ( -13.42604558747169285, 21.08886574588681384, 7.000000000000000000 ) ) ;
#31736=ORIENTED_EDGE ( 'NONE', *, *, #11770, .T. ) ;
#31739=EDGE_CURVE ( 'NONE', #11008, #23024, #33365, .T. ) ;
#31744=VECTOR ( 'NONE', #36718, 1000.000000000000114 ) ;
#31746=CARTESIAN_POINT ( 'NONE',  ( 10.14060191828659541, 25.26915018278934610, 11.00000000000000000 ) ) ;
#31747=AXIS2_PLACEMENT_3D ( 'NONE', #10765, #20114, #14008 ) ;
#31753=FACE_OUTER_BOUND ( 'NONE', #18607, .T. ) ;
#31754=EDGE_CURVE ( 'NONE', #4170, #24423, #3359, .T. ) ;
#31756=ORIENTED_EDGE ( 'NONE', *, *, #22897, .F. ) ;
#31759=EDGE_CURVE ( 'NONE', #39078, #2539, #37881, .T. ) ;
#31762=ORIENTED_EDGE ( 'NONE', *, *, #3462, .F. ) ;
#31764=FACE_OUTER_BOUND ( 'NONE', #4804, .T. ) ;
#31767=CARTESIAN_POINT ( 'NONE',  ( 7.748046928843868031, 9.655464433119462342, 7.102474990965862212 ) ) ;
#31769=DIRECTION ( 'NONE',  ( -0.3090169943749560000, -0.9510565162951507556, -3.469446951953612611E-15 ) ) ;
#31774=DIRECTION ( 'NONE',  ( 0.000000000000000000, 0.000000000000000000, 1.000000000000000000 ) ) ;
#31776=VERTEX_POINT ( 'NONE', #37492 ) ;
#31778=CARTESIAN_POINT ( 'NONE',  ( -7.713869163866014844, 10.18146832927085299, 9.500000000000000000 ) ) ;
#31780=DIRECTION ( 'NONE',  ( 1.000000000000000000, 0.000000000000000000, 0.000000000000000000 ) ) ;
#31787=DIRECTION ( 'NONE',  ( 0.000000000000000000, -0.000000000000000000, -1.000000000000000000 ) ) ;
#31789=ADVANCED_FACE ( 'NONE', ( #9670 ), #28335, .F. ) ;
#31791=DIRECTION ( 'NONE',  ( -0.7431448254773862505, 0.6691306063588670083, 0.000000000000000000 ) ) ;
#31792=CARTESIAN_POINT ( 'NONE',  ( -6.811226782241547539, 35.33967249274200384, 9.500000000000000000 ) ) ;
#31795=FACE_OUTER_BOUND ( 'NONE', #20745, .T. ) ;
#31798=CIRCLE ( 'NONE', #18189, 15.00000000000000000 ) ;
#31800=LINE ( 'NONE', #29158, #17741 ) ;
#31802=CARTESIAN_POINT ( 'NONE',  ( -4.678013043399448456, 44.50832101651065642, 7.000000000000000000 ) ) ;
#31805=CARTESIAN_POINT ( 'NONE',  ( -3.503793317224518145, 8.420815634768723967, 7.499999999999997335 ) ) ;
#31806=CARTESIAN_POINT ( 'NONE',  ( 13.01373512357458928, 15.56386679243127347, 10.94387467463492847 ) ) ;
#31808=CARTESIAN_POINT ( 'NONE',  ( 13.47830981910550641, 21.58612669357077607, 7.000000000000000000 ) ) ;
#31810=ORIENTED_EDGE ( 'NONE', *, *, #29002, .T. ) ;
#31812=VERTEX_POINT ( 'NONE', #24698 ) ;
#31814=CARTESIAN_POINT ( 'NONE',  ( 12.99377146717206344, 26.19620116591418224, 9.500000000000000000 ) ) ;
#31817=CIRCLE ( 'NONE', #37011, 0.5000000000000004441 ) ;
#31821=ORIENTED_EDGE ( 'NONE', *, *, #8830, .F. ) ;
#31825=ORIENTED_EDGE ( 'NONE', *, *, #23489, .T. ) ;
#31828=ORIENTED_EDGE ( 'NONE', *, *, #2599, .T. ) ;
#31829=B_SPLINE_CURVE_WITH_KNOTS ( 'NONE', 3,
 ( #24795, #21546, #24997, #13194, #19294, #31692, #27846, #36993 ),
 .UNSPECIFIED., .F., .F.,
 ( 4, 2, 2, 4 ),
 ( 2.168404344971008868E-19, 0.0004726692273637090745, 0.0007090038410455647231, 0.0009453384547274204259 ),
 .UNSPECIFIED. ) ;
#31831=DIRECTION ( 'NONE',  ( -0.1045284632676569819, -0.9945218953682730678, 0.000000000000000000 ) ) ;
#31832=AXIS2_PLACEMENT_3D ( 'NONE', #18517, #9170, #34358 ) ;
#31837=ORIENTED_EDGE ( 'NONE', *, *, #3147, .T. ) ;
#31838=PLANE ( 'NONE',  #4131 ) ;
#31840=AXIS2_PLACEMENT_3D ( 'NONE', #33768, #15060, #3070 ) ;
#31848=EDGE_CURVE ( 'NONE', #33983, #31959, #39041, .T. ) ;
#31849=DIRECTION ( 'NONE',  ( -0.3090169943749450643, 0.9510565162951543083, 0.000000000000000000 ) ) ;
#31850=CARTESIAN_POINT ( 'NONE',  ( -14.49025312501840723, 21.64735187953135309, 10.83333333333333215 ) ) ;
#31853=FACE_OUTER_BOUND ( 'NONE', #23298, .T. ) ;
#31856=CARTESIAN_POINT ( 'NONE',  ( 13.14827996435953494, 25.72067290776660897, 10.50000000000000000 ) ) ;
#31859=DIRECTION ( 'NONE',  ( 0.4156269377774525209, 0.5720614028176911336, -0.7071067811865425767 ) ) ;
#31867=EDGE_CURVE ( 'NONE', #6401, #13649, #34839, .T. ) ;
#31871=VERTEX_POINT ( 'NONE', #10253 ) ;
#31872=B_SPLINE_CURVE_WITH_KNOTS ( 'NONE', 3,
 ( #21584, #2704, #21192, #33985 ),
 .UNSPECIFIED., .F., .F.,
 ( 4, 4 ),
 ( 0.000000000000000000, 1.000000000000000000 ),
 .UNSPECIFIED. ) ;
#31878=AXIS2_PLACEMENT_3D ( 'NONE', #35600, #35396, #17321 ) ;
#31879=CARTESIAN_POINT ( 'NONE',  ( 0.5000000000000001110, 37.00000000000000711, 9.000000000000001776 ) ) ;
#31880=LINE ( 'NONE', #4041, #23253 ) ;
#31884=VERTEX_POINT ( 'NONE', #20772 ) ;
#31886=ORIENTED_EDGE ( 'NONE', *, *, #22508, .F. ) ;
#31888=DIRECTION ( 'NONE',  ( 0.9781476007338072431, 0.2079116908177517375, 0.000000000000000000 ) ) ;
#31889=DIRECTION ( 'NONE',  ( -0.000000000000000000, -0.000000000000000000, -1.000000000000000000 ) ) ;
#31890=PLANE ( 'NONE',  #3345 ) ;
#31893=DIRECTION ( 'NONE',  ( -0.000000000000000000, -0.000000000000000000, -1.000000000000000000 ) ) ;
#31896=DIRECTION ( 'NONE',  ( 1.000000000000000000, 0.000000000000000000, 0.000000000000000000 ) ) ;
#31897=CARTESIAN_POINT ( 'NONE',  ( -6.354454053420248272, 35.54304081427989814, 9.000000000000001776 ) ) ;
#31901=ORIENTED_EDGE ( 'NONE', *, *, #14006, .T. ) ;
#31904=LINE ( 'NONE', #19720, #22353 ) ;
#31912=EDGE_CURVE ( 'NONE', #8749, #14728, #4154, .T. ) ;
#31916=CARTESIAN_POINT ( 'NONE',  ( -6.557822374958137246, 35.99981354310120452, 10.63089969389957012 ) ) ;
#31919=DIRECTION ( 'NONE',  ( 0.000000000000000000, 0.000000000000000000, 1.000000000000000000 ) ) ;
#31920=EDGE_LOOP ( 'NONE', ( #29649, #18526, #21269, #39222, #4760 ) ) ;
#31922=DIRECTION ( 'NONE',  ( 1.000000000000000000, 0.000000000000000000, 0.000000000000000000 ) ) ;
#31923=CARTESIAN_POINT ( 'NONE',  ( 13.05736835487433467, 16.11602540378438420, 10.49999999999999822 ) ) ;
#31926=CARTESIAN_POINT ( 'NONE',  ( -5.465749975257388371, 36.45564430483327811, 10.49999999999999822 ) ) ;
#31927=ORIENTED_EDGE ( 'NONE', *, *, #7482, .T. ) ;
#31929=DIRECTION ( 'NONE',  ( -0.000000000000000000, -0.000000000000000000, -1.000000000000000000 ) ) ;
#31930=VECTOR ( 'NONE', #3915, 1000.000000000000114 ) ;
#31934=CARTESIAN_POINT ( 'NONE',  ( -10.81260707898136708, 32.90853150812170469, 7.000000000000000000 ) ) ;
#31935=EDGE_CURVE ( 'NONE', #19575, #855, #2081, .T. ) ;
#31937=CARTESIAN_POINT ( 'NONE',  ( -23.14043693410022229, 26.33379778550221673, 10.00000000000000000 ) ) ;
#31940=DIRECTION ( 'NONE',  ( 0.000000000000000000, 0.000000000000000000, -1.000000000000000000 ) ) ;
#31942=VECTOR ( 'NONE', #595, 1000.000000000000000 ) ;
#31947=DIRECTION ( 'NONE',  ( 0.9781476007338042455, -0.2079116908177663370, -0.000000000000000000 ) ) ;
#31959=VERTEX_POINT ( 'NONE', #36209 ) ;
#31961=CARTESIAN_POINT ( 'NONE',  ( 8.014845354181460380, 9.820632123551975567, 7.338691926023214407 ) ) ;
#31962=EDGE_CURVE ( 'NONE', #21971, #5904, #10020, .T. ) ;
#31964=CARTESIAN_POINT ( 'NONE',  ( 12.74038105676654631, 14.56698729810771731, 10.49999999999999822 ) ) ;
#31965=EDGE_CURVE ( 'NONE', #2211, #3294, #27547, .T. ) ;
#31972=ORIENTED_EDGE ( 'NONE', *, *, #797, .F. ) ;
#31976=CARTESIAN_POINT ( 'NONE',  ( -4.727507481117092070, 31.88885898370948269, 10.50000000000000000 ) ) ;
#31977=ORIENTED_EDGE ( 'NONE', *, *, #31714, .T. ) ;
#31983=EDGE_CURVE ( 'NONE', #21143, #17826, #38287, .T. ) ;
#31984=AXIS2_PLACEMENT_3D ( 'NONE', #16365, #725, #35253 ) ;
#31985=DIRECTION ( 'NONE',  ( -0.000000000000000000, -0.000000000000000000, -1.000000000000000000 ) ) ;
#31986=ADVANCED_FACE ( 'NONE', ( #22840 ), #8727, .T. ) ;
#31987=FACE_OUTER_BOUND ( 'NONE', #35541, .T. ) ;
#31988=EDGE_CURVE ( 'NONE', #37754, #2697, #35240, .T. ) ;
#31990=CIRCLE ( 'NONE', #27446, 6.000000000000013323 ) ;
#31992=FACE_OUTER_BOUND ( 'NONE', #15887, .T. ) ;
#31995=ORIENTED_EDGE ( 'NONE', *, *, #6439, .T. ) ;
#31996=FACE_OUTER_BOUND ( 'NONE', #14909, .T. ) ;
#32003=CARTESIAN_POINT ( 'NONE',  ( -10.73859285986284640, 31.49625607628545154, 7.500000000000005329 ) ) ;
#32009=DIRECTION ( 'NONE',  ( 1.000000000000000000, 5.204170427930407084E-15, 0.000000000000000000 ) ) ;
#32011=ORIENTED_EDGE ( 'NONE', *, *, #39347, .F. ) ;
#32013=ORIENTED_EDGE ( 'NONE', *, *, #10369, .F. ) ;
#32015=CARTESIAN_POINT ( 'NONE',  ( 3.503793317224320969, 8.420815634768672453, 11.00000000000000000 ) ) ;
#32019=EDGE_CURVE ( 'NONE', #11801, #30503, #5912, .T. ) ;
#32021=CIRCLE ( 'NONE', #30754, 0.4999999999999999445 ) ;
#32024=VERTEX_POINT ( 'NONE', #37198 ) ;
#32029=ORIENTED_EDGE ( 'NONE', *, *, #32599, .T. ) ;
#32034=CARTESIAN_POINT ( 'NONE',  ( -14.35088184066156280, 20.32132268570699196, 10.83333333333333393 ) ) ;
#32037=CIRCLE ( 'NONE', #30747, 0.5000000000000001110 ) ;
#32041=DIRECTION ( 'NONE',  ( -0.8660254037844454800, -0.4999999999999881206, 0.000000000000000000 ) ) ;
#32044=ORIENTED_EDGE ( 'NONE', *, *, #25566, .F. ) ;
#32045=AXIS2_PLACEMENT_3D ( 'NONE', #27061, #36405, #14872 ) ;
#32050=CARTESIAN_POINT ( 'NONE',  ( 5.537946624086096392, 36.44027069998188750, 7.500000000000000888 ) ) ;
#32051=CARTESIAN_POINT ( 'NONE',  ( -22.32447841415231338, 25.34915137120643180, 11.00000000000000000 ) ) ;
#32053=CARTESIAN_POINT ( 'NONE',  ( -8.118377661053488126, 10.47536095541708967, 7.000000000000000000 ) ) ;
#32057=DIRECTION ( 'NONE',  ( -1.000000000000000000, 0.000000000000000000, 0.000000000000000000 ) ) ;
#32064=VECTOR ( 'NONE', #18019, 1000.000000000000000 ) ;
#32071=FACE_OUTER_BOUND ( 'NONE', #31920, .T. ) ;
#32075=AXIS2_PLACEMENT_3D ( 'NONE', #39352, #33476, #23912 ) ;
#32077=EDGE_LOOP ( 'NONE', ( #39102, #15115, #9651, #24990, #408 ) ) ;
#32079=FACE_OUTER_BOUND ( 'NONE', #6658, .T. ) ;
#32081=EDGE_CURVE ( 'NONE', #25787, #8554, #9392, .T. ) ;
#32082=B_SPLINE_SURFACE_WITH_KNOTS ( 'NONE', 1, 3, ( 
 ( #22343, #21952, #37601, #25391, #9371, #6899, #31104, #3468, #12409, #25002 ),
 ( #15260, #12212, #15661, #9767, #24801, #2872, #15460, #6502, #34548, #37394 ) ),
 .UNSPECIFIED., .F., .F., .F.,
 ( 2, 2 ),
 ( 4, 2, 2, 2, 4 ),
 ( 0.000000000000000000, 1.000000000000000000 ),
 ( -1.421612811542168231, -1.028913729843446090, -0.6362146481447240598, -0.2435155664460019742, 0.1491835152527200836 ),
 .UNSPECIFIED. ) ;
#32083=EDGE_LOOP ( 'NONE', ( #32390, #7950, #27409 ) ) ;
#32086=ORIENTED_EDGE ( 'NONE', *, *, #9158, .F. ) ;
#32089=VERTEX_POINT ( 'NONE', #24201 ) ;
#32091=FACE_OUTER_BOUND ( 'NONE', #4857, .T. ) ;
#32094=CARTESIAN_POINT ( 'NONE',  ( 4.524139159579307012, 31.43208625488810171, 10.00000000000000000 ) ) ;
#32096=AXIS2_PLACEMENT_3D ( 'NONE', #24, #11815, #5510 ) ;
#32100=DIRECTION ( 'NONE',  ( -0.000000000000000000, -0.000000000000000000, 1.000000000000000000 ) ) ;
#32101=EDGE_CURVE ( 'NONE', #23066, #37754, #6730, .T. ) ;
#32102=LINE ( 'NONE', #38395, #24697 ) ;
#32105=ORIENTED_EDGE ( 'NONE', *, *, #35133, .T. ) ;
#32107=LINE ( 'NONE', #4067, #7786 ) ;
#32110=LINE ( 'NONE', #19721, #32190 ) ;
#32111=B_SPLINE_CURVE_WITH_KNOTS ( 'NONE', 3,
 ( #17876, #21111, #39788, #8109, #5659, #20911 ),
 .UNSPECIFIED., .F., .F.,
 ( 4, 2, 4 ),
 ( 0.000000000000000000, 0.4333333202469910606, 0.8666666404939821211 ),
 .UNSPECIFIED. ) ;
#32117=EDGE_CURVE ( 'NONE', #3600, #9898, #40033, .T. ) ;
#32122=AXIS2_PLACEMENT_3D ( 'NONE', #4169, #11284, #1330 ) ;
#32123=DIRECTION ( 'NONE',  ( -0.000000000000000000, -0.000000000000000000, -1.000000000000000000 ) ) ;
#32124=CARTESIAN_POINT ( 'NONE',  ( -12.38757880222266650, 14.77067777473956767, 10.99387789255785464 ) ) ;
#32125=AXIS2_PLACEMENT_3D ( 'NONE', #15613, #3616, #6458 ) ;
#32129=ORIENTED_EDGE ( 'NONE', *, *, #31739, .T. ) ;
#32131=EDGE_CURVE ( 'NONE', #7162, #11320, #2788, .T. ) ;
#32134=ADVANCED_FACE ( 'NONE', ( #11622 ), #14589, .T. ) ;
#32135=ORIENTED_EDGE ( 'NONE', *, *, #30958, .T. ) ;
#32138=ORIENTED_EDGE ( 'NONE', *, *, #21753, .T. ) ;
#32140=LINE ( 'NONE', #22987, #16145 ) ;
#32146=CIRCLE ( 'NONE', #28892, 0.5000000000000001110 ) ;
#32148=FACE_OUTER_BOUND ( 'NONE', #26992, .T. ) ;
#32150=PLANE ( 'NONE',  #13044 ) ;
#32153=AXIS2_PLACEMENT_3D ( 'NONE', #21455, #15164, #18418 ) ;
#32154=TOROIDAL_SURFACE ( 'NONE', #33461, 1.000000000000000000, 0.5000000000000000000 ) ;
#32160=ORIENTED_EDGE ( 'NONE', *, *, #32743, .F. ) ;
#32162=ORIENTED_EDGE ( 'NONE', *, *, #28988, .T. ) ;
#32170=ORIENTED_EDGE ( 'NONE', *, *, #9617, .F. ) ;
#32172=PLANE ( 'NONE',  #10174 ) ;
#32174=ADVANCED_FACE ( 'NONE', ( #2480 ), #18315, .T. ) ;
#32179=CARTESIAN_POINT ( 'NONE',  ( 12.05736835487432579, 14.38397459621550567, 10.49999999999999822 ) ) ;
#32181=ORIENTED_EDGE ( 'NONE', *, *, #38260, .T. ) ;
#32183=CARTESIAN_POINT ( 'NONE',  ( -11.74460609746112461, 31.83082137946488643, 7.365559175140416137 ) ) ;
#32189=CONICAL_SURFACE ( 'NONE', #31513, 1.000000000000004441, 0.7853981633974591592 ) ;
#32190=VECTOR ( 'NONE', #4275, 1000.000000000000000 ) ;
#32192=VECTOR ( 'NONE', #2784, 1000.000000000000114 ) ;
#32193=ORIENTED_EDGE ( 'NONE', *, *, #18111, .F. ) ;
#32195=CARTESIAN_POINT ( 'NONE',  ( -14.09933648065464062, 26.02968990214173317, 10.50000000000000533 ) ) ;
#32196=DIRECTION ( 'NONE',  ( 0.4999999999999919509, -0.8660254037844432595, 0.000000000000000000 ) ) ;
#32197=DIRECTION ( 'NONE',  ( -0.5877852522924690293, 0.8090169943749503378, -0.000000000000000000 ) ) ;
#32199=CARTESIAN_POINT ( 'NONE',  ( -11.11016527260153630, 31.83082137946488643, 11.00000000000000000 ) ) ;
#32202=EDGE_LOOP ( 'NONE', ( #18574, #35166, #15552, #18771 ) ) ;
#32204=DIRECTION ( 'NONE',  ( -0.6691306063588671194, -0.7431448254773862505, 0.000000000000000000 ) ) ;
#32206=DIRECTION ( 'NONE',  ( 0.7032331762534084207, 0.07391278520354237214, -0.7071067811865459074 ) ) ;
#32207=DIRECTION ( 'NONE',  ( 0.000000000000000000, -0.000000000000000000, -1.000000000000000000 ) ) ;
#32209=ORIENTED_EDGE ( 'NONE', *, *, #26253, .T. ) ;
#32211=VECTOR ( 'NONE', #8641, 1000.000000000000000 ) ;
#32212=CARTESIAN_POINT ( 'NONE',  ( 14.42035624161478857, 26.65972665747660031, 10.50000000000000000 ) ) ;
#32213=VECTOR ( 'NONE', #16741, 1000.000000000000000 ) ;
#32217=VERTEX_POINT ( 'NONE', #19301 ) ;
#32219=ORIENTED_EDGE ( 'NONE', *, *, #35193, .F. ) ;
#32221=DIRECTION ( 'NONE',  ( 0.000000000000000000, 0.000000000000000000, 1.000000000000000000 ) ) ;
#32223=EDGE_CURVE ( 'NONE', #8314, #22563, #12635, .T. ) ;
#32229=EDGE_CURVE ( 'NONE', #39481, #24143, #37994, .T. ) ;
#32232=CARTESIAN_POINT ( 'NONE',  ( -9.697889840765283154, 31.90483559858340357, 10.00000000000000000 ) ) ;
#32234=VERTEX_POINT ( 'NONE', #22543 ) ;
#32238=CARTESIAN_POINT ( 'NONE',  ( -19.50480011250488843, 16.42246729932494276, 10.00000000000000000 ) ) ;
#32239=VERTEX_POINT ( 'NONE', #10566 ) ;
#32240=CARTESIAN_POINT ( 'NONE',  ( -13.13581098909220302, 27.45627467658446008, 7.499999999999993783 ) ) ;
#32241=CARTESIAN_POINT ( 'NONE',  ( -10.03245514394471627, 31.53326318584470656, 7.000000000000000000 ) ) ;
#32242=CARTESIAN_POINT ( 'NONE',  ( -12.99377146717200660, 26.19620116591435277, 7.000000000000000000 ) ) ;
#32246=CIRCLE ( 'NONE', #14730, 1.000000000000004441 ) ;
#32247=ORIENTED_EDGE ( 'NONE', *, *, #21207, .F. ) ;
#32248=LINE ( 'NONE', #4412, #11950 ) ;
#32252=LINE ( 'NONE', #25940, #22689 ) ;
#32255=PLANE ( 'NONE',  #21086 ) ;
#32256=DIRECTION ( 'NONE',  ( -0.5254827454987532898, 0.4731467892558212651, -0.7071067811865475727 ) ) ;
#32257=CARTESIAN_POINT ( 'NONE',  ( -8.505700342264141511, 22.10876900990917804, 9.000000000000001776 ) ) ;
#32258=DIRECTION ( 'NONE',  ( -0.1045284632676570929, -0.9945218953682729568, 0.000000000000000000 ) ) ;
#32262=EDGE_LOOP ( 'NONE', ( #15881, #18305, #3924 ) ) ;
#32264=DIRECTION ( 'NONE',  ( 0.5877852522924690293, -0.8090169943749503378, 0.000000000000000000 ) ) ;
#32265=CARTESIAN_POINT ( 'NONE',  ( -14.11133924723977451, 27.61078317377193869, 10.49999999999999112 ) ) ;
#32267=FACE_OUTER_BOUND ( 'NONE', #27990, .T. ) ;
#32273=VECTOR ( 'NONE', #4600, 1000.000000000000114 ) ;
#32277=EDGE_CURVE ( 'NONE', #18096, #13411, #23361, .T. ) ;
#32279=DIRECTION ( 'NONE',  ( 1.000000000000000000, 0.000000000000000000, 0.000000000000000000 ) ) ;
#32284=EDGE_LOOP ( 'NONE', ( #1909, #28308, #11210 ) ) ;
#32287=DIRECTION ( 'NONE',  ( -0.9781476007338069101, -0.2079116908177533751, 0.000000000000000000 ) ) ;
#32290=PLANE ( 'NONE',  #5077 ) ;
#32291=DIRECTION ( 'NONE',  ( 0.000000000000000000, 0.000000000000000000, -1.000000000000000000 ) ) ;
#32296=VERTEX_POINT ( 'NONE', #26399 ) ;
#32300=DIRECTION ( 'NONE',  ( 0.2876062384759424106, -0.6459741880212539478, -0.7071067811865482389 ) ) ;
#32302=VECTOR ( 'NONE', #8952, 1000.000000000000000 ) ;
#32304=CARTESIAN_POINT ( 'NONE',  ( 13.94482798346721353, 26.50521816028912525, 9.000000000000001776 ) ) ;
#32305=ORIENTED_EDGE ( 'NONE', *, *, #36311, .T. ) ;
#32307=CARTESIAN_POINT ( 'NONE',  ( 9.331903152615748098, 11.35703883385568780, 7.500000000000000888 ) ) ;
#32310=CONICAL_SURFACE ( 'NONE', #37493, 1.000000000000014655, 0.7853981633974526089 ) ;
#32311=CARTESIAN_POINT ( 'NONE',  ( 10.44103466624280507, 32.57396620494213124, 7.000000000000000000 ) ) ;
#32313=CIRCLE ( 'NONE', #20631, 6.000000000000000888 ) ;
#32315=ORIENTED_EDGE ( 'NONE', *, *, #15111, .T. ) ;
#32316=CARTESIAN_POINT ( 'NONE',  ( 4.984135866956517447, 36.15314577889351000, 7.500000000000000888 ) ) ;
#32319=LINE ( 'NONE', #6708, #10047 ) ;
#32325=CARTESIAN_POINT ( 'NONE',  ( 8.118377661053324701, 10.47536095541698486, 11.00000000000000000 ) ) ;
#32326=VERTEX_POINT ( 'NONE', #35552 ) ;
#32327=ORIENTED_EDGE ( 'NONE', *, *, #7543, .T. ) ;
#32331=CIRCLE ( 'NONE', #14812, 0.9999999999999974465 ) ;
#32335=EDGE_LOOP ( 'NONE', ( #25202, #18513, #1399, #23261 ) ) ;
#32337=CARTESIAN_POINT ( 'NONE',  ( -5.400683141673551901, 15.91724817395922997, 7.000000000000000000 ) ) ;
#32339=EDGE_CURVE ( 'NONE', #31037, #32234, #30157, .T. ) ;
#32341=CONICAL_SURFACE ( 'NONE', #23256, 1.000000000000004441, 0.7853981633974522758 ) ;
#32342=EDGE_LOOP ( 'NONE', ( #17507, #25066, #6968 ) ) ;
#32344=CARTESIAN_POINT ( 'NONE',  ( -5.558911028763774631, 36.44455752850708308, 10.49999999999999822 ) ) ;
#32345=VERTEX_POINT ( 'NONE', #4866 ) ;
#32347=AXIS2_PLACEMENT_3D ( 'NONE', #36339, #8094, #11152 ) ;
#32348=LINE ( 'NONE', #35391, #23915 ) ;
#32350=ORIENTED_EDGE ( 'NONE', *, *, #5168, .T. ) ;
#32353=CYLINDRICAL_SURFACE ( 'NONE', #6550, 0.5000000000000004441 ) ;
#32356=ADVANCED_FACE ( 'NONE', ( #5071 ), #20117, .T. ) ;
#32357=CARTESIAN_POINT ( 'NONE',  ( 8.339609403135806787, 11.87216320208440479, 9.500000000000000000 ) ) ;
#32358=CIRCLE ( 'NONE', #38182, 0.5000000000000007772 ) ;
#32370=ORIENTED_EDGE ( 'NONE', *, *, #23048, .F. ) ;
#32375=CARTESIAN_POINT ( 'NONE',  ( -14.26729173199937684, 26.60999298350843389, 10.87262190629277647 ) ) ;
#32377=ORIENTED_EDGE ( 'NONE', *, *, #39823, .F. ) ;
#32381=DIRECTION ( 'NONE',  ( 0.000000000000000000, 0.000000000000000000, -1.000000000000000000 ) ) ;
#32382=B_SPLINE_CURVE_WITH_KNOTS ( 'NONE', 3,
 ( #27877, #8998, #15089, #25028, #21580, #12435 ),
 .UNSPECIFIED., .F., .F.,
 ( 4, 2, 4 ),
 ( 0.000000000000000000, 0.5000000000000000000, 1.000000000000000000 ),
 .UNSPECIFIED. ) ;
#32384=DIRECTION ( 'NONE',  ( 1.000000000000000000, 0.000000000000000000, 0.000000000000000000 ) ) ;
#32385=VERTEX_POINT ( 'NONE', #29651 ) ;
#32388=CARTESIAN_POINT ( 'NONE',  ( -5.440908595777639079, 35.94977745735568675, 11.00000000000000000 ) ) ;
#32390=ORIENTED_EDGE ( 'NONE', *, *, #38942, .T. ) ;
#32393=ADVANCED_FACE ( 'NONE', ( #33117 ), #1834, .T. ) ;
#32395=EDGE_CURVE ( 'NONE', #6243, #29659, #11170, .T. ) ;
#32400=CIRCLE ( 'NONE', #18758, 0.4999999999999998335 ) ;
#32406=CARTESIAN_POINT ( 'NONE',  ( -6.607858460703655901, 34.88289976392069747, 9.500000000000000000 ) ) ;
#32407=CARTESIAN_POINT ( 'NONE',  ( 14.02783499842348647, 22.03112340962107751, 9.500000000000000000 ) ) ;
#32409=DIRECTION ( 'NONE',  ( 1.000000000000000000, 0.000000000000000000, 0.000000000000000000 ) ) ;
#32410=CYLINDRICAL_SURFACE ( 'NONE', #13213, 0.4999999999999997224 ) ;
#32411=CARTESIAN_POINT ( 'NONE',  ( -0.5000000000000008882, 36.00000000000000711, 10.50000000000000000 ) ) ;
#32412=EDGE_LOOP ( 'NONE', ( #30206, #39032, #25534, #40133 ) ) ;
#32414=DIRECTION ( 'NONE',  ( 0.6691306063588662312, 0.7431448254773869166, 0.000000000000000000 ) ) ;
#32416=CARTESIAN_POINT ( 'NONE',  ( 3.153820973115410098, 32.04219121950180238, 10.49999999999999822 ) ) ;
#32417=CARTESIAN_POINT ( 'NONE',  ( 1.000000000000000666, 32.50000000000000000, 10.50000000000000178 ) ) ;
#32419=DIRECTION ( 'NONE',  ( 0.000000000000000000, -0.000000000000000000, 1.000000000000000000 ) ) ;
#32420=AXIS2_PLACEMENT_3D ( 'NONE', #23264, #14722, #30163 ) ;
#32421=ORIENTED_EDGE ( 'NONE', *, *, #37180, .F. ) ;
#32423=CYLINDRICAL_SURFACE ( 'NONE', #35466, 0.4999999999999986122 ) ;
#32425=CARTESIAN_POINT ( 'NONE',  ( 14.31603901957230462, 19.98981538725069740, 10.50000000000000533 ) ) ;
#32427=VERTEX_POINT ( 'NONE', #13607 ) ;
#32429=VECTOR ( 'NONE', #33718, 1000.000000000000000 ) ;
#32430=ORIENTED_EDGE ( 'NONE', *, *, #28271, .F. ) ;
#32441=CARTESIAN_POINT ( 'NONE',  ( 0.5000000000000000000, 37.00000000000000711, 10.99999999999999645 ) ) ;
#32442=EDGE_CURVE ( 'NONE', #614, #16736, #23562, .T. ) ;
#32443=DIRECTION ( 'NONE',  ( -0.000000000000000000, -0.000000000000000000, -1.000000000000000000 ) ) ;
#32444=ORIENTED_EDGE ( 'NONE', *, *, #39892, .F. ) ;
#32449=CARTESIAN_POINT ( 'NONE',  ( 6.151085731882510288, 35.08626808545850650, 10.00000000000000000 ) ) ;
#32450=CARTESIAN_POINT ( 'NONE',  ( -13.97557076678966403, 21.53386246193713305, 7.500000000000004441 ) ) ;
#32453=CIRCLE ( 'NONE', #656, 6.000000000000005329 ) ;
#32457=DIRECTION ( 'NONE',  ( 1.000000000000000000, 0.000000000000000000, 0.000000000000000000 ) ) ;
#32458=B_SPLINE_CURVE_WITH_KNOTS ( 'NONE', 3,
 ( #5732, #14884, #21570, #5530, #27467, #9185 ),
 .UNSPECIFIED., .F., .F.,
 ( 4, 2, 4 ),
 ( 0.000000000000000000, 0.5000000000000000000, 1.000000000000000000 ),
 .UNSPECIFIED. ) ;
#32459=EDGE_CURVE ( 'NONE', #2015, #24787, #19911, .T. ) ;
#32461=EDGE_LOOP ( 'NONE', ( #35174, #30549, #38391, #6371 ) ) ;
#32464=FACE_OUTER_BOUND ( 'NONE', #7892, .T. ) ;
#32465=DIRECTION ( 'NONE',  ( -0.000000000000000000, -0.000000000000000000, -1.000000000000000000 ) ) ;
#32466=EDGE_CURVE ( 'NONE', #35419, #2211, #27206, .T. ) ;
#32471=PLANE ( 'NONE',  #25046 ) ;
#32472=VERTEX_POINT ( 'NONE', #8922 ) ;
#32474=EDGE_CURVE ( 'NONE', #27705, #27849, #15216, .T. ) ;
#32476=LINE ( 'NONE', #13366, #20684 ) ;
#32479=CARTESIAN_POINT ( 'NONE',  ( 11.81630298851978722, 31.79381426990546089, 11.00000000000000000 ) ) ;
#32487=CARTESIAN_POINT ( 'NONE',  ( 5.440908595777817602, 35.94977745735560859, 7.000000000000000000 ) ) ;
#32488=EDGE_CURVE ( 'NONE', #6492, #39980, #2283, .T. ) ;
#32490=VECTOR ( 'NONE', #26201, 1000.000000000000000 ) ;
#32492=ADVANCED_FACE ( 'NONE', ( #27402 ), #33721, .T. ) ;
#32495=DIRECTION ( 'NONE',  ( 0.9945218953682740670, 0.1045284632676460046, 0.000000000000000000 ) ) ;
#32496=ORIENTED_EDGE ( 'NONE', *, *, #4512, .F. ) ;
#32497=DIRECTION ( 'NONE',  ( 0.000000000000000000, 0.000000000000000000, 1.000000000000000000 ) ) ;
#32498=CARTESIAN_POINT ( 'NONE',  ( 9.997483185316561105, 21.95197631500756685, 10.50000000000000000 ) ) ;
#32501=EDGE_LOOP ( 'NONE', ( #32893, #9552, #10790, #18157 ) ) ;
#32503=VECTOR ( 'NONE', #18169, 1000.000000000000114 ) ;
#32504=CIRCLE ( 'NONE', #29879, 1.000000000000013101 ) ;
#32509=DIRECTION ( 'NONE',  ( 1.000000000000000000, 0.000000000000000000, 0.000000000000000000 ) ) ;
#32510=DIRECTION ( 'NONE',  ( -0.8660254037844431485, -0.4999999999999921174, 0.000000000000000000 ) ) ;
#32513=CARTESIAN_POINT ( 'NONE',  ( -11.60262927932668298, 31.67393310092496961, 10.49999999999999822 ) ) ;
#32514=VERTEX_POINT ( 'NONE', #36955 ) ;
#32515=EDGE_CURVE ( 'NONE', #27237, #25471, #12363, .T. ) ;
#32516=( NAMED_UNIT ( * ) SI_UNIT ( $, .STERADIAN. ) SOLID_ANGLE_UNIT ( ) );
#32517=DIRECTION ( 'NONE',  ( 0.3090169943749573878, 0.9510565162951503115, 0.000000000000000000 ) ) ;
#32518=CARTESIAN_POINT ( 'NONE',  ( -14.47283171447380035, 21.48159823030330884, 9.000000000000001776 ) ) ;
#32519=AXIS2_PLACEMENT_3D ( 'NONE', #37996, #4061, #35149 ) ;
#32520=CARTESIAN_POINT ( 'NONE',  ( -14.84160187385924523, 20.32586711126994672, 7.000000000000000000 ) ) ;
#32523=VERTEX_POINT ( 'NONE', #36755 ) ;
#32528=DIRECTION ( 'NONE',  ( 0.1045284632676569680, 0.9945218953682730678, -0.000000000000000000 ) ) ;
#32529=ORIENTED_EDGE ( 'NONE', *, *, #25537, .T. ) ;
#32531=AXIS2_PLACEMENT_3D ( 'NONE', #26854, #20963, #14866 ) ;
#32539=PLANE ( 'NONE',  #4243 ) ;
#32542=CARTESIAN_POINT ( 'NONE',  ( 8.160254037844358876, 16.63397459621553054, 10.49999999999999822 ) ) ;
#32543=ORIENTED_EDGE ( 'NONE', *, *, #30990, .T. ) ;
#32545=CARTESIAN_POINT ( 'NONE',  ( -10.50986403156571036, 32.63594044384558401, 10.99387789255783510 ) ) ;
#32546=DIRECTION ( 'NONE',  ( -1.000000000000000000, 0.000000000000000000, 0.000000000000000000 ) ) ;
#32547=LINE ( 'NONE', #9992, #1157 ) ;
#32548=ORIENTED_EDGE ( 'NONE', *, *, #26435, .T. ) ;
#32550=FACE_OUTER_BOUND ( 'NONE', #6317, .T. ) ;
#32557=LINE ( 'NONE', #38639, #15644 ) ;
#32559=DIRECTION ( 'NONE',  ( 0.5778781230733963659, 0.000000000000000000, 0.8161230758122015594 ) ) ;
#32560=ORIENTED_EDGE ( 'NONE', *, *, #442, .F. ) ;
#32561=AXIS2_PLACEMENT_3D ( 'NONE', #33114, #8716, #27203 ) ;
#32562=CARTESIAN_POINT ( 'NONE',  ( 13.24038105676655164, 15.43301270189216368, 10.49999999999999822 ) ) ;
#32566=CONICAL_SURFACE ( 'NONE', #9852, 0.5000000000000023315, 0.7853981633974492782 ) ;
#32569=FACE_OUTER_BOUND ( 'NONE', #33065, .T. ) ;
#32570=DIRECTION ( 'NONE',  ( 1.000000000000000000, 0.000000000000000000, 0.000000000000000000 ) ) ;
#32571=ORIENTED_EDGE ( 'NONE', *, *, #19718, .T. ) ;
#32573=ORIENTED_EDGE ( 'NONE', *, *, #9889, .T. ) ;
#32576=CARTESIAN_POINT ( 'NONE',  ( -14.42035624161472995, 26.65972665747678505, 10.49999999999999112 ) ) ;
#32578=ORIENTED_EDGE ( 'NONE', *, *, #26869, .F. ) ;
#32580=ORIENTED_EDGE ( 'NONE', *, *, #25892, .T. ) ;
#32582=DIRECTION ( 'NONE',  ( 0.000000000000000000, 0.000000000000000000, 1.000000000000000000 ) ) ;
#32584=B_SPLINE_CURVE_WITH_KNOTS ( 'NONE', 3,
 ( #22064, #28758, #21862, #933 ),
 .UNSPECIFIED., .F., .F.,
 ( 4, 4 ),
 ( 0.000000000000000000, 0.0001748523089235895619 ),
 .UNSPECIFIED. ) ;
#32585=DIRECTION ( 'NONE',  ( 0.8090169943749423442, -0.5877852522924800205, 0.000000000000000000 ) ) ;
#32591=ORIENTED_EDGE ( 'NONE', *, *, #821, .F. ) ;
#32593=ADVANCED_FACE ( 'NONE', ( #21504 ), #39791, .T. ) ;
#32594=FACE_OUTER_BOUND ( 'NONE', #23444, .T. ) ;
#32596=ORIENTED_EDGE ( 'NONE', *, *, #11946, .T. ) ;
#32599=EDGE_CURVE ( 'NONE', #38623, #19050, #10560, .T. ) ;
#32601=EDGE_LOOP ( 'NONE', ( #1456, #31762, #30818, #20060 ) ) ;
#32604=EDGE_CURVE ( 'NONE', #35381, #21382, #36355, .T. ) ;
#32607=AXIS2_PLACEMENT_3D ( 'NONE', #34230, #37272, #18594 ) ;
#32608=DIRECTION ( 'NONE',  ( 1.000000000000000000, 0.000000000000000000, 0.000000000000000000 ) ) ;
#32609=CARTESIAN_POINT ( 'NONE',  ( 0.5000000000000000000, 37.00000000000000711, 11.00000000000000000 ) ) ;
#32610=CARTESIAN_POINT ( 'NONE',  ( 6.460609604078280555, 35.78147008481143132, 10.94611345180490680 ) ) ;
#32612=LINE ( 'NONE', #28943, #33481 ) ;
#32615=EDGE_CURVE ( 'NONE', #21181, #12596, #8518, .T. ) ;
#32616=CARTESIAN_POINT ( 'NONE',  ( -6.557822374958091949, 35.99981354310121873, 10.59344459855558540 ) ) ;
#32617=ADVANCED_FACE ( 'NONE', ( #9323 ), #26263, .T. ) ;
#32618=DIRECTION ( 'NONE',  ( 0.9781476007338069101, 0.2079116908177532641, 0.000000000000000000 ) ) ;
#32620=DIRECTION ( 'NONE',  ( 0.9781476007338072431, 0.2079116908177519041, 0.000000000000000000 ) ) ;
#32621=DIRECTION ( 'NONE',  ( 0.9659258262890655367, -0.2588190451025308980, -9.462988938997540172E-16 ) ) ;
#32623=VECTOR ( 'NONE', #11871, 1000.000000000000114 ) ;
#32624=CARTESIAN_POINT ( 'NONE',  ( -3.665809487923753274, 43.57847826359346755, 10.00000000000000000 ) ) ;
#32625=VERTEX_POINT ( 'NONE', #5268 ) ;
#32628=VECTOR ( 'NONE', #13, 1000.000000000000114 ) ;
#32630=CARTESIAN_POINT ( 'NONE',  ( 22.42900687741999732, 24.35462947583785720, 11.00000000000000000 ) ) ;
#32632=VERTEX_POINT ( 'NONE', #18073 ) ;
#32634=ORIENTED_EDGE ( 'NONE', *, *, #4660, .T. ) ;
#32639=VECTOR ( 'NONE', #37816, 1000.000000000000000 ) ;
#32643=ORIENTED_EDGE ( 'NONE', *, *, #28531, .T. ) ;
#32645=CARTESIAN_POINT ( 'NONE',  ( -3.118675362266497775, 7.827785988992935096, 7.000000000000000000 ) ) ;
#32647=CARTESIAN_POINT ( 'NONE',  ( 2.525645716490524606, 8.212903943950921715, 11.00000000000000000 ) ) ;
#32648=ORIENTED_EDGE ( 'NONE', *, *, #21909, .F. ) ;
#32654=CIRCLE ( 'NONE', #13138, 1.000000000000013101 ) ;
#32655=CARTESIAN_POINT ( 'NONE',  ( -9.665073660138984835, 25.11464168560199184, 10.50000000000000000 ) ) ;
#32659=CARTESIAN_POINT ( 'NONE',  ( -10.29511041547401895, 24.79362192464190073, 10.50000000000000533 ) ) ;
#32661=VECTOR ( 'NONE', #6497, 1000.000000000000000 ) ;
#32662=CARTESIAN_POINT ( 'NONE',  ( 5.490944681523308724, 34.83286367817510154, 7.000000000000000000 ) ) ;
#32665=LINE ( 'NONE', #4214, #347 ) ;
#32668=ADVANCED_FACE ( 'NONE', ( #38139 ), #10115, .F. ) ;
#32669=FACE_OUTER_BOUND ( 'NONE', #29869, .T. ) ;
#32670=CARTESIAN_POINT ( 'NONE',  ( 12.30736835487432934, 14.81698729810772797, 11.00000000000000000 ) ) ;
#32671=AXIS2_PLACEMENT_3D ( 'NONE', #5025, #26757, #8476 ) ;
#32674=CARTESIAN_POINT ( 'NONE',  ( 0.000000000000000000, 22.50000000000000355, 7.000000000000000000 ) ) ;
#32675=ORIENTED_EDGE ( 'NONE', *, *, #22058, .F. ) ;
#32677=CARTESIAN_POINT ( 'NONE',  ( 1.000000000000000222, 36.00000000000000711, 10.50000000000000000 ) ) ;
#32680=DIRECTION ( 'NONE',  ( -0.5773502691896259531, -0.5773502691896217343, 0.5773502691896298389 ) ) ;
#32683=DIRECTION ( 'NONE',  ( 1.000000000000000000, 0.000000000000000000, 0.000000000000000000 ) ) ;
#32689=CARTESIAN_POINT ( 'NONE',  ( 0.5000000000000004441, 36.00000000000000711, 9.500000000000000000 ) ) ;
#32690=EDGE_LOOP ( 'NONE', ( #32430, #1337, #5309, #570 ) ) ;
#32693=EDGE_CURVE ( 'NONE', #22086, #29202, #34503, .T. ) ;
#32694=VECTOR ( 'NONE', #10359, 1000.000000000000000 ) ;
#32695=DIRECTION ( 'NONE',  ( -0.000000000000000000, -0.000000000000000000, 1.000000000000000000 ) ) ;
#32698=CARTESIAN_POINT ( 'NONE',  ( 8.927394655428274817, 11.06314620770945290, 11.00000000000000000 ) ) ;
#32703=AXIS2_PLACEMENT_3D ( 'NONE', #29551, #36054, #33219 ) ;
#32706=CARTESIAN_POINT ( 'NONE',  ( 14.11133924723984379, 27.61078317377175750, 10.49999999999999822 ) ) ;
#32707=ORIENTED_EDGE ( 'NONE', *, *, #26160, .T. ) ;
#32712=DIRECTION ( 'NONE',  ( 0.7431448254773961315, 0.6691306063588561281, 0.000000000000000000 ) ) ;
#32713=VERTEX_POINT ( 'NONE', #28000 ) ;
#32714=DIRECTION ( 'NONE',  ( 1.000000000000000000, 0.000000000000000000, 0.000000000000000000 ) ) ;
#32715=CARTESIAN_POINT ( 'NONE',  ( -2.672146553953451242, 12.33340603770395560, 11.00000000000000000 ) ) ;
#32716=DIRECTION ( 'NONE',  ( 0.000000000000000000, 0.000000000000000000, 1.000000000000000000 ) ) ;
#32721=ORIENTED_EDGE ( 'NONE', *, *, #24665, .T. ) ;
#32722=DIRECTION ( 'NONE',  ( 1.000000000000000000, 0.000000000000000000, 0.000000000000000000 ) ) ;
#32725=DIRECTION ( 'NONE',  ( 0.9510565162951503115, -0.3090169943749572767, 0.000000000000000000 ) ) ;
#32726=CARTESIAN_POINT ( 'NONE',  ( 5.473344025737210572, 14.11593743010426394, 10.49999999999999822 ) ) ;
#32727=ORIENTED_EDGE ( 'NONE', *, *, #33389, .F. ) ;
#32732=ORIENTED_EDGE ( 'NONE', *, *, #36802, .F. ) ;
#32736=EDGE_CURVE ( 'NONE', #25142, #3653, #19249, .T. ) ;
#32738=AXIS2_PLACEMENT_3D ( 'NONE', #12374, #37359, #3032 ) ;
#32741=ORIENTED_EDGE ( 'NONE', *, *, #3395, .F. ) ;
#32743=EDGE_CURVE ( 'NONE', #5091, #38482, #5238, .T. ) ;
#32744=CARTESIAN_POINT ( 'NONE',  ( -10.81260707898156959, 32.90853150812147021, 10.59344459855568843 ) ) ;
#32745=DIRECTION ( 'NONE',  ( 0.2079116908177532919, -0.9781476007338070211, -0.000000000000000000 ) ) ;
#32749=CARTESIAN_POINT ( 'NONE',  ( -13.97943872024075951, 27.84235072122942611, 10.49999999999999822 ) ) ;
#32750=ORIENTED_EDGE ( 'NONE', *, *, #35246, .T. ) ;
#32752=VECTOR ( 'NONE', #32197, 1000.000000000000114 ) ;
#32753=EDGE_CURVE ( 'NONE', #20104, #39848, #19450, .T. ) ;
#32760=LINE ( 'NONE', #10411, #13558 ) ;
#32761=ORIENTED_EDGE ( 'NONE', *, *, #23736, .F. ) ;
#32762=CARTESIAN_POINT ( 'NONE',  ( -7.748210172783978500, 9.655561136695068214, 7.102637441331450141 ) ) ;
#32765=AXIS2_PLACEMENT_3D ( 'NONE', #11583, #26817, #29263 ) ;
#32770=FACE_OUTER_BOUND ( 'NONE', #32989, .T. ) ;
#32771=VECTOR ( 'NONE', #28952, 1000.000000000000227 ) ;
#32776=EDGE_LOOP ( 'NONE', ( #32193, #17727, #11790, #11353 ) ) ;
#32782=ORIENTED_EDGE ( 'NONE', *, *, #10805, .T. ) ;
#32784=ORIENTED_EDGE ( 'NONE', *, *, #22388, .T. ) ;
#32793=LINE ( 'NONE', #23437, #29372 ) ;
#32797=EDGE_CURVE ( 'NONE', #15571, #31096, #14441, .T. ) ;
#32798=CARTESIAN_POINT ( 'NONE',  ( -8.395951170269910335, 10.09331379572990350, 10.68306085400108607 ) ) ;
#32800=ORIENTED_EDGE ( 'NONE', *, *, #14456, .F. ) ;
#32805=ORIENTED_EDGE ( 'NONE', *, *, #26160, .F. ) ;
#32810=AXIS2_PLACEMENT_3D ( 'NONE', #13503, #23658, #36055 ) ;
#32813=DIRECTION ( 'NONE',  ( -0.000000000000000000, -0.000000000000000000, -1.000000000000000000 ) ) ;
#32815=DIRECTION ( 'NONE',  ( -0.7071067811865500152, 1.239037099348077946E-16, -0.7071067811865451302 ) ) ;
#32816=ORIENTED_EDGE ( 'NONE', *, *, #21510, .F. ) ;
#32819=CARTESIAN_POINT ( 'NONE',  ( 4.096822963000107620, 8.035697679810645866, 11.00000000000000000 ) ) ;
#32821=EDGE_CURVE ( 'NONE', #3600, #28389, #24331, .T. ) ;
#32823=CARTESIAN_POINT ( 'NONE',  ( -14.46041492111391946, 20.47739500831029957, 10.99387789255785108 ) ) ;
#32826=ORIENTED_EDGE ( 'NONE', *, *, #215, .F. ) ;
#32837=DIRECTION ( 'NONE',  ( -1.000000000000000000, 0.000000000000000000, 0.000000000000000000 ) ) ;
#32841=CONICAL_SURFACE ( 'NONE', #36079, 0.9999999999999986677, 0.7853981633974503884 ) ;
#32845=EDGE_LOOP ( 'NONE', ( #5608, #25526, #38845, #22531 ) ) ;
#32847=VECTOR ( 'NONE', #12719, 1000.000000000000000 ) ;
#32848=FACE_OUTER_BOUND ( 'NONE', #14037, .T. ) ;
#32849=DIRECTION ( 'NONE',  ( 0.7431448254773846962, -0.6691306063588690067, 0.000000000000000000 ) ) ;
#32850=DIRECTION ( 'NONE',  ( -0.9945218953682730678, 0.1045284632676569819, -0.000000000000000000 ) ) ;
#32851=ORIENTED_EDGE ( 'NONE', *, *, #87, .T. ) ;
#32853=CARTESIAN_POINT ( 'NONE',  ( -13.48130249190472796, 27.93180293473203690, 11.00000000000000000 ) ) ;
#32855=CARTESIAN_POINT ( 'NONE',  ( -4.984135866956331817, 36.15314577889358105, 10.50000000000000533 ) ) ;
#32856=ADVANCED_FACE ( 'NONE', ( #34304 ), #6850, .T. ) ;
#32859=ORIENTED_EDGE ( 'NONE', *, *, #8529, .T. ) ;
#32861=VECTOR ( 'NONE', #20440, 1000.000000000000000 ) ;
#32863=ORIENTED_EDGE ( 'NONE', *, *, #22386, .T. ) ;
#32867=EDGE_CURVE ( 'NONE', #21421, #27921, #4216, .T. ) ;
#32868=CARTESIAN_POINT ( 'NONE',  ( 14.85579657860257541, 20.34187940403349870, 10.49999999999999822 ) ) ;
#32869=CARTESIAN_POINT ( 'NONE',  ( -14.09933648065464240, 26.02968990214173317, 11.00000000000000000 ) ) ;
#32872=DIRECTION ( 'NONE',  ( -0.5720614028176888022, -0.4156269377774527984, -0.7071067811865442421 ) ) ;
#32874=LINE ( 'NONE', #38552, #4277 ) ;
#32875=ORIENTED_EDGE ( 'NONE', *, *, #6469, .T. ) ;
#32877=PLANE ( 'NONE',  #8375 ) ;
#32879=CARTESIAN_POINT ( 'NONE',  ( -0.9938779058054629800, 37.09261900150649893, 10.49999999999999822 ) ) ;
#32882=CARTESIAN_POINT ( 'NONE',  ( 2.036571916123615100, 8.108948098542045457, 7.499999999999990230 ) ) ;
#32885=CYLINDRICAL_SURFACE ( 'NONE', #39517, 0.5000000000000000000 ) ;
#32893=ORIENTED_EDGE ( 'NONE', *, *, #33108, .F. ) ;
#32895=CIRCLE ( 'NONE', #6934, 0.5000000000000004441 ) ;
#32896=CIRCLE ( 'NONE', #34190, 0.5000000000000007772 ) ;
#32897=FACE_OUTER_BOUND ( 'NONE', #20800, .T. ) ;
#32898=ORIENTED_EDGE ( 'NONE', *, *, #26789, .F. ) ;
#32900=ADVANCED_FACE ( 'NONE', ( #11122 ), #16821, .T. ) ;
#32901=FACE_OUTER_BOUND ( 'NONE', #11761, .T. ) ;
#32902=EDGE_CURVE ( 'NONE', #16528, #15223, #38748, .T. ) ;
#32903=EDGE_LOOP ( 'NONE', ( #18348, #37196, #10683, #20405, #27739 ) ) ;
#32908=CARTESIAN_POINT ( 'NONE',  ( -0.4999999999999998890, 37.50000000000000711, 10.49999999999999822 ) ) ;
#32911=LINE ( 'NONE', #33517, #22794 ) ;
#32912=DIRECTION ( 'NONE',  ( -0.6691306063588570163, 0.7431448254773953543, -0.000000000000000000 ) ) ;
#32915=CARTESIAN_POINT ( 'NONE',  ( -2.579909280894606916, 7.957613945008774614, 10.94611345180490325 ) ) ;
#32919=CIRCLE ( 'NONE', #3063, 0.5000000000000004441 ) ;
#32924=CARTESIAN_POINT ( 'NONE',  ( -2.036571916123810055, 8.108948098542073879, 11.00000000000000000 ) ) ;
#32927=AXIS2_PLACEMENT_3D ( 'NONE', #30646, #6048, #34089 ) ;
#32935=EDGE_LOOP ( 'NONE', ( #12421, #10339, #21496, #18448 ) ) ;
#32937=DIRECTION ( 'NONE',  ( 0.000000000000000000, 0.000000000000000000, -1.000000000000000000 ) ) ;
#32938=CARTESIAN_POINT ( 'NONE',  ( 6.576253646258387597, 14.29921418520925513, 11.00000000000000000 ) ) ;
#32940=DIRECTION ( 'NONE',  ( -0.000000000000000000, -0.000000000000000000, -1.000000000000000000 ) ) ;
#32943=CYLINDRICAL_SURFACE ( 'NONE', #5711, 0.5000000000000000000 ) ;
#32946=EDGE_CURVE ( 'NONE', #18096, #22349, #32665, .T. ) ;
#32947=ORIENTED_EDGE ( 'NONE', *, *, #16236, .T. ) ;
#32950=ORIENTED_EDGE ( 'NONE', *, *, #4020, .T. ) ;
#32953=CIRCLE ( 'NONE', #5038, 15.00000000000000000 ) ;
#32954=CIRCLE ( 'NONE', #6328, 0.5000000000000004441 ) ;
#32956=ORIENTED_EDGE ( 'NONE', *, *, #26611, .T. ) ;
#32958=AXIS2_PLACEMENT_3D ( 'NONE', #22043, #2966, #33855 ) ;
#32960=CARTESIAN_POINT ( 'NONE',  ( -3.000488737322915878, 30.46850471150003159, 9.000000000000001776 ) ) ;
#32962=AXIS2_PLACEMENT_3D ( 'NONE', #29283, #9846, #12886 ) ;
#32963=CARTESIAN_POINT ( 'NONE',  ( 4.003793318659404576, 8.455722206104576699, 10.49999999999999822 ) ) ;
#32967=ADVANCED_FACE ( 'NONE', ( #32464 ), #32255, .F. ) ;
#32969=DIRECTION ( 'NONE',  ( -0.000000000000000000, -0.000000000000000000, -1.000000000000000000 ) ) ;
#32973=CARTESIAN_POINT ( 'NONE',  ( -2.806807826039844578, 9.295007390093649846, 7.000000000000000000 ) ) ;
#32974=VECTOR ( 'NONE', #1238, 1000.000000000000114 ) ;
#32975=DIRECTION ( 'NONE',  ( 1.000000000000000000, 0.000000000000000000, 0.000000000000000000 ) ) ;
#32976=CARTESIAN_POINT ( 'NONE',  ( 2.109203785269305964, 7.931710454523196674, 10.49999999999999822 ) ) ;
#32977=EDGE_LOOP ( 'NONE', ( #38832, #15725, #30837, #15459, #25487 ) ) ;
#32979=AXIS2_PLACEMENT_3D ( 'NONE', #19852, #28184, #361 ) ;
#32980=ORIENTED_EDGE ( 'NONE', *, *, #19282, .T. ) ;
#32983=EDGE_CURVE ( 'NONE', #22904, #1365, #15378, .T. ) ;
#32985=CARTESIAN_POINT ( 'NONE',  ( -14.14332487906608549, 26.04398259919136294, 10.49999999999999822 ) ) ;
#32989=EDGE_LOOP ( 'NONE', ( #18547, #3682, #15803, #32816 ) ) ;
#32990=AXIS2_PLACEMENT_3D ( 'NONE', #33214, #11465, #24053 ) ;
#32992=CYLINDRICAL_SURFACE ( 'NONE', #19241, 0.5000000000000004441 ) ;
#32996=ORIENTED_EDGE ( 'NONE', *, *, #35228, .T. ) ;
#33002=CARTESIAN_POINT ( 'NONE',  ( -12.68475447279705470, 27.14725768220950641, 9.500000000000000000 ) ) ;
#33005=ORIENTED_EDGE ( 'NONE', *, *, #16612, .T. ) ;
#33008=EDGE_CURVE ( 'NONE', #38994, #17440, #10512, .T. ) ;
#33011=ORIENTED_EDGE ( 'NONE', *, *, #29898, .T. ) ;
#33017=VECTOR ( 'NONE', #14103, 1000.000000000000000 ) ;
#33018=EDGE_CURVE ( 'NONE', #19729, #25837, #39884, .T. ) ;
#33020=FACE_OUTER_BOUND ( 'NONE', #24799, .T. ) ;
#33021=LINE ( 'NONE', #30158, #2850 ) ;
#33022=EDGE_CURVE ( 'NONE', #21064, #16758, #7456, .T. ) ;
#33029=DIRECTION ( 'NONE',  ( -0.000000000000000000, -0.000000000000000000, -1.000000000000000000 ) ) ;
#33030=DIRECTION ( 'NONE',  ( 0.000000000000000000, 0.000000000000000000, 1.000000000000000000 ) ) ;
#33039=CARTESIAN_POINT ( 'NONE',  ( -14.86131180699622334, 21.44076732726277967, 10.82238861112337247 ) ) ;
#33040=ORIENTED_EDGE ( 'NONE', *, *, #24968, .T. ) ;
#33042=LINE ( 'NONE', #36076, #32211 ) ;
#33046=AXIS2_PLACEMENT_3D ( 'NONE', #19018, #21467, #28159 ) ;
#33049=CARTESIAN_POINT ( 'NONE',  ( 4.984135866956514782, 36.15314577889351000, 10.49999999999999822 ) ) ;
#33051=ORIENTED_EDGE ( 'NONE', *, *, #22309, .T. ) ;
#33054=DIRECTION ( 'NONE',  ( -0.2876062384759514590, -0.6459741880212531706, -0.7071067811865452413 ) ) ;
#33055=CARTESIAN_POINT ( 'NONE',  ( 0.000000000000000000, 22.50000000000000355, 7.000000000000000000 ) ) ;
#33056=AXIS2_PLACEMENT_3D ( 'NONE', #4718, #28894, #1271 ) ;
#33060=FACE_OUTER_BOUND ( 'NONE', #37081, .T. ) ;
#33062=CYLINDRICAL_SURFACE ( 'NONE', #35578, 5.999999999999996447 ) ;
#33064=FACE_OUTER_BOUND ( 'NONE', #13022, .T. ) ;
#33065=EDGE_LOOP ( 'NONE', ( #27205, #2860, #11992 ) ) ;
#33068=DIRECTION ( 'NONE',  ( 1.000000000000000000, 0.000000000000000000, 0.000000000000000000 ) ) ;
#33069=ORIENTED_EDGE ( 'NONE', *, *, #4143, .F. ) ;
#33071=CARTESIAN_POINT ( 'NONE',  ( -5.440908595777636414, 35.94977745735568675, 7.500000000000000888 ) ) ;
#33072=CARTESIAN_POINT ( 'NONE',  ( -13.03339520833720222, 15.55251603720152431, 10.94611345180490680 ) ) ;
#33075=CARTESIAN_POINT ( 'NONE',  ( -12.05736835487443237, 14.38397459621567442, 9.500000000000000000 ) ) ;
#33076=LINE ( 'NONE', #36314, #37270 ) ;
#33077=CARTESIAN_POINT ( 'NONE',  ( 13.48130249190479191, 27.93180293473185927, 10.50000000000000533 ) ) ;
#33079=DIRECTION ( 'NONE',  ( -0.2876062384759508483, -0.6459741880212497289, -0.7071067811865486830 ) ) ;
#33080=ORIENTED_EDGE ( 'NONE', *, *, #3348, .F. ) ;
#33082=DIRECTION ( 'NONE',  ( 0.000000000000000000, 0.000000000000000000, 1.000000000000000000 ) ) ;
#33083=CARTESIAN_POINT ( 'NONE',  ( -14.02836544648977579, 27.77630492435593013, 10.49999999999999822 ) ) ;
#33085=CARTESIAN_POINT ( 'NONE',  ( -3.503793317224517700, 8.420815634768727520, 7.000000000000000000 ) ) ;
#33087=DIRECTION ( 'NONE',  ( -0.2079116908177663092, -0.9781476007338041345, 0.000000000000000000 ) ) ;
#33093=CARTESIAN_POINT ( 'NONE',  ( -9.771904059883794957, 33.31711103041964606, 7.000000000000000000 ) ) ;
#33094=ORIENTED_EDGE ( 'NONE', *, *, #17972, .F. ) ;
#33098=DIRECTION ( 'NONE',  ( -0.000000000000000000, -0.000000000000000000, -1.000000000000000000 ) ) ;
#33100=LINE ( 'NONE', #27190, #28443 ) ;
#33102=CARTESIAN_POINT ( 'NONE',  ( 9.428145666828122273, 11.00786382055638768, 10.49999999999999822 ) ) ;
#33103=AXIS2_PLACEMENT_3D ( 'NONE', #38339, #16616, #7662 ) ;
#33104=ORIENTED_EDGE ( 'NONE', *, *, #6313, .T. ) ;
#33106=ORIENTED_EDGE ( 'NONE', *, *, #32983, .F. ) ;
#33108=EDGE_CURVE ( 'NONE', #33983, #24685, #14964, .T. ) ;
#33110=CARTESIAN_POINT ( 'NONE',  ( 13.74617375768325900, 27.96120515612769708, 10.49999999999999822 ) ) ;
#33111=ORIENTED_EDGE ( 'NONE', *, *, #6896, .T. ) ;
#33112=EDGE_CURVE ( 'NONE', #29442, #7636, #5614, .T. ) ;
#33114=CARTESIAN_POINT ( 'NONE',  ( 6.354454053420414361, 35.54304081427980577, 11.00000000000000000 ) ) ;
#33115=DIRECTION ( 'NONE',  ( -0.000000000000000000, -0.000000000000000000, 1.000000000000000000 ) ) ;
#33117=FACE_OUTER_BOUND ( 'NONE', #13721, .T. ) ;
#33122=ORIENTED_EDGE ( 'NONE', *, *, #25537, .F. ) ;
#33124=CARTESIAN_POINT ( 'NONE',  ( 10.44103466624280507, 32.57396620494213124, 11.00000000000000000 ) ) ;
#33126=ADVANCED_FACE ( 'NONE', ( #18025 ), #27354, .T. ) ;
#33127=EDGE_CURVE ( 'NONE', #20195, #36614, #20674, .T. ) ;
#33130=VECTOR ( 'NONE', #5169, 1000.000000000000000 ) ;
#33131=LINE ( 'NONE', #14832, #19861 ) ;
#33135=CARTESIAN_POINT ( 'NONE',  ( -9.381156159426771168, 10.79514327830607101, 7.482036690254806111 ) ) ;
#33136=VERTEX_POINT ( 'NONE', #33472 ) ;
#33137=ORIENTED_EDGE ( 'NONE', *, *, #22554, .F. ) ;
#33139=DIRECTION ( 'NONE',  ( 0.000000000000000000, 0.000000000000000000, -1.000000000000000000 ) ) ;
#33142=DIRECTION ( 'NONE',  ( -0.8660254037844425934, -0.4999999999999933942, 0.000000000000000000 ) ) ;
#33147=FACE_OUTER_BOUND ( 'NONE', #12307, .T. ) ;
#33148=CARTESIAN_POINT ( 'NONE',  ( -2.444768620640030754, 7.712926687590090147, 10.49999999999999822 ) ) ;
#33151=B_SPLINE_CURVE_WITH_KNOTS ( 'NONE', 3,
 ( #10119, #29207, #31850, #1378 ),
 .UNSPECIFIED., .F., .F.,
 ( 4, 4 ),
 ( 0.000000000000000000, 1.000000000000000000 ),
 .UNSPECIFIED. ) ;
#33152=ADVANCED_FACE ( 'NONE', ( #30416 ), #39255, .T. ) ;
#33153=DIRECTION ( 'NONE',  ( 0.000000000000000000, 0.000000000000000000, -1.000000000000000000 ) ) ;
#33154=ORIENTED_EDGE ( 'NONE', *, *, #14847, .T. ) ;
#33157=ORIENTED_EDGE ( 'NONE', *, *, #6409, .F. ) ;
#33159=B_SPLINE_CURVE_WITH_KNOTS ( 'NONE', 3,
 ( #20909, #33716, #26800, #17677 ),
 .UNSPECIFIED., .F., .F.,
 ( 4, 4 ),
 ( 0.000000000000000000, 1.000000000000000000 ),
 .UNSPECIFIED. ) ;
#33160=CIRCLE ( 'NONE', #14318, 1.000000000000016431 ) ;
#33169=AXIS2_PLACEMENT_3D ( 'NONE', #36601, #5913, #21361 ) ;
#33172=CONICAL_SURFACE ( 'NONE', #7191, 1.000000000000000888, 0.7853981633974552734 ) ;
#33173=EDGE_CURVE ( 'NONE', #33798, #35217, #33272, .T. ) ;
#33175=DIRECTION ( 'NONE',  ( -1.000000000000000000, 0.000000000000000000, 0.000000000000000000 ) ) ;
#33176=CARTESIAN_POINT ( 'NONE',  ( 9.221287281574507944, 10.65863771052197784, 11.00000000000000000 ) ) ;
#33178=ORIENTED_EDGE ( 'NONE', *, *, #3666, .T. ) ;
#33180=ORIENTED_EDGE ( 'NONE', *, *, #33660, .F. ) ;
#33187=AXIS2_PLACEMENT_3D ( 'NONE', #20916, #5664, #30466 ) ;
#33192=CARTESIAN_POINT ( 'NONE',  ( 14.85188145504474022, 20.30462949162087938, 10.49999999999999645 ) ) ;
#33196=CARTESIAN_POINT ( 'NONE',  ( -5.184280209938394890, 31.68549066217158483, 10.50000000000000355 ) ) ;
#33203=EDGE_CURVE ( 'NONE', #34486, #25343, #7497, .T. ) ;
#33204=ORIENTED_EDGE ( 'NONE', *, *, #15000, .F. ) ;
#33206=VECTOR ( 'NONE', #25544, 1000.000000000000114 ) ;
#33207=ADVANCED_FACE ( 'NONE', ( #11721 ), #36707, .T. ) ;
#33209=VECTOR ( 'NONE', #3263, 1000.000000000000000 ) ;
#33211=EDGE_CURVE ( 'NONE', #11176, #34232, #24108, .T. ) ;
#33213=CARTESIAN_POINT ( 'NONE',  ( 7.096882951594525757, 29.56287847632727050, 10.00000000000000000 ) ) ;
#33214=CARTESIAN_POINT ( 'NONE',  ( 1.000000000000000000, 37.50000000000000711, 10.50000000000000178 ) ) ;
#33215=EDGE_CURVE ( 'NONE', #4297, #37780, #14568, .T. ) ;
#33216=CYLINDRICAL_SURFACE ( 'NONE', #8356, 0.5000000000000000000 ) ;
#33217=VECTOR ( 'NONE', #35782, 1000.000000000000000 ) ;
#33219=DIRECTION ( 'NONE',  ( -1.000000000000000000, 0.000000000000000000, 0.000000000000000000 ) ) ;
#33221=ORIENTED_EDGE ( 'NONE', *, *, #11983, .F. ) ;
#33224=CARTESIAN_POINT ( 'NONE',  ( 9.221287281574507944, 10.65863771052197784, 10.49999999999999822 ) ) ;
#33227=CARTESIAN_POINT ( 'NONE',  ( 2.525645716490518389, 8.212903943950921715, 7.000000000000000000 ) ) ;
#33229=EDGE_CURVE ( 'NONE', #38194, #31599, #30209, .T. ) ;
#33232=ORIENTED_EDGE ( 'NONE', *, *, #39274, .T. ) ;
#33236=CYLINDRICAL_SURFACE ( 'NONE', #23040, 6.000000000000001776 ) ;
#33239=CARTESIAN_POINT ( 'NONE',  ( 12.30736835487432757, 14.81698729810772441, 7.000000000000000000 ) ) ;
#33240=ORIENTED_EDGE ( 'NONE', *, *, #18293, .T. ) ;
#33242=CARTESIAN_POINT ( 'NONE',  ( -12.74038105676665289, 14.56698729810790027, 11.00000000000000000 ) ) ;
#33244=CARTESIAN_POINT ( 'NONE',  ( 7.848705329595008884, 10.27943253798616219, 10.66666666666666075 ) ) ;
#33249=EDGE_LOOP ( 'NONE', ( #27838, #5206, #25540 ) ) ;
#33252=AXIS2_PLACEMENT_3D ( 'NONE', #4648, #29430, #1606 ) ;
#33254=CARTESIAN_POINT ( 'NONE',  ( -13.94482798346716201, 26.50521816028930644, 9.000000000000001776 ) ) ;
#33255=ORIENTED_EDGE ( 'NONE', *, *, #916, .F. ) ;
#33257=EDGE_CURVE ( 'NONE', #39980, #13142, #13861, .T. ) ;
#33260=DIRECTION ( 'NONE',  ( 0.9510565162951544194, 0.3090169943749449533, -0.000000000000000000 ) ) ;
#33263=LINE ( 'NONE', #36697, #26806 ) ;
#33265=EDGE_CURVE ( 'NONE', #31717, #7910, #22134, .T. ) ;
#33266=VECTOR ( 'NONE', #35612, 1000.000000000000000 ) ;
#33267=ORIENTED_EDGE ( 'NONE', *, *, #38933, .T. ) ;
#33270=ORIENTED_EDGE ( 'NONE', *, *, #24059, .F. ) ;
#33272=LINE ( 'NONE', #5819, #16556 ) ;
#33273=DIRECTION ( 'NONE',  ( -0.000000000000000000, 1.000000000000000000, -0.000000000000000000 ) ) ;
#33275=PLANE ( 'NONE',  #10308 ) ;
#33276=DIRECTION ( 'NONE',  ( -0.000000000000000000, -0.000000000000000000, 1.000000000000000000 ) ) ;
#33277=CARTESIAN_POINT ( 'NONE',  ( 12.42073081513896327, 14.75153745115793313, 11.00000000000000000 ) ) ;
#33281=CARTESIAN_POINT ( 'NONE',  ( 9.365580931528452169, 10.78282772046311599, 7.485646746502377269 ) ) ;
#33282=ORIENTED_EDGE ( 'NONE', *, *, #28179, .F. ) ;
#33285=PLANE ( 'NONE',  #9045 ) ;
#33286=DIRECTION ( 'NONE',  ( 1.000000000000000000, 0.000000000000000000, 0.000000000000000000 ) ) ;
#33291=PLANE ( 'NONE',  #5696 ) ;
#33299=VECTOR ( 'NONE', #36264, 1000.000000000000114 ) ;
#33302=EDGE_CURVE ( 'NONE', #16943, #8916, #30855, .T. ) ;
#33303=PLANE ( 'NONE',  #8994 ) ;
#33304=AXIS2_PLACEMENT_3D ( 'NONE', #3267, #21551, #34749 ) ;
#33308=AXIS2_PLACEMENT_3D ( 'NONE', #26515, #1942, #32620 ) ;
#33309=ORIENTED_EDGE ( 'NONE', *, *, #1920, .F. ) ;
#33312=ORIENTED_EDGE ( 'NONE', *, *, #9062, .F. ) ;
#33313=DIRECTION ( 'NONE',  ( 1.000000000000000000, 0.000000000000000000, 0.000000000000000000 ) ) ;
#33314=DIRECTION ( 'NONE',  ( 0.000000000000000000, 0.000000000000000000, -1.000000000000000000 ) ) ;
#33316=DIRECTION ( 'NONE',  ( 0.4999999999999921174, -0.8660254037844431485, -0.000000000000000000 ) ) ;
#33317=ORIENTED_EDGE ( 'NONE', *, *, #39419, .T. ) ;
#33319=CARTESIAN_POINT ( 'NONE',  ( 13.47830981910552062, 21.58612669357077607, 9.500000000000000000 ) ) ;
#33320=FACE_OUTER_BOUND ( 'NONE', #14418, .T. ) ;
#33327=CARTESIAN_POINT ( 'NONE',  ( -6.354454053420248272, 35.54304081427989814, 9.000000000000001776 ) ) ;
#33329=ADVANCED_FACE ( 'NONE', ( #6406 ), #21109, .T. ) ;
#33332=CARTESIAN_POINT ( 'NONE',  ( -6.101049646136835314, 36.20318186463909882, 7.000000000000000000 ) ) ;
#33333=EDGE_CURVE ( 'NONE', #24423, #19575, #28545, .T. ) ;
#33336=VECTOR ( 'NONE', #6058, 1000.000000000000000 ) ;
#33339=CARTESIAN_POINT ( 'NONE',  ( 11.48173768534036121, 32.16538668264416145, 10.49999999999999822 ) ) ;
#33340=EDGE_CURVE ( 'NONE', #9244, #23354, #34732, .T. ) ;
#33341=VERTEX_POINT ( 'NONE', #34256 ) ;
#33342=ORIENTED_EDGE ( 'NONE', *, *, #30842, .T. ) ;
#33345=CARTESIAN_POINT ( 'NONE',  ( -12.99377146717201015, 26.19620116591435632, 9.500000000000000000 ) ) ;
#33346=AXIS2_PLACEMENT_3D ( 'NONE', #28339, #38490, #22238 ) ;
#33347=DIRECTION ( 'NONE',  ( -0.2876062384759501267, -0.6459741880212528375, -0.7071067811865461294 ) ) ;
#33350=DIRECTION ( 'NONE',  ( -1.000000000000000000, 0.000000000000000000, 0.000000000000000000 ) ) ;
#33351=CARTESIAN_POINT ( 'NONE',  ( -2.291516524179419978, 7.763791616332306411, 10.49999999999999822 ) ) ;
#33354=FACE_OUTER_BOUND ( 'NONE', #30428, .T. ) ;
#33355=ORIENTED_EDGE ( 'NONE', *, *, #13497, .F. ) ;
#33357=CIRCLE ( 'NONE', #5444, 0.5000000000000000000 ) ;
#33365=CIRCLE ( 'NONE', #15829, 0.4999999999999993339 ) ;
#33366=DIRECTION ( 'NONE',  ( 0.9945218953682730678, -0.1045284632676569819, 0.000000000000000000 ) ) ;
#33372=VECTOR ( 'NONE', #31453, 1000.000000000000000 ) ;
#33377=CARTESIAN_POINT ( 'NONE',  ( 11.11016527260166420, 31.83082137946473367, 7.499999999999997335 ) ) ;
#33378=LINE ( 'NONE', #5522, #13551 ) ;
#33380=ORIENTED_EDGE ( 'NONE', *, *, #39678, .F. ) ;
#33382=CONICAL_SURFACE ( 'NONE', #28171, 1.000000000000002665, 0.7853981633974548293 ) ;
#33383=EDGE_LOOP ( 'NONE', ( #2092, #11255, #5784, #3105 ) ) ;
#33387=CARTESIAN_POINT ( 'NONE',  ( -3.900351417861621428, 8.105760029628179097, 10.49999999999999822 ) ) ;
#33389=EDGE_CURVE ( 'NONE', #25420, #31354, #11921, .T. ) ;
#33390=EDGE_LOOP ( 'NONE', ( #12100, #29386, #37922, #38931 ) ) ;
#33392=VERTEX_POINT ( 'NONE', #19200 ) ;
#33394=DIRECTION ( 'NONE',  ( 0.000000000000000000, -0.000000000000000000, -1.000000000000000000 ) ) ;
#33406=VERTEX_POINT ( 'NONE', #25486 ) ;
#33411=ADVANCED_FACE ( 'NONE', ( #25100 ), #37886, .T. ) ;
#33414=EDGE_CURVE ( 'NONE', #19420, #40188, #6996, .T. ) ;
#33415=CIRCLE ( 'NONE', #26088, 1.000000000000002665 ) ;
#33416=CARTESIAN_POINT ( 'NONE',  ( 0.5000000000000004441, 36.00000000000000711, 9.500000000000000000 ) ) ;
#33419=CARTESIAN_POINT ( 'NONE',  ( 14.47283171447379502, 21.48159823030311344, 7.000000000000000000 ) ) ;
#33420=CARTESIAN_POINT ( 'NONE',  ( -3.161220354320351422, 12.43736188311283897, 11.00000000000000000 ) ) ;
#33421=VECTOR ( 'NONE', #20029, 1000.000000000000114 ) ;
#33428=DIRECTION ( 'NONE',  ( 1.000000000000000000, 0.000000000000000000, 0.000000000000000000 ) ) ;
#33430=CARTESIAN_POINT ( 'NONE',  ( -9.997483185316568211, 21.95197631500770186, 10.49999999999999289 ) ) ;
#33431=EDGE_CURVE ( 'NONE', #4287, #34838, #523, .T. ) ;
#33439=EDGE_LOOP ( 'NONE', ( #23993, #23484, #28778 ) ) ;
#33445=CARTESIAN_POINT ( 'NONE',  ( 8.118377661053333583, 10.47536095541699197, 11.00000000000000000 ) ) ;
#33446=AXIS2_PLACEMENT_3D ( 'NONE', #17036, #20082, #22910 ) ;
#33451=ORIENTED_EDGE ( 'NONE', *, *, #19600, .F. ) ;
#33460=VECTOR ( 'NONE', #14620, 1000.000000000000000 ) ;
#33461=AXIS2_PLACEMENT_3D ( 'NONE', #5689, #36574, #5890 ) ;
#33462=CARTESIAN_POINT ( 'NONE',  ( 5.187504188494417079, 36.60991850771481637, 10.50000000000000000 ) ) ;
#33464=PLANE ( 'NONE',  #9300 ) ;
#33468=CARTESIAN_POINT ( 'NONE',  ( 14.99771543937018414, 22.21207258816060559, 7.102637441331453694 ) ) ;
#33469=CARTESIAN_POINT ( 'NONE',  ( 6.830039222088956308, 35.38192592444566742, 10.49999999999999822 ) ) ;
#33472=CARTESIAN_POINT ( 'NONE',  ( -3.914034194965524183, 30.06176806842423943, 7.000000000000000000 ) ) ;
#33474=LINE ( 'NONE', #30420, #28489 ) ;
#33475=CARTESIAN_POINT ( 'NONE',  ( -14.96930490892015797, 21.54088032874991399, 7.500000000000004441 ) ) ;
#33476=DIRECTION ( 'NONE',  ( -0.000000000000000000, -0.000000000000000000, -1.000000000000000000 ) ) ;
#33477=EDGE_CURVE ( 'NONE', #18376, #9166, #24903, .T. ) ;
#33478=CARTESIAN_POINT ( 'NONE',  ( 6.354454053420414361, 35.54304081427980577, 7.000000000000000000 ) ) ;
#33480=LINE ( 'NONE', #36317, #26902 ) ;
#33481=VECTOR ( 'NONE', #26092, 999.9999999999998863 ) ;
#33482=ORIENTED_EDGE ( 'NONE', *, *, #11685, .T. ) ;
#33484=LINE ( 'NONE', #23721, #25879 ) ;
#33485=CIRCLE ( 'NONE', #30249, 0.9999999999999995559 ) ;
#33486=FACE_OUTER_BOUND ( 'NONE', #31024, .T. ) ;
#33487=EDGE_CURVE ( 'NONE', #20155, #31096, #4361, .T. ) ;
#33491=ORIENTED_EDGE ( 'NONE', *, *, #14614, .T. ) ;
#33492=CARTESIAN_POINT ( 'NONE',  ( 7.118377661053320260, 10.47536095541698486, 7.000000000000000000 ) ) ;
#33493=DIRECTION ( 'NONE',  ( 1.000000000000000000, 0.000000000000000000, 0.000000000000000000 ) ) ;
#33499=CARTESIAN_POINT ( 'NONE',  ( 1.693998953219512105, 12.12549434688614625, 11.00000000000000000 ) ) ;
#33504=ORIENTED_EDGE ( 'NONE', *, *, #16846, .F. ) ;
#33506=DIRECTION ( 'NONE',  ( -0.000000000000000000, -0.000000000000000000, 1.000000000000000000 ) ) ;
#33510=EDGE_CURVE ( 'NONE', #1570, #12591, #35850, .T. ) ;
#33511=AXIS2_PLACEMENT_3D ( 'NONE', #18387, #18192, #2940 ) ;
#33512=AXIS2_PLACEMENT_3D ( 'NONE', #24515, #8484, #17844 ) ;
#33514=CARTESIAN_POINT ( 'NONE',  ( -2.036571916123810055, 8.108948098542073879, 10.49999999999999822 ) ) ;
#33515=ORIENTED_EDGE ( 'NONE', *, *, #19587, .F. ) ;
#33516=CARTESIAN_POINT ( 'NONE',  ( 14.97283170755579818, 21.46414480565946903, 10.49999999999999822 ) ) ;
#33517=CARTESIAN_POINT ( 'NONE',  ( 9.625795778761983001, 10.95253033666821274, 10.50000000000000000 ) ) ;
#33518=CARTESIAN_POINT ( 'NONE',  ( -2.568190708544555001, 12.82247983807085134, 10.50000000000000533 ) ) ;
#33519=ORIENTED_EDGE ( 'NONE', *, *, #27995, .T. ) ;
#33521=CYLINDRICAL_SURFACE ( 'NONE', #39683, 0.5000000000000004441 ) ;
#33522=FACE_OUTER_BOUND ( 'NONE', #18385, .T. ) ;
#33524=EDGE_CURVE ( 'NONE', #6233, #22876, #25890, .T. ) ;
#33529=CARTESIAN_POINT ( 'NONE',  ( -4.678013043399448456, 44.50832101651065642, 7.000000000000000000 ) ) ;
#33540=EDGE_LOOP ( 'NONE', ( #35783, #28111, #21549, #8425 ) ) ;
#33545=DIRECTION ( 'NONE',  ( 1.000000000000000000, 3.469446951953598806E-15, 0.000000000000000000 ) ) ;
#33549=CARTESIAN_POINT ( 'NONE',  ( 13.62967667376826419, 40.40898974728997217, 11.00000000000000000 ) ) ;
#33550=EDGE_LOOP ( 'NONE', ( #36238, #15147, #25676 ) ) ;
#33552=FACE_OUTER_BOUND ( 'NONE', #29431, .T. ) ;
#33558=EDGE_CURVE ( 'NONE', #3451, #5601, #25640, .T. ) ;
#33563=CARTESIAN_POINT ( 'NONE',  ( 10.70158575030369796, 30.79011836036717753, 10.00000000000000000 ) ) ;
#33565=CARTESIAN_POINT ( 'NONE',  ( 10.81260707898150386, 32.90853150812155548, 10.49999999999999822 ) ) ;
#33568=CARTESIAN_POINT ( 'NONE',  ( -9.151574469205524309, 1.945227203041487218, 7.000000000000000000 ) ) ;
#33571=DIRECTION ( 'NONE',  ( 1.000000000000000000, 0.000000000000000000, 0.000000000000000000 ) ) ;
#33572=DIRECTION ( 'NONE',  ( -0.7071067811865493491, 0.000000000000000000, -0.7071067811865456854 ) ) ;
#33576=ORIENTED_EDGE ( 'NONE', *, *, #27498, .T. ) ;
#33580=CARTESIAN_POINT ( 'NONE',  ( -3.607749162633349105, 7.931741834401817570, 10.59344459855560316 ) ) ;
#33582=ORIENTED_EDGE ( 'NONE', *, *, #19085, .T. ) ;
#33586=CARTESIAN_POINT ( 'NONE',  ( 8.412270287199559604, 10.07085245822950981, 10.50000000000000178 ) ) ;
#33591=ORIENTED_EDGE ( 'NONE', *, *, #19694, .F. ) ;
#33595=ORIENTED_EDGE ( 'NONE', *, *, #5391, .F. ) ;
#33599=AXIS2_PLACEMENT_3D ( 'NONE', #6985, #19391, #31787 ) ;
#33604=VECTOR ( 'NONE', #36687, 999.9999999999998863 ) ;
#33606=EDGE_CURVE ( 'NONE', #9581, #18534, #32612, .T. ) ;
#33607=ORIENTED_EDGE ( 'NONE', *, *, #10096, .T. ) ;
#33612=EDGE_CURVE ( 'NONE', #37387, #36832, #4894, .T. ) ;
#33613=DIRECTION ( 'NONE',  ( 0.8090169943749504489, 0.5877852522924690293, -0.000000000000000000 ) ) ;
#33614=EDGE_CURVE ( 'NONE', #5349, #10226, #26507, .T. ) ;
#33615=B_SPLINE_CURVE_WITH_KNOTS ( 'NONE', 3,
 ( #36793, #8970, #21357, #36004, #20569, #2079 ),
 .UNSPECIFIED., .F., .F.,
 ( 4, 2, 4 ),
 ( 0.000000000000000000, 0.5000000000000000000, 1.000000000000000000 ),
 .UNSPECIFIED. ) ;
#33616=CIRCLE ( 'NONE', #7642, 0.5000000000000004441 ) ;
#33619=DIRECTION ( 'NONE',  ( -0.7431448254773953543, -0.6691306063588570163, 0.000000000000000000 ) ) ;
#33620=ORIENTED_EDGE ( 'NONE', *, *, #27200, .F. ) ;
#33626=CYLINDRICAL_SURFACE ( 'NONE', #817, 6.000000000000003553 ) ;
#33628=CIRCLE ( 'NONE', #9630, 0.5000000000000004441 ) ;
#33633=EDGE_CURVE ( 'NONE', #21531, #19894, #16769, .T. ) ;
#33634=ADVANCED_FACE ( 'NONE', ( #38898 ), #38698, .T. ) ;
#33635=FACE_OUTER_BOUND ( 'NONE', #27092, .T. ) ;
#33637=ORIENTED_EDGE ( 'NONE', *, *, #34932, .F. ) ;
#33638=CARTESIAN_POINT ( 'NONE',  ( -14.84898236231945745, 21.81673761604096384, 10.49999999999999822 ) ) ;
#33641=CARTESIAN_POINT ( 'NONE',  ( 7.468455364333220103, 29.89744377950669474, 10.50000000000000000 ) ) ;
#33646=CARTESIAN_POINT ( 'NONE',  ( 1.000000000000000000, 37.00000000000000711, 11.00000000000000000 ) ) ;
#33652=FACE_OUTER_BOUND ( 'NONE', #38011, .T. ) ;
#33653=ORIENTED_EDGE ( 'NONE', *, *, #31537, .T. ) ;
#33656=AXIS2_PLACEMENT_3D ( 'NONE', #38069, #25873, #22625 ) ;
#33659=AXIS2_PLACEMENT_3D ( 'NONE', #23255, #38894, #17375 ) ;
#33660=EDGE_CURVE ( 'NONE', #3751, #23354, #7608, .T. ) ;
#33662=CARTESIAN_POINT ( 'NONE',  ( -11.61016527260153808, 31.83082137946488643, 7.500000000000004441 ) ) ;
#33663=VECTOR ( 'NONE', #31630, 1000.000000000000000 ) ;
#33665=PLANE ( 'NONE',  #23634 ) ;
#33666=CARTESIAN_POINT ( 'NONE',  ( 14.36830325120613594, 20.48707633493483371, 7.000000000000000000 ) ) ;
#33667=CARTESIAN_POINT ( 'NONE',  ( -4.727507481117093846, 31.88885898370948269, 10.00000000000000000 ) ) ;
#33669=CARTESIAN_POINT ( 'NONE',  ( -6.282361020112269046, 14.70372268239681546, 10.50000000000000178 ) ) ;
#33671=DIRECTION ( 'NONE',  ( 1.000000000000000000, 0.000000000000000000, -0.000000000000000000 ) ) ;
#33673=DIRECTION ( 'NONE',  ( 1.000000000000000000, 0.000000000000000000, 0.000000000000000000 ) ) ;
#33677=CARTESIAN_POINT ( 'NONE',  ( 0.5000000000000035527, 32.50000000000000000, 10.50000000000000178 ) ) ;
#33679=VERTEX_POINT ( 'NONE', #920 ) ;
#33681=DIRECTION ( 'NONE',  ( -0.1277282058445971258, 0.8064441531181095746, 0.5773502691896276184 ) ) ;
#33682=CARTESIAN_POINT ( 'NONE',  ( -11.62435565298221185, 14.63397459621566910, 9.500000000000000000 ) ) ;
#33687=B_SPLINE_CURVE_WITH_KNOTS ( 'NONE', 3,
 ( #16533, #6767, #687, #25661, #16940, #13473 ),
 .UNSPECIFIED., .F., .F.,
 ( 4, 2, 4 ),
 ( 0.000000000000000000, 0.5000000000000000000, 1.000000000000000000 ),
 .UNSPECIFIED. ) ;
#33690=LINE ( 'NONE', #12727, #10785 ) ;
#33701=ORIENTED_EDGE ( 'NONE', *, *, #26921, .T. ) ;
#33702=CARTESIAN_POINT ( 'NONE',  ( 1.734965421685031872, 7.600674680189132282, 7.000000000000000000 ) ) ;
#33703=LINE ( 'NONE', #9506, #8319 ) ;
#33705=EDGE_CURVE ( 'NONE', #5508, #7975, #4653, .T. ) ;
#33709=EDGE_CURVE ( 'NONE', #29758, #29828, #26967, .T. ) ;
#33710=EDGE_LOOP ( 'NONE', ( #22969, #39601, #34926 ) ) ;
#33711=ADVANCED_FACE ( 'NONE', ( #30363 ), #31489, .T. ) ;
#33712=CARTESIAN_POINT ( 'NONE',  ( 3.000488737323008248, 30.46850471149999962, 7.000000000000000000 ) ) ;
#33716=CARTESIAN_POINT ( 'NONE',  ( 6.658969205967948390, 35.40746193325453817, 10.66666666666666430 ) ) ;
#33717=EDGE_CURVE ( 'NONE', #32632, #16758, #9457, .T. ) ;
#33718=DIRECTION ( 'NONE',  ( -1.000000000000000000, 0.000000000000000000, 0.000000000000000000 ) ) ;
#33721=CYLINDRICAL_SURFACE ( 'NONE', #5526, 0.5000000000000004441 ) ;
#33722=FACE_OUTER_BOUND ( 'NONE', #24671, .T. ) ;
#33729=DIRECTION ( 'NONE',  ( 0.8090169943749426773, -0.5877852522924797984, 0.000000000000000000 ) ) ;
#33731=CARTESIAN_POINT ( 'NONE',  ( 13.46929972531963848, 26.35070966310165375, 10.00000000000000000 ) ) ;
#33733=ADVANCED_FACE ( 'NONE', ( #26704 ), #14917, .T. ) ;
#33737=CIRCLE ( 'NONE', #16202, 0.5000000000000004441 ) ;
#33740=DIRECTION ( 'NONE',  ( 0.000000000000000000, 0.000000000000000000, -1.000000000000000000 ) ) ;
#33741=ORIENTED_EDGE ( 'NONE', *, *, #4115, .T. ) ;
#33742=ORIENTED_EDGE ( 'NONE', *, *, #25374, .T. ) ;
#33747=CARTESIAN_POINT ( 'NONE',  ( -9.665073660138979506, 25.11464168560200605, 10.49999999999999112 ) ) ;
#33750=CARTESIAN_POINT ( 'NONE',  ( -13.94482798346716201, 26.50521816028930999, 7.499999999999993783 ) ) ;
#33752=ORIENTED_EDGE ( 'NONE', *, *, #18311, .F. ) ;
#33754=DIRECTION ( 'NONE',  ( 0.000000000000000000, 0.000000000000000000, 1.000000000000000000 ) ) ;
#33755=EDGE_CURVE ( 'NONE', #39268, #37780, #39886, .T. ) ;
#33758=EDGE_CURVE ( 'NONE', #18974, #5349, #20820, .T. ) ;
#33759=EDGE_LOOP ( 'NONE', ( #20316, #37385, #6961, #11189 ) ) ;
#33764=CIRCLE ( 'NONE', #3238, 1.000000000000002665 ) ;
#33766=EDGE_LOOP ( 'NONE', ( #28685, #3854, #22853, #36725, #13538 ) ) ;
#33768=CARTESIAN_POINT ( 'NONE',  ( 3.503793317224326298, 8.420815634768676006, 9.500000000000000000 ) ) ;
#33769=VECTOR ( 'NONE', #4359, 1000.000000000000000 ) ;
#33771=DIRECTION ( 'NONE',  ( -1.000000000000000000, -1.224646799147351235E-16, 0.000000000000000000 ) ) ;
#33774=DIRECTION ( 'NONE',  ( 0.5821182788257952545, 0.000000000000000000, 0.8131041196900269385 ) ) ;
#33775=DIRECTION ( 'NONE',  ( 0.000000000000000000, -0.5906904945688840058, 0.8068982213550648375 ) ) ;
#33778=AXIS2_PLACEMENT_3D ( 'NONE', #15308, #14715, #24650 ) ;
#33781=CARTESIAN_POINT ( 'NONE',  ( 3.718716484603448613, 7.955328666817497840, 10.49999999999999822 ) ) ;
#33783=EDGE_LOOP ( 'NONE', ( #20015, #18277, #16727, #18081, #30076, #31362, #39652 ) ) ;
#33785=CARTESIAN_POINT ( 'NONE',  ( 8.016213763118591018, 9.982035245863860595, 10.49999999999999822 ) ) ;
#33788=CARTESIAN_POINT ( 'NONE',  ( 18.68254918188133473, 8.687943646703843115, 9.500000000000000000 ) ) ;
#33789=ORIENTED_EDGE ( 'NONE', *, *, #14642, .T. ) ;
#33793=ORIENTED_EDGE ( 'NONE', *, *, #20072, .T. ) ;
#33795=DIRECTION ( 'NONE',  ( -0.3090169943749448977, 0.9510565162951543083, 0.000000000000000000 ) ) ;
#33796=CARTESIAN_POINT ( 'NONE',  ( -19.23557158514982746, 34.18301270189230934, 11.00000000000000000 ) ) ;
#33797=AXIS2_PLACEMENT_3D ( 'NONE', #3073, #25396, #31503 ) ;
#33798=VERTEX_POINT ( 'NONE', #29951 ) ;
#33808=AXIS2_PLACEMENT_3D ( 'NONE', #5318, #11816, #24203 ) ;
#33810=AXIS2_PLACEMENT_3D ( 'NONE', #5821, #26754, #8674 ) ;
#33811=DIRECTION ( 'NONE',  ( 0.6916548014802246236, -0.1470157664652213536, -0.7071067811865437980 ) ) ;
#33813=CARTESIAN_POINT ( 'NONE',  ( -5.203512939752292787, 36.56867331639969620, 7.338691926023215295 ) ) ;
#33814=ORIENTED_EDGE ( 'NONE', *, *, #28478, .F. ) ;
#33819=TOROIDAL_SURFACE ( 'NONE', #1387, 1.000000000000000000, 0.5000000000000000000 ) ;
#33820=DIRECTION ( 'NONE',  ( -0.000000000000000000, -0.000000000000000000, 1.000000000000000000 ) ) ;
#33822=EDGE_LOOP ( 'NONE', ( #17975, #9779, #18103, #10343 ) ) ;
#33825=EDGE_CURVE ( 'NONE', #9944, #9209, #19151, .T. ) ;
#33826=DIRECTION ( 'NONE',  ( 0.9135454576426059736, 0.4067366430757887730, 0.000000000000000000 ) ) ;
#33832=FACE_OUTER_BOUND ( 'NONE', #22862, .T. ) ;
#33837=LINE ( 'NONE', #33646, #18327 ) ;
#33842=VECTOR ( 'NONE', #66, 1000.000000000000114 ) ;
#33844=DIRECTION ( 'NONE',  ( 0.2185080122244077161, -0.6724985119639543818, 0.7071067811865513475 ) ) ;
#33845=EDGE_CURVE ( 'NONE', #39810, #30652, #11471, .T. ) ;
#33846=PLANE ( 'NONE',  #6967 ) ;
#33850=CARTESIAN_POINT ( 'NONE',  ( 13.32151712420403555, 20.09434385051835648, 9.500000000000000000 ) ) ;
#33852=VERTEX_POINT ( 'NONE', #8215 ) ;
#33853=VECTOR ( 'NONE', #25182, 1000.000000000000114 ) ;
#33855=DIRECTION ( 'NONE',  ( 0.4067366430758010964, 0.9135454576426005335, 0.000000000000000000 ) ) ;
#33857=ADVANCED_FACE ( 'NONE', ( #24452 ), #8424, .F. ) ;
#33858=DIRECTION ( 'NONE',  ( 0.4999999999999912292, -0.8660254037844437036, 0.000000000000000000 ) ) ;
#33860=LINE ( 'NONE', #27551, #14935 ) ;
#33863=LINE ( 'NONE', #22241, #13659 ) ;
#33864=LINE ( 'NONE', #6015, #20064 ) ;
#33865=LINE ( 'NONE', #18421, #16713 ) ;
#33866=LINE ( 'NONE', #31401, #3454 ) ;
#33867=CARTESIAN_POINT ( 'NONE',  ( -5.537946624085890335, 36.44027069998196566, 7.500000000000000888 ) ) ;
#33870=ORIENTED_EDGE ( 'NONE', *, *, #33633, .F. ) ;
#33872=DIRECTION ( 'NONE',  ( -1.000000000000000000, 0.000000000000000000, 0.000000000000000000 ) ) ;
#33880=DIRECTION ( 'NONE',  ( -0.5877852522924791323, -0.8090169943749430104, 0.000000000000000000 ) ) ;
#33888=LINE ( 'NONE', #9891, #5011 ) ;
#33889=ADVANCED_FACE ( 'NONE', ( #5769 ), #26906, .T. ) ;
#33894=ORIENTED_EDGE ( 'NONE', *, *, #9465, .T. ) ;
#33901=AXIS2_PLACEMENT_3D ( 'NONE', #4095, #7336, #10401 ) ;
#33902=CYLINDRICAL_SURFACE ( 'NONE', #34944, 0.5000000000000004441 ) ;
#33903=ORIENTED_EDGE ( 'NONE', *, *, #35182, .T. ) ;
#33904=EDGE_CURVE ( 'NONE', #8719, #14392, #40041, .T. ) ;
#33905=CARTESIAN_POINT ( 'NONE',  ( 9.892954722048896699, 20.95745441963929068, 10.50000000000000355 ) ) ;
#33906=FACE_OUTER_BOUND ( 'NONE', #15919, .T. ) ;
#33907=CARTESIAN_POINT ( 'NONE',  ( -5.473344025737326923, 14.11593743010433499, 10.50000000000000000 ) ) ;
#33908=ORIENTED_EDGE ( 'NONE', *, *, #992, .T. ) ;
#33910=CARTESIAN_POINT ( 'NONE',  ( -3.666817917346822941, 8.455467583238350571, 10.83333333333333215 ) ) ;
#33911=CARTESIAN_POINT ( 'NONE',  ( 4.096822963000107620, 8.035697679810645866, 10.49999999999999289 ) ) ;
#33912=CARTESIAN_POINT ( 'NONE',  ( -8.118377661053486349, 10.47536095541708967, 11.00000000000000000 ) ) ;
#33918=CARTESIAN_POINT ( 'NONE',  ( 11.44134295108989186, 15.31698729810772797, 10.50000000000000000 ) ) ;
#33922=ADVANCED_FACE ( 'NONE', ( #6356 ), #15913, .T. ) ;
#33927=CARTESIAN_POINT ( 'NONE',  ( 11.28725060478870823, 31.99026972875169150, 10.94387467463331731 ) ) ;
#33930=CARTESIAN_POINT ( 'NONE',  ( -3.992867117591420545, 8.524771480177605554, 11.00000000000000000 ) ) ;
#33931=CARTESIAN_POINT ( 'NONE',  ( -8.412270287199726582, 10.07085245822961994, 10.49999999999999822 ) ) ;
#33932=CARTESIAN_POINT ( 'NONE',  ( -9.381390373407009875, 11.27850996657559790, 10.49999999999999822 ) ) ;
#33936=DIRECTION ( 'NONE',  ( 0.5877852522924796874, 0.8090169943749426773, 0.000000000000000000 ) ) ;
#33939=CARTESIAN_POINT ( 'NONE',  ( 14.97009266215792778, 21.42933399866928568, 7.000000000000000000 ) ) ;
#33940=AXIS2_PLACEMENT_3D ( 'NONE', #23714, #24112, #36113 ) ;
#33941=ORIENTED_EDGE ( 'NONE', *, *, #27498, .F. ) ;
#33943=ORIENTED_EDGE ( 'NONE', *, *, #18917, .F. ) ;
#33949=CARTESIAN_POINT ( 'NONE',  ( 4.984135866956514782, 36.15314577889351000, 10.49999999999999467 ) ) ;
#33953=AXIS2_PLACEMENT_3D ( 'NONE', #19366, #28510, #38055 ) ;
#33954=DIRECTION ( 'NONE',  ( -0.4067366430758009299, -0.9135454576426005335, 0.000000000000000000 ) ) ;
#33955=CARTESIAN_POINT ( 'NONE',  ( -6.811226782241547539, 35.33967249274200384, 7.500000000000000888 ) ) ;
#33957=VECTOR ( 'NONE', #13801, 1000.000000000000000 ) ;
#33958=PLANE ( 'NONE',  #34761 ) ;
#33961=DIRECTION ( 'NONE',  ( 0.1045284632676415082, -0.9945218953682745111, 0.000000000000000000 ) ) ;
#33963=EDGE_CURVE ( 'NONE', #21146, #11250, #13349, .T. ) ;
#33964=AXIS2_PLACEMENT_3D ( 'NONE', #23465, #29958, #21021 ) ;
#33965=ORIENTED_EDGE ( 'NONE', *, *, #33717, .F. ) ;
#33971=DIRECTION ( 'NONE',  ( 1.000000000000000000, 0.000000000000000000, 0.000000000000000000 ) ) ;
#33973=ORIENTED_EDGE ( 'NONE', *, *, #450, .T. ) ;
#33976=DIRECTION ( 'NONE',  ( -0.7032331762534065334, 0.07391278520356939219, -0.7071067811865449082 ) ) ;
#33983=VERTEX_POINT ( 'NONE', #12219 ) ;
#33985=CARTESIAN_POINT ( 'NONE',  ( 9.331903152615748098, 11.35703883385568780, 10.49999999999999645 ) ) ;
#33986=DIRECTION ( 'NONE',  ( 0.000000000000000000, 0.000000000000000000, -1.000000000000000000 ) ) ;
#33987=EDGE_LOOP ( 'NONE', ( #7192, #17538, #36361, #8557 ) ) ;
#33989=EDGE_LOOP ( 'NONE', ( #11433, #36961, #37330, #22224 ) ) ;
#33992=VECTOR ( 'NONE', #21305, 1000.000000000000114 ) ;
#33995=VERTEX_POINT ( 'NONE', #27857 ) ;
#33997=EDGE_CURVE ( 'NONE', #4123, #6233, #7085, .T. ) ;
#33998=CARTESIAN_POINT ( 'NONE',  ( -5.982165713378357452, 28.55918256678905465, 9.000000000000001776 ) ) ;
#33999=EDGE_CURVE ( 'NONE', #4629, #22450, #34703, .T. ) ;
#34000=CARTESIAN_POINT ( 'NONE',  ( -1.000000000000000000, 37.00000000000000711, 7.500000000000000888 ) ) ;
#34003=B_SPLINE_SURFACE_WITH_KNOTS ( 'NONE', 1, 3, ( 
 ( #28558, #37899, #17336, #10073, #29711, #7009, #32976, #28353, #533, #23217 ),
 ( #12917, #9871, #30116, #8778, #39251, #8383, #27066, #24616, #26862, #11432 ) ),
 .UNSPECIFIED., .F., .F., .F.,
 ( 2, 2 ),
 ( 4, 2, 2, 2, 4 ),
 ( 0.000000000000000000, 1.000000000000000000 ),
 ( 4.563205465131974670, 4.955904546830696589, 5.348603628529417620, 5.741302710228138650, 6.134001791926860570 ),
 .UNSPECIFIED. ) ;
#34006=AXIS2_PLACEMENT_3D ( 'NONE', #5568, #29555, #5371 ) ;
#34010=DIRECTION ( 'NONE',  ( -0.7431448254773961315, -0.6691306063588561281, 0.000000000000000000 ) ) ;
#34011=DIRECTION ( 'NONE',  ( -0.000000000000000000, -0.000000000000000000, -1.000000000000000000 ) ) ;
#34014=EDGE_CURVE ( 'NONE', #9003, #39013, #12415, .T. ) ;
#34019=ADVANCED_FACE ( 'NONE', ( #31853 ), #2982, .T. ) ;
#34026=CARTESIAN_POINT ( 'NONE',  ( 13.30736791475921699, 15.68301270237638967, 10.49999999999999822 ) ) ;
#34037=DIRECTION ( 'NONE',  ( 0.9510565162951544194, 0.3090169943749450643, 0.000000000000000000 ) ) ;
#34038=CARTESIAN_POINT ( 'NONE',  ( -13.24038105676664401, 15.43301270189234486, 10.49999999999999822 ) ) ;
#34040=ORIENTED_EDGE ( 'NONE', *, *, #7128, .F. ) ;
#34045=ORIENTED_EDGE ( 'NONE', *, *, #29264, .T. ) ;
#34047=CARTESIAN_POINT ( 'NONE',  ( 0.6666666666666681840, 37.00000000000000711, 10.83333333333333215 ) ) ;
#34048=VECTOR ( 'NONE', #915, 1000.000000000000114 ) ;
#34049=ORIENTED_EDGE ( 'NONE', *, *, #32821, .F. ) ;
#34050=EDGE_CURVE ( 'NONE', #30652, #21181, #35104, .T. ) ;
#34051=DIRECTION ( 'NONE',  ( -0.3090169943749465631, 0.9510565162951538642, 0.000000000000000000 ) ) ;
#34052=FACE_OUTER_BOUND ( 'NONE', #2938, .T. ) ;
#34056=CARTESIAN_POINT ( 'NONE',  ( 14.46041492111391236, 20.47739500831021076, 10.99387789255783687 ) ) ;
#34057=DIRECTION ( 'NONE',  ( 0.000000000000000000, 0.000000000000000000, -1.000000000000000000 ) ) ;
#34059=CARTESIAN_POINT ( 'NONE',  ( -8.007761790012255076, 9.776959832083379709, 10.50000000000000000 ) ) ;
#34063=DIRECTION ( 'NONE',  ( 0.4999999999999930056, -0.8660254037844428154, 0.000000000000000000 ) ) ;
#34064=VERTEX_POINT ( 'NONE', #21559 ) ;
#34066=CARTESIAN_POINT ( 'NONE',  ( 12.14070168820766149, 14.52831216351291133, 10.66666666666666430 ) ) ;
#34072=ORIENTED_EDGE ( 'NONE', *, *, #14187, .T. ) ;
#34073=AXIS2_PLACEMENT_3D ( 'NONE', #24910, #10070, #27956 ) ;
#34074=CARTESIAN_POINT ( 'NONE',  ( -3.992867117591420545, 8.524771480177605554, 10.50000000000000533 ) ) ;
#34082=DIRECTION ( 'NONE',  ( -0.000000000000000000, -0.000000000000000000, -1.000000000000000000 ) ) ;
#34083=EDGE_CURVE ( 'NONE', #25600, #19954, #23099, .T. ) ;
#34085=ORIENTED_EDGE ( 'NONE', *, *, #28381, .T. ) ;
#34089=DIRECTION ( 'NONE',  ( 1.000000000000000000, 0.000000000000000000, 0.000000000000000000 ) ) ;
#34090=CARTESIAN_POINT ( 'NONE',  ( 5.167086843766644400, 44.40436517110171621, 11.00000000000000000 ) ) ;
#34093=VECTOR ( 'NONE', #33139, 1000.000000000000000 ) ;
#34094=EDGE_CURVE ( 'NONE', #28626, #26207, #38005, .T. ) ;
#34095=ORIENTED_EDGE ( 'NONE', *, *, #3274, .F. ) ;
#34096=CYLINDRICAL_SURFACE ( 'NONE', #6397, 6.000000000000008882 ) ;
#34098=DIRECTION ( 'NONE',  ( -1.000000000000000000, 0.000000000000000000, 0.000000000000000000 ) ) ;
#34099=CIRCLE ( 'NONE', #37977, 15.00000000000000000 ) ;
#34100=CARTESIAN_POINT ( 'NONE',  ( -2.525645716490710679, 8.212903943950959018, 7.000000000000000000 ) ) ;
#34102=AXIS2_PLACEMENT_3D ( 'NONE', #27625, #2058, #12386 ) ;
#34104=ORIENTED_EDGE ( 'NONE', *, *, #34105, .T. ) ;
#34105=EDGE_CURVE ( 'NONE', #31246, #33136, #4222, .T. ) ;
#34109=EDGE_CURVE ( 'NONE', #37387, #21382, #26327, .T. ) ;
#34114=ORIENTED_EDGE ( 'NONE', *, *, #17474, .F. ) ;
#34120=DIRECTION ( 'NONE',  ( -0.9781476007338042455, 0.2079116908177663647, -0.000000000000000000 ) ) ;
#34124=EDGE_CURVE ( 'NONE', #3294, #6531, #31655, .T. ) ;
#34126=CARTESIAN_POINT ( 'NONE',  ( 11.11016527260166953, 31.83082137946472656, 11.00000000000000000 ) ) ;
#34127=ADVANCED_FACE ( 'NONE', ( #21365 ), #24806, .T. ) ;
#34133=AXIS2_PLACEMENT_3D ( 'NONE', #30910, #4015, #28805 ) ;
#34134=AXIS2_PLACEMENT_3D ( 'NONE', #21475, #24720, #27573 ) ;
#34135=CARTESIAN_POINT ( 'NONE',  ( -9.126688212161006675, 10.78884215935646829, 10.87262190629280134 ) ) ;
#34136=ORIENTED_EDGE ( 'NONE', *, *, #37633, .F. ) ;
#34139=AXIS2_PLACEMENT_3D ( 'NONE', #19260, #13161, #25554 ) ;
#34141=ORIENTED_EDGE ( 'NONE', *, *, #11500, .F. ) ;
#34143=CARTESIAN_POINT ( 'NONE',  ( 12.19134295108989718, 16.61602540378438775, 10.50000000000000000 ) ) ;
#34146=EDGE_LOOP ( 'NONE', ( #13241, #8704, #32851 ) ) ;
#34149=CARTESIAN_POINT ( 'NONE',  ( 0.5000000000000012212, 31.00000000000000355, 7.000000000000000000 ) ) ;
#34150=ADVANCED_FACE ( 'NONE', ( #9173 ), #33958, .F. ) ;
#34152=CARTESIAN_POINT ( 'NONE',  ( 2.525645716490518833, 8.212903943950921715, 7.000000000000000000 ) ) ;
#34153=EDGE_LOOP ( 'NONE', ( #36436, #6675, #2479, #17359 ) ) ;
#34154=CARTESIAN_POINT ( 'NONE',  ( 1.872892888448897120, -2.256054360071899634, 7.000000000000000000 ) ) ;
#34156=CARTESIAN_POINT ( 'NONE',  ( 6.151085731882510288, 35.08626808545850650, 7.500000000000000000 ) ) ;
#34158=AXIS2_PLACEMENT_3D ( 'NONE', #11984, #27619, #11591 ) ;
#34159=CARTESIAN_POINT ( 'NONE',  ( 12.74038105676654453, 14.56698729810772264, 10.49999999999999822 ) ) ;
#34161=AXIS2_PLACEMENT_3D ( 'NONE', #21621, #18780, #31366 ) ;
#34166=VERTEX_POINT ( 'NONE', #12019 ) ;
#34171=EDGE_CURVE ( 'NONE', #751, #28389, #5919, .T. ) ;
#34172=VERTEX_POINT ( 'NONE', #2877 ) ;
#34180=FACE_OUTER_BOUND ( 'NONE', #32412, .T. ) ;
#34183=CARTESIAN_POINT ( 'NONE',  ( 10.44103466624280507, 32.57396620494213124, 9.500000000000000000 ) ) ;
#34184=DIRECTION ( 'NONE',  ( 0.000000000000000000, 0.000000000000000000, -1.000000000000000000 ) ) ;
#34185=ORIENTED_EDGE ( 'NONE', *, *, #15871, .F. ) ;
#34190=AXIS2_PLACEMENT_3D ( 'NONE', #36029, #8588, #8187 ) ;
#34195=LINE ( 'NONE', #12653, #3311 ) ;
#34197=CARTESIAN_POINT ( 'NONE',  ( 5.037377569032880587, 36.27272859966225127, 10.49999999999999645 ) ) ;
#34199=EDGE_CURVE ( 'NONE', #34486, #38096, #32874, .T. ) ;
#34201=ADVANCED_FACE ( 'NONE', ( #23717 ), #32471, .T. ) ;
#34202=DIRECTION ( 'NONE',  ( 1.000000000000000000, 0.000000000000000000, 0.000000000000000000 ) ) ;
#34206=DIRECTION ( 'NONE',  ( 0.6691306063588670083, 0.7431448254773863615, -0.000000000000000000 ) ) ;
#34208=DIRECTION ( 'NONE',  ( -0.000000000000000000, -0.000000000000000000, -1.000000000000000000 ) ) ;
#34210=VECTOR ( 'NONE', #23186, 1000.000000000000000 ) ;
#34211=ORIENTED_EDGE ( 'NONE', *, *, #33333, .F. ) ;
#34213=CIRCLE ( 'NONE', #1773, 1.000000000000014655 ) ;
#34219=ADVANCED_FACE ( 'NONE', ( #8276 ), #29812, .T. ) ;
#34220=ORIENTED_EDGE ( 'NONE', *, *, #14977, .T. ) ;
#34225=CARTESIAN_POINT ( 'NONE',  ( 12.38757880222261143, 14.77067777473940069, 10.99387789255784220 ) ) ;
#34226=EDGE_CURVE ( 'NONE', #38194, #9581, #7521, .T. ) ;
#34230=CARTESIAN_POINT ( 'NONE',  ( -25.19768531712390569, 23.50223830518991619, 7.000000000000000000 ) ) ;
#34232=VERTEX_POINT ( 'NONE', #23111 ) ;
#34234=FACE_OUTER_BOUND ( 'NONE', #2672, .T. ) ;
#34235=CARTESIAN_POINT ( 'NONE',  ( -2.629601561899595374, 7.723830143584053509, 7.000000000000000000 ) ) ;
#34236=CARTESIAN_POINT ( 'NONE',  ( -3.888911272182536294, 9.013845280544513727, 10.50000000000000000 ) ) ;
#34237=EDGE_LOOP ( 'NONE', ( #9408, #18264, #19299, #27097 ) ) ;
#34244=EDGE_CURVE ( 'NONE', #23135, #10104, #14668, .T. ) ;
#34245=CARTESIAN_POINT ( 'NONE',  ( 0.8333333333333349247, 37.00000000000000711, 10.66666666666666607 ) ) ;
#34246=VECTOR ( 'NONE', #25186, 999.9999999999998863 ) ;
#34247=CONICAL_SURFACE ( 'NONE', #20619, 1.000000000000004441, 0.7853981633974482790 ) ;
#34249=ORIENTED_EDGE ( 'NONE', *, *, #12218, .T. ) ;
#34251=TOROIDAL_SURFACE ( 'NONE', #16737, 1.000000000000000000, 0.5000000000000000000 ) ;
#34253=CYLINDRICAL_SURFACE ( 'NONE', #9744, 0.5000000000000000000 ) ;
#34254=CARTESIAN_POINT ( 'NONE',  ( 7.530592408760857559, 11.28437794979193498, 9.500000000000000000 ) ) ;
#34256=CARTESIAN_POINT ( 'NONE',  ( -3.295881626406750975, 9.398963235502533209, 7.000000000000000000 ) ) ;
#34257=CARTESIAN_POINT ( 'NONE',  ( 14.72308455763283064, 20.12562289931477366, 10.49999999999999822 ) ) ;
#34258=DIRECTION ( 'NONE',  ( 1.000000000000000000, 0.000000000000000000, 0.000000000000000000 ) ) ;
#34263=PLANE ( 'NONE',  #17849 ) ;
#34264=VERTEX_POINT ( 'NONE', #5028 ) ;
#34267=DIRECTION ( 'NONE',  ( 1.000000000000000000, 0.000000000000000000, -0.000000000000000000 ) ) ;
#34277=VECTOR ( 'NONE', #30546, 999.9999999999998863 ) ;
#34283=AXIS2_PLACEMENT_3D ( 'NONE', #4152, #13496, #32196 ) ;
#34284=VERTEX_POINT ( 'NONE', #1585 ) ;
#34288=VERTEX_POINT ( 'NONE', #10519 ) ;
#34290=DIRECTION ( 'NONE',  ( -0.6916548014802208488, 0.1470157664652026186, -0.7071067811865512365 ) ) ;
#34294=ORIENTED_EDGE ( 'NONE', *, *, #34447, .T. ) ;
#34295=CARTESIAN_POINT ( 'NONE',  ( -15.02235689379176620, 21.92659494635362449, 11.00000000000000000 ) ) ;
#34297=CARTESIAN_POINT ( 'NONE',  ( 7.713869163865849643, 10.18146832927074996, 10.49999999999999822 ) ) ;
#34298=CARTESIAN_POINT ( 'NONE',  ( 12.99038105676654986, 14.99999999999993960, 7.000000000000000000 ) ) ;
#34300=AXIS2_PLACEMENT_3D ( 'NONE', #14649, #29683, #23185 ) ;
#34301=DIRECTION ( 'NONE',  ( -0.4067366430757888840, 0.9135454576426058626, 0.000000000000000000 ) ) ;
#34304=FACE_OUTER_BOUND ( 'NONE', #32935, .T. ) ;
#34305=DIRECTION ( 'NONE',  ( -0.000000000000000000, -0.000000000000000000, -1.000000000000000000 ) ) ;
#34306=CONICAL_SURFACE ( 'NONE', #576, 1.000000000000002665, 0.7853981633974548293 ) ;
#34307=DIRECTION ( 'NONE',  ( -0.000000000000000000, -0.000000000000000000, 1.000000000000000000 ) ) ;
#34308=LINE ( 'NONE', #39644, #10655 ) ;
#34311=ORIENTED_EDGE ( 'NONE', *, *, #14235, .T. ) ;
#34315=DIRECTION ( 'NONE',  ( 1.000000000000000000, 0.000000000000000000, -0.000000000000000000 ) ) ;
#34324=ADVANCED_FACE ( 'NONE', ( #11129 ), #39150, .F. ) ;
#34325=CARTESIAN_POINT ( 'NONE',  ( 5.478580155932369244, 36.03438916679310466, 10.99387789255784043 ) ) ;
#34326=EDGE_LOOP ( 'NONE', ( #26663, #3952, #7330, #22422 ) ) ;
#34328=DIRECTION ( 'NONE',  ( -0.000000000000000000, -0.000000000000000000, 1.000000000000000000 ) ) ;
#34329=LINE ( 'NONE', #9550, #12693 ) ;
#34332=FACE_OUTER_BOUND ( 'NONE', #31320, .T. ) ;
#34333=ORIENTED_EDGE ( 'NONE', *, *, #12904, .F. ) ;
#34336=CARTESIAN_POINT ( 'NONE',  ( 14.48316745233715075, 26.40420323494709365, 7.455539900862802050 ) ) ;
#34337=FACE_OUTER_BOUND ( 'NONE', #29998, .T. ) ;
#34338=ADVANCED_FACE ( 'NONE', ( #16829 ), #32189, .T. ) ;
#34340=B_SPLINE_SURFACE_WITH_KNOTS ( 'NONE', 1, 3, ( 
 ( #29510, #2089, #1686, #14469, #29311, #26861, #13869, #36015, #23418, #35810 ),
 ( #7965, #11227, #8174, #20578, #17536, #39250, #30718, #27262, #11823, #36609 ) ),
 .UNSPECIFIED., .F., .F., .F.,
 ( 2, 2 ),
 ( 4, 2, 2, 2, 4 ),
 ( 0.000000000000000000, 1.000000000000000000 ),
 ( 4.324792293729522896, 4.717491375428245703, 5.110190457126968511, 5.502889538825691318, 5.895588620524415013 ),
 .UNSPECIFIED. ) ;
#34341=VERTEX_POINT ( 'NONE', #1381 ) ;
#34343=DIRECTION ( 'NONE',  ( 0.000000000000000000, 0.000000000000000000, -1.000000000000000000 ) ) ;
#34346=ORIENTED_EDGE ( 'NONE', *, *, #35727, .T. ) ;
#34348=CARTESIAN_POINT ( 'NONE',  ( -7.713869163866016621, 10.18146832927085121, 7.000000000000000000 ) ) ;
#34349=CARTESIAN_POINT ( 'NONE',  ( 2.036571916123615100, 8.108948098542045457, 11.00000000000000000 ) ) ;
#34351=DIRECTION ( 'NONE',  ( 0.1470157664652248786, 0.6916548014802228472, -0.7071067811865445751 ) ) ;
#34352=EDGE_LOOP ( 'NONE', ( #18291, #9386, #15132, #39897 ) ) ;
#34353=LINE ( 'NONE', #9167, #6672 ) ;
#34355=EDGE_CURVE ( 'NONE', #10259, #2141, #34647, .T. ) ;
#34356=CARTESIAN_POINT ( 'NONE',  ( 12.23327497914553597, 13.81973598992451713, 7.000000000000000000 ) ) ;
#34357=EDGE_CURVE ( 'NONE', #20669, #26489, #26361, .T. ) ;
#34358=DIRECTION ( 'NONE',  ( -1.000000000000000000, 0.000000000000000000, 0.000000000000000000 ) ) ;
#34361=CIRCLE ( 'NONE', #3870, 0.5000000000000004441 ) ;
#34363=CARTESIAN_POINT ( 'NONE',  ( 8.169448529985288587, 9.961039561530309783, 10.49999999999999822 ) ) ;
#34364=CIRCLE ( 'NONE', #16859, 0.4999999999999998335 ) ;
#34365=DIRECTION ( 'NONE',  ( -0.000000000000000000, -0.000000000000000000, -1.000000000000000000 ) ) ;
#34375=EDGE_CURVE ( 'NONE', #31487, #1365, #37374, .T. ) ;
#34383=DIRECTION ( 'NONE',  ( 0.000000000000000000, -0.000000000000000000, 1.000000000000000000 ) ) ;
#34384=LINE ( 'NONE', #12644, #19949 ) ;
#34385=ORIENTED_EDGE ( 'NONE', *, *, #16962, .T. ) ;
#34387=VERTEX_POINT ( 'NONE', #33677 ) ;
#34394=LINE ( 'NONE', #25240, #17612 ) ;
#34396=LINE ( 'NONE', #34792, #15514 ) ;
#34397=EDGE_CURVE ( 'NONE', #16754, #2909, #35438, .T. ) ;
#34398=LINE ( 'NONE', #12853, #24688 ) ;
#34400=AXIS2_PLACEMENT_3D ( 'NONE', #2424, #39787, #8918 ) ;
#34405=DIRECTION ( 'NONE',  ( 1.000000000000000000, 0.000000000000000000, 0.000000000000000000 ) ) ;
#34407=DIRECTION ( 'NONE',  ( 0.8090169943749430104, -0.5877852522924791323, 0.000000000000000000 ) ) ;
#34409=ORIENTED_EDGE ( 'NONE', *, *, #37932, .T. ) ;
#34412=DIRECTION ( 'NONE',  ( 0.1470157664652028962, 0.6916548014802217370, 0.7071067811865503483 ) ) ;
#34414=EDGE_LOOP ( 'NONE', ( #15836, #16034, #30698, #23241 ) ) ;
#34415=CARTESIAN_POINT ( 'NONE',  ( -5.767236651883567156, 13.71142893291686171, 10.50000000000000000 ) ) ;
#34416=VECTOR ( 'NONE', #26750, 999.9999999999998863 ) ;
#34417=ORIENTED_EDGE ( 'NONE', *, *, #2689, .T. ) ;
#34419=CYLINDRICAL_SURFACE ( 'NONE', #10816, 0.4999999999999998335 ) ;
#34421=EDGE_CURVE ( 'NONE', #2164, #35202, #21464, .T. ) ;
#34423=ORIENTED_EDGE ( 'NONE', *, *, #36084, .F. ) ;
#34426=CYLINDRICAL_SURFACE ( 'NONE', #37782, 5.999999999999998224 ) ;
#34431=EDGE_CURVE ( 'NONE', #17047, #36571, #30426, .T. ) ;
#34432=CARTESIAN_POINT ( 'NONE',  ( -9.201548168576545450, 26.54122646004472585, 10.50000000000000533 ) ) ;
#34439=AXIS2_PLACEMENT_3D ( 'NONE', #35299, #1782, #38546 ) ;
#34440=ORIENTED_EDGE ( 'NONE', *, *, #33825, .T. ) ;
#34442=LINE ( 'NONE', #28140, #12809 ) ;
#34443=EDGE_LOOP ( 'NONE', ( #20821, #14188, #17471, #27916, #31330, #18539, #1732, #34509, #18906, #949, #24830, #26762, #1321, #21585, #13882, #8602, #28058, #2226, #22702, #37789, #2029, #17965, #14888, #7387, #39750, #2230, #11101, #37658, #10811, #13333, #30289, #39377, #35826, #7530, #13206, #6129, #30496, #965, #19310, #2467, #18460, #40089, #1661, #2889, #3215, #10203, #15249, #25797, #416, #16046, #9646, #23294, #13477, #28774, #29295 ) ) ;
#34446=EDGE_CURVE ( 'NONE', #15350, #22657, #38684, .T. ) ;
#34447=EDGE_CURVE ( 'NONE', #16160, #16754, #33480, .T. ) ;
#34449=CARTESIAN_POINT ( 'NONE',  ( -14.97277451176450924, 21.48159783397892397, 10.49999999999999822 ) ) ;
#34451=CARTESIAN_POINT ( 'NONE',  ( -13.53280532430055416, 27.77329351534951485, 10.66666666666666963 ) ) ;
#34452=LINE ( 'NONE', #12705, #14344 ) ;
#34453=LINE ( 'NONE', #19401, #9067 ) ;
#34454=DIRECTION ( 'NONE',  ( 0.9135454576426005335, -0.4067366430758009299, 0.000000000000000000 ) ) ;
#34455=DIRECTION ( 'NONE',  ( -0.6691306063588571273, 0.7431448254773952433, 0.000000000000000000 ) ) ;
#34458=PLANE ( 'NONE',  #34698 ) ;
#34459=ORIENTED_EDGE ( 'NONE', *, *, #23651, .F. ) ;
#34460=CONICAL_SURFACE ( 'NONE', #35771, 1.000000000000016431, 0.7853981633974533860 ) ;
#34463=CARTESIAN_POINT ( 'NONE',  ( -10.10646936306323518, 32.94553861768095970, 11.00000000000000000 ) ) ;
#34464=VECTOR ( 'NONE', #11617, 1000.000000000000000 ) ;
#34469=ORIENTED_EDGE ( 'NONE', *, *, #21090, .T. ) ;
#34477=ORIENTED_EDGE ( 'NONE', *, *, #6067, .F. ) ;
#34482=EDGE_LOOP ( 'NONE', ( #29537, #33380, #4331 ) ) ;
#34484=EDGE_CURVE ( 'NONE', #8314, #11507, #8682, .T. ) ;
#34486=VERTEX_POINT ( 'NONE', #30620 ) ;
#34487=CARTESIAN_POINT ( 'NONE',  ( 14.36830325120613594, 20.48707633493483371, 11.00000000000000000 ) ) ;
#34488=LINE ( 'NONE', #32241, #31028 ) ;
#34493=AXIS2_PLACEMENT_3D ( 'NONE', #9763, #37192, #21743 ) ;
#34496=VERTEX_POINT ( 'NONE', #11729 ) ;
#34497=LINE ( 'NONE', #9316, #19712 ) ;
#34498=EDGE_CURVE ( 'NONE', #34284, #29758, #15883, .T. ) ;
#34500=DIRECTION ( 'NONE',  ( 1.000000000000000000, 0.000000000000000000, 0.000000000000000000 ) ) ;
#34501=ORIENTED_EDGE ( 'NONE', *, *, #14597, .F. ) ;
#34503=LINE ( 'NONE', #37551, #3557 ) ;
#34504=CARTESIAN_POINT ( 'NONE',  ( -5.440908595777639079, 35.94977745735568675, 11.00000000000000000 ) ) ;
#34507=CARTESIAN_POINT ( 'NONE',  ( -2.140527761532693418, 7.619874298175171035, 7.000000000000000000 ) ) ;
#34509=ORIENTED_EDGE ( 'NONE', *, *, #3566, .F. ) ;
#34516=FACE_OUTER_BOUND ( 'NONE', #1954, .T. ) ;
#34523=CARTESIAN_POINT ( 'NONE',  ( 8.145563986382251542, 10.43794218875012270, 11.00000000000000000 ) ) ;
#34524=CARTESIAN_POINT ( 'NONE',  ( 5.558911028763954931, 36.44455752850700492, 10.49999999999999822 ) ) ;
#34528=CARTESIAN_POINT ( 'NONE',  ( -12.30736835487442704, 14.81698729810789672, 7.000000000000000000 ) ) ;
#34529=ORIENTED_EDGE ( 'NONE', *, *, #27200, .T. ) ;
#34533=DIRECTION ( 'NONE',  ( 0.6729908358753983189, 0.000000000000000000, -0.7396508195275205422 ) ) ;
#34534=ORIENTED_EDGE ( 'NONE', *, *, #27851, .F. ) ;
#34536=LINE ( 'NONE', #35136, #22856 ) ;
#34537=ORIENTED_EDGE ( 'NONE', *, *, #30104, .F. ) ;
#34540=VERTEX_POINT ( 'NONE', #27562 ) ;
#34545=DIRECTION ( 'NONE',  ( -0.000000000000000000, -0.000000000000000000, -1.000000000000000000 ) ) ;
#34546=EDGE_LOOP ( 'NONE', ( #4372, #3901, #26145, #20553 ) ) ;
#34547=VECTOR ( 'NONE', #33820, 1000.000000000000000 ) ;
#34548=CARTESIAN_POINT ( 'NONE',  ( 4.002483478063409095, 8.479530061156575371, 10.49999999999999822 ) ) ;
#34551=EDGE_CURVE ( 'NONE', #39411, #39304, #36715, .T. ) ;
#34552=CARTESIAN_POINT ( 'NONE',  ( 7.530592408760857559, 11.28437794979193498, 9.500000000000000000 ) ) ;
#34555=VECTOR ( 'NONE', #37184, 1000.000000000000114 ) ;
#34556=EDGE_CURVE ( 'NONE', #17440, #20104, #10699, .T. ) ;
#34558=CARTESIAN_POINT ( 'NONE',  ( 5.187504188494417079, 36.60991850771481637, 7.000000000000000000 ) ) ;
#34559=DIRECTION ( 'NONE',  ( 0.8090169943749497827, 0.5877852522924698064, 0.000000000000000000 ) ) ;
#34567=ORIENTED_EDGE ( 'NONE', *, *, #31491, .F. ) ;
#34569=CARTESIAN_POINT ( 'NONE',  ( -6.557822374958138134, 35.99981354310120452, 10.49999999999999822 ) ) ;
#34573=VECTOR ( 'NONE', #33572, 1000.000000000000000 ) ;
#34574=LINE ( 'NONE', #26021, #28728 ) ;
#34578=CARTESIAN_POINT ( 'NONE',  ( 5.440908595777814050, 35.94977745735560859, 7.000000000000000000 ) ) ;
#34579=EDGE_CURVE ( 'NONE', #24416, #38300, #38537, .T. ) ;
#34580=EDGE_LOOP ( 'NONE', ( #18803, #29429, #36147, #22429, #5652, #22369 ) ) ;
#34582=ORIENTED_EDGE ( 'NONE', *, *, #38667, .F. ) ;
#34584=CIRCLE ( 'NONE', #9303, 1.000000000000001110 ) ;
#34587=ORIENTED_EDGE ( 'NONE', *, *, #38286, .T. ) ;
#34588=LINE ( 'NONE', #19146, #33842 ) ;
#34591=ADVANCED_FACE ( 'NONE', ( #5432 ), #29509, .T. ) ;
#34592=DIRECTION ( 'NONE',  ( -0.5720614028176770338, 0.4156269377774552409, -0.7071067811865524577 ) ) ;
#34594=CARTESIAN_POINT ( 'NONE',  ( -11.48173768534023154, 32.16538668264431777, 10.49999999999999822 ) ) ;
#34596=EDGE_CURVE ( 'NONE', #17719, #4586, #31275, .T. ) ;
#34599=EDGE_CURVE ( 'NONE', #13849, #26235, #12631, .T. ) ;
#34607=STYLED_ITEM ( 'NONE', ( #13199 ), #36190 ) ;
#34614=DIRECTION ( 'NONE',  ( 1.000000000000000000, 0.000000000000000000, 0.000000000000000000 ) ) ;
#34617=EDGE_LOOP ( 'NONE', ( #39835, #26724, #8760, #13336 ) ) ;
#34624=CARTESIAN_POINT ( 'NONE',  ( -13.63581098909220479, 27.45627467658446008, 11.00000000000000000 ) ) ;
#34625=EDGE_CURVE ( 'NONE', #11714, #1404, #25701, .T. ) ;
#34627=ADVANCED_FACE ( 'NONE', ( #38095 ), #34458, .F. ) ;
#34629=ORIENTED_EDGE ( 'NONE', *, *, #957, .F. ) ;
#34637=CARTESIAN_POINT ( 'NONE',  ( 9.819582157326484761, 24.63911342745429778, 10.50000000000000533 ) ) ;
#34638=ORIENTED_EDGE ( 'NONE', *, *, #5247, .F. ) ;
#34639=DIRECTION ( 'NONE',  ( -0.9510565162951538642, -0.3090169943749466186, -0.000000000000000000 ) ) ;
#34640=EDGE_CURVE ( 'NONE', #25412, #29091, #8105, .T. ) ;
#34643=DIRECTION ( 'NONE',  ( -0.4067366430757884399, 0.9135454576426061957, 1.040834085586084414E-14 ) ) ;
#34646=CARTESIAN_POINT ( 'NONE',  ( 3.597409820281487480, 14.42008525284347087, 9.000000000000001776 ) ) ;
#34647=B_SPLINE_CURVE_WITH_KNOTS ( 'NONE', 3,
 ( #35912, #20075, #26155, #17029, #29409, #13969 ),
 .UNSPECIFIED., .F., .F.,
 ( 4, 2, 4 ),
 ( 0.000000000000000000, 0.5000000000000000000, 1.000000000000000000 ),
 .UNSPECIFIED. ) ;
#34649=CARTESIAN_POINT ( 'NONE',  ( 14.36830325120613594, 20.48707633493483371, 7.000000000000000000 ) ) ;
#34650=CARTESIAN_POINT ( 'NONE',  ( -8.505700342264141511, 22.10876900990917804, 9.000000000000001776 ) ) ;
#34651=CARTESIAN_POINT ( 'NONE',  ( -24.90379269097766368, 23.90674680237738770, 9.500000000000000000 ) ) ;
#34653=CARTESIAN_POINT ( 'NONE',  ( -6.972208014302417212, 35.78128242463058228, 7.339470489435489853 ) ) ;
#34654=ORIENTED_EDGE ( 'NONE', *, *, #28957, .T. ) ;
#34656=LINE ( 'NONE', #11228, #27194 ) ;
#34657=CIRCLE ( 'NONE', #32045, 0.5000000000000004441 ) ;
#34658=CARTESIAN_POINT ( 'NONE',  ( 13.30786737960926480, 15.60542992190359435, 10.49999999999999822 ) ) ;
#34660=DIRECTION ( 'NONE',  ( -1.000000000000000000, 0.000000000000000000, 0.000000000000000000 ) ) ;
#34662=ORIENTED_EDGE ( 'NONE', *, *, #6198, .T. ) ;
#34666=CARTESIAN_POINT ( 'NONE',  ( -8.339609403135950672, 11.87216320208450959, 10.00000000000000000 ) ) ;
#34677=ORIENTED_EDGE ( 'NONE', *, *, #3423, .F. ) ;
#34679=EDGE_CURVE ( 'NONE', #1586, #3451, #23690, .T. ) ;
#34682=ORIENTED_EDGE ( 'NONE', *, *, #26974, .T. ) ;
#34687=ORIENTED_EDGE ( 'NONE', *, *, #28780, .F. ) ;
#34689=FACE_OUTER_BOUND ( 'NONE', #36092, .T. ) ;
#34690=CARTESIAN_POINT ( 'NONE',  ( -0.8333333333333351467, 37.00000000000000711, 10.66666666666666607 ) ) ;
#34691=ADVANCED_FACE ( 'NONE', ( #13107 ), #129, .T. ) ;
#34693=ORIENTED_EDGE ( 'NONE', *, *, #34881, .T. ) ;
#34694=ADVANCED_FACE ( 'NONE', ( #18626 ), #34263, .T. ) ;
#34696=DIRECTION ( 'NONE',  ( 0.2079116908177532363, -0.9781476007338070211, 0.000000000000000000 ) ) ;
#34697=CARTESIAN_POINT ( 'NONE',  ( -12.30736835487442882, 14.81698729810789672, 7.000000000000000000 ) ) ;
#34698=AXIS2_PLACEMENT_3D ( 'NONE', #6606, #3573, #19209 ) ;
#34699=DIRECTION ( 'NONE',  ( 0.000000000000000000, 0.000000000000000000, 1.000000000000000000 ) ) ;
#34700=FACE_OUTER_BOUND ( 'NONE', #16989, .T. ) ;
#34703=LINE ( 'NONE', #6856, #21793 ) ;
#34705=ORIENTED_EDGE ( 'NONE', *, *, #24763, .F. ) ;
#34706=ADVANCED_FACE ( 'NONE', ( #35054 ), #31598, .T. ) ;
#34708=CARTESIAN_POINT ( 'NONE',  ( 7.419976537719617404, 10.58597682645822324, 10.50000000000000000 ) ) ;
#34709=DIRECTION ( 'NONE',  ( 1.000000000000000000, 0.000000000000000000, 0.000000000000000000 ) ) ;
#34711=DIRECTION ( 'NONE',  ( 0.3090169943749448977, -0.9510565162951543083, 0.000000000000000000 ) ) ;
#34714=CARTESIAN_POINT ( 'NONE',  ( 9.427394962683440127, 11.06314620782477753, 10.49999999999999822 ) ) ;
#34719=CARTESIAN_POINT ( 'NONE',  ( -13.36146265112639675, 15.68301270189280672, 7.445905703748357141 ) ) ;
#34720=CARTESIAN_POINT ( 'NONE',  ( 5.537830610278449583, 36.16746786612485920, 10.94387467463502439 ) ) ;
#34722=ORIENTED_EDGE ( 'NONE', *, *, #189, .T. ) ;
#34726=VECTOR ( 'NONE', #31265, 1000.000000000000114 ) ;
#34727=DIRECTION ( 'NONE',  ( -0.000000000000000000, -0.000000000000000000, -1.000000000000000000 ) ) ;
#34728=VERTEX_POINT ( 'NONE', #25307 ) ;
#34730=CARTESIAN_POINT ( 'NONE',  ( 6.354454053420411697, 35.54304081427980577, 11.00000000000000000 ) ) ;
#34732=B_SPLINE_CURVE_WITH_KNOTS ( 'NONE', 3,
 ( #22240, #21850, #9674, #3757, #16359, #15757 ),
 .UNSPECIFIED., .F., .F.,
 ( 4, 2, 4 ),
 ( 0.000000000000000000, 0.5000000000000000000, 1.000000000000000000 ),
 .UNSPECIFIED. ) ;
#34733=ORIENTED_EDGE ( 'NONE', *, *, #1611, .F. ) ;
#34736=ORIENTED_EDGE ( 'NONE', *, *, #25148, .F. ) ;
#34738=AXIS2_PLACEMENT_3D ( 'NONE', #33071, #39544, #30006 ) ;
#34739=AXIS2_PLACEMENT_3D ( 'NONE', #20937, #15036, #39616 ) ;
#34740=EDGE_LOOP ( 'NONE', ( #26440, #32947, #7017 ) ) ;
#34743=CARTESIAN_POINT ( 'NONE',  ( 6.677405195727081022, 35.94657184102473479, 10.49999999999999645 ) ) ;
#34744=EDGE_CURVE ( 'NONE', #16887, #15951, #8466, .T. ) ;
#34746=FACE_OUTER_BOUND ( 'NONE', #15525, .T. ) ;
#34749=DIRECTION ( 'NONE',  ( 1.000000000000000000, 0.000000000000000000, 0.000000000000000000 ) ) ;
#34751=CARTESIAN_POINT ( 'NONE',  ( 12.47908909340999273, 14.17675236482283907, 7.338691926023210854 ) ) ;
#34755=ORIENTED_EDGE ( 'NONE', *, *, #6937, .T. ) ;
#34759=DIRECTION ( 'NONE',  ( -1.000000000000000000, 0.000000000000000000, 0.000000000000000000 ) ) ;
#34760=ORIENTED_EDGE ( 'NONE', *, *, #4912, .F. ) ;
#34761=AXIS2_PLACEMENT_3D ( 'NONE', #19658, #6116, #981 ) ;
#34763=AXIS2_PLACEMENT_3D ( 'NONE', #11979, #27022, #23574 ) ;
#34766=CIRCLE ( 'NONE', #34139, 0.5000000000000004441 ) ;
#34769=VERTEX_POINT ( 'NONE', #15765 ) ;
#34778=CARTESIAN_POINT ( 'NONE',  ( 15.00000000000000000, 22.50000000000000711, 7.000000000000000000 ) ) ;
#34779=EDGE_CURVE ( 'NONE', #19849, #23702, #27572, .T. ) ;
#34782=ORIENTED_EDGE ( 'NONE', *, *, #17564, .T. ) ;
#34789=DIRECTION ( 'NONE',  ( -0.3090169943749448977, 0.9510565162951543083, 0.000000000000000000 ) ) ;
#34791=CIRCLE ( 'NONE', #3012, 1.000000000000007772 ) ;
#34792=CARTESIAN_POINT ( 'NONE',  ( -13.53057405073934838, 22.08338764125508291, 10.00000000000000000 ) ) ;
#34793=VECTOR ( 'NONE', #22705, 1000.000000000000000 ) ;
#34794=CARTESIAN_POINT ( 'NONE',  ( 13.62967667376826419, 40.40898974728997217, 11.00000000000000000 ) ) ;
#34804=CARTESIAN_POINT ( 'NONE',  ( 10.69300419909370525, 32.80084059136112984, 10.87262190629272318 ) ) ;
#34806=ORIENTED_EDGE ( 'NONE', *, *, #26846, .T. ) ;
#34808=PLANE ( 'NONE',  #21593 ) ;
#34811=CARTESIAN_POINT ( 'NONE',  ( -9.608347198026816471, 2.148595524579384186, 11.00000000000000000 ) ) ;
#34813=CARTESIAN_POINT ( 'NONE',  ( 12.64565515434632559, 14.62167732336930648, 10.82238861112336892 ) ) ;
#34815=AXIS2_PLACEMENT_3D ( 'NONE', #1292, #28712, #12874 ) ;
#34816=VERTEX_POINT ( 'NONE', #22060 ) ;
#34819=CARTESIAN_POINT ( 'NONE',  ( 8.927394655428274817, 11.06314620770945290, 11.00000000000000000 ) ) ;
#34824=CARTESIAN_POINT ( 'NONE',  ( 13.28401428810676066, 15.50858767547181394, 10.49999999999999822 ) ) ;
#34825=CARTESIAN_POINT ( 'NONE',  ( 3.992867117591230919, 8.524771480177550487, 7.000000000000000000 ) ) ;
#34826=CARTESIAN_POINT ( 'NONE',  ( -10.10646936306323518, 32.94553861768095970, 10.49999999999999822 ) ) ;
#34828=VERTEX_POINT ( 'NONE', #29160 ) ;
#34831=ADVANCED_FACE ( 'NONE', ( #4981 ), #4371, .F. ) ;
#34834=EDGE_LOOP ( 'NONE', ( #20804, #26568, #9110, #27227 ) ) ;
#34835=ADVANCED_FACE ( 'NONE', ( #14120 ), #13941, .T. ) ;
#34837=CARTESIAN_POINT ( 'NONE',  ( -14.47283171447380035, 21.48159823030330884, 11.00000000000000000 ) ) ;
#34838=VERTEX_POINT ( 'NONE', #35860 ) ;
#34839=LINE ( 'NONE', #2277, #22340 ) ;
#34840=VECTOR ( 'NONE', #15689, 1000.000000000000114 ) ;
#34841=VECTOR ( 'NONE', #31228, 1000.000000000000000 ) ;
#34842=CARTESIAN_POINT ( 'NONE',  ( -11.47910261372038399, 31.49019768869758806, 10.49999999999999822 ) ) ;
#34846=VERTEX_POINT ( 'NONE', #32003 ) ;
#34848=CARTESIAN_POINT ( 'NONE',  ( -6.807850151676340111, 35.76876263333496553, 10.49999999999999822 ) ) ;
#34849=EDGE_CURVE ( 'NONE', #172, #25521, #7208, .T. ) ;
#34850=CARTESIAN_POINT ( 'NONE',  ( 10.49474413300069386, 21.89971208337373554, 10.50000000000000000 ) ) ;
#34852=AXIS2_PLACEMENT_3D ( 'NONE', #24938, #3601, #37331 ) ;
#34853=PLANE ( 'NONE',  #10857 ) ;
#34854=DIRECTION ( 'NONE',  ( -0.6691306063588671194, -0.7431448254773862505, 0.000000000000000000 ) ) ;
#34855=LINE ( 'NONE', #7004, #10660 ) ;
#34857=VECTOR ( 'NONE', #18622, 1000.000000000000000 ) ;
#34859=ORIENTED_EDGE ( 'NONE', *, *, #10015, .T. ) ;
#34868=ORIENTED_EDGE ( 'NONE', *, *, #22527, .T. ) ;
#34869=CARTESIAN_POINT ( 'NONE',  ( 14.30862178846744825, 26.15670448022654782, 10.49999999999999822 ) ) ;
#34879=EDGE_LOOP ( 'NONE', ( #23338, #20602, #36143, #20639 ) ) ;
#34881=EDGE_CURVE ( 'NONE', #18776, #11714, #20023, .T. ) ;
#34884=ORIENTED_EDGE ( 'NONE', *, *, #36199, .F. ) ;
#34885=DIRECTION ( 'NONE',  ( -0.000000000000000000, -0.000000000000000000, -1.000000000000000000 ) ) ;
#34886=DIRECTION ( 'NONE',  ( -0.000000000000000000, -0.000000000000000000, -1.000000000000000000 ) ) ;
#34887=CIRCLE ( 'NONE', #25136, 6.000000000000000000 ) ;
#34890=CIRCLE ( 'NONE', #23203, 6.000000000000000000 ) ;
#34891=EDGE_LOOP ( 'NONE', ( #10402, #15071, #1280, #31977 ) ) ;
#34895=FACE_OUTER_BOUND ( 'NONE', #14606, .T. ) ;
#34896=ORIENTED_EDGE ( 'NONE', *, *, #29113, .T. ) ;
#34898=CARTESIAN_POINT ( 'NONE',  ( -13.96115708084650464, 27.98552962950150302, 7.381627713044564665 ) ) ;
#34899=PLANE ( 'NONE',  #4000 ) ;
#34901=VECTOR ( 'NONE', #9580, 1000.000000000000227 ) ;
#34903=CARTESIAN_POINT ( 'NONE',  ( -13.94482798346716201, 26.50521816028930644, 9.000000000000001776 ) ) ;
#34904=CARTESIAN_POINT ( 'NONE',  ( -3.503793317224518145, 8.420815634768723967, 7.499999999999997335 ) ) ;
#34905=VECTOR ( 'NONE', #25377, 1000.000000000000114 ) ;
#34907=DIRECTION ( 'NONE',  ( 1.000000000000000000, 0.000000000000000000, 0.000000000000000000 ) ) ;
#34909=ORIENTED_EDGE ( 'NONE', *, *, #24863, .F. ) ;
#34912=CARTESIAN_POINT ( 'NONE',  ( 3.357189294653307954, 32.49896394832310165, 10.50000000000000000 ) ) ;
#34914=CARTESIAN_POINT ( 'NONE',  ( 3.057264508911339274, 12.92643568347968674, 10.49999999999999467 ) ) ;
#34916=VECTOR ( 'NONE', #29944, 1000.000000000000000 ) ;
#34918=DIRECTION ( 'NONE',  ( -0.000000000000000000, 1.000000000000000000, -0.000000000000000000 ) ) ;
#34919=AXIS2_PLACEMENT_3D ( 'NONE', #31879, #10547, #35331 ) ;
#34924=CARTESIAN_POINT ( 'NONE',  ( 13.67111072870491206, 27.95752071293676266, 10.49999999999999822 ) ) ;
#34925=DIRECTION ( 'NONE',  ( -0.8090169943749426773, 0.5877852522924797984, 0.000000000000000000 ) ) ;
#34926=ORIENTED_EDGE ( 'NONE', *, *, #37728, .F. ) ;
#34928=EDGE_CURVE ( 'NONE', #9701, #13281, #35255, .T. ) ;
#34929=CARTESIAN_POINT ( 'NONE',  ( 14.31603901957230462, 19.98981538725069740, 7.500000000000010658 ) ) ;
#34932=EDGE_CURVE ( 'NONE', #11008, #21646, #15245, .T. ) ;
#34933=CARTESIAN_POINT ( 'NONE',  ( -0.5000000000000004441, 37.00000000000000711, 7.000000000000000000 ) ) ;
#34934=DIRECTION ( 'NONE',  ( -0.000000000000000000, -0.000000000000000000, -1.000000000000000000 ) ) ;
#34938=ORIENTED_EDGE ( 'NONE', *, *, #6213, .F. ) ;
#34940=AXIS2_PLACEMENT_3D ( 'NONE', #10151, #22523, #12987 ) ;
#34941=ADVANCED_FACE ( 'NONE', ( #26102 ), #38299, .F. ) ;
#34944=AXIS2_PLACEMENT_3D ( 'NONE', #33514, #12749, #18459 ) ;
#34946=CARTESIAN_POINT ( 'NONE',  ( -10.49474413300070097, 21.89971208337388120, 10.50000000000000000 ) ) ;
#34948=CIRCLE ( 'NONE', #34852, 0.5000000000000004441 ) ;
#34949=CARTESIAN_POINT ( 'NONE',  ( 3.503793317224329851, 8.420815634768676006, 7.000000000000000000 ) ) ;
#34950=EDGE_LOOP ( 'NONE', ( #7813, #34782, #15642 ) ) ;
#34953=CYLINDRICAL_SURFACE ( 'NONE', #8507, 0.4999999999999995559 ) ;
#34955=EDGE_CURVE ( 'NONE', #6691, #4778, #26941, .T. ) ;
#34956=CARTESIAN_POINT ( 'NONE',  ( -13.63581098909220479, 27.45627467658446008, 9.000000000000001776 ) ) ;
#34957=EDGE_CURVE ( 'NONE', #7636, #22687, #2272, .T. ) ;
#34960=ORIENTED_EDGE ( 'NONE', *, *, #20306, .F. ) ;
#34962=CARTESIAN_POINT ( 'NONE',  ( 13.22516817658079802, 40.70288237343621063, 7.000000000000000000 ) ) ;
#34973=CIRCLE ( 'NONE', #27176, 15.00000000000000000 ) ;
#34975=CARTESIAN_POINT ( 'NONE',  ( 5.184280209938516570, 31.68549066217151733, 11.00000000000000000 ) ) ;
#34978=EDGE_CURVE ( 'NONE', #33679, #113, #5504, .T. ) ;
#34980=CYLINDRICAL_SURFACE ( 'NONE', #20938, 0.5000000000000007772 ) ;
#34981=ORIENTED_EDGE ( 'NONE', *, *, #35003, .F. ) ;
#34983=EDGE_CURVE ( 'NONE', #747, #3751, #19604, .T. ) ;
#34985=CARTESIAN_POINT ( 'NONE',  ( -5.767236651883568044, 13.71142893291686171, 10.00000000000000000 ) ) ;
#34986=VERTEX_POINT ( 'NONE', #25906 ) ;
#34988=LINE ( 'NONE', #38429, #11161 ) ;
#34989=ORIENTED_EDGE ( 'NONE', *, *, #29167, .T. ) ;
#34996=LINE ( 'NONE', #28290, #13693 ) ;
#35000=DIRECTION ( 'NONE',  ( 1.000000000000000000, 0.000000000000000000, 0.000000000000000000 ) ) ;
#35001=CIRCLE ( 'NONE', #31747, 0.5000000000000005551 ) ;
#35003=EDGE_CURVE ( 'NONE', #39848, #20455, #10719, .T. ) ;
#35008=CARTESIAN_POINT ( 'NONE',  ( -14.45127508551987994, 26.52006039836903284, 7.493552897947291846 ) ) ;
#35009=ORIENTED_EDGE ( 'NONE', *, *, #13084, .F. ) ;
#35014=FACE_OUTER_BOUND ( 'NONE', #28974, .T. ) ;
#35016=EDGE_LOOP ( 'NONE', ( #35186, #15371, #9520 ) ) ;
#35019=EDGE_LOOP ( 'NONE', ( #14205, #11645, #7837, #19602, #15746 ) ) ;
#35024=CIRCLE ( 'NONE', #24001, 1.000000000000004441 ) ;
#35025=EDGE_LOOP ( 'NONE', ( #15938, #18053, #25611 ) ) ;
#35032=EDGE_CURVE ( 'NONE', #1897, #1674, #35262, .T. ) ;
#35043=CARTESIAN_POINT ( 'NONE',  ( 0.000000000000000000, 22.50000000000000355, 7.000000000000000000 ) ) ;
#35045=DIRECTION ( 'NONE',  ( -0.7431448254773862505, 0.6691306063588670083, 0.000000000000000000 ) ) ;
#35047=ORIENTED_EDGE ( 'NONE', *, *, #29221, .T. ) ;
#35049=CARTESIAN_POINT ( 'NONE',  ( 3.992867117591230919, 8.524771480177550487, 10.49999999999999289 ) ) ;
#35051=DIRECTION ( 'NONE',  ( 0.9135454576426059736, 0.4067366430757889395, -0.000000000000000000 ) ) ;
#35052=FACE_OUTER_BOUND ( 'NONE', #10967, .T. ) ;
#35054=FACE_OUTER_BOUND ( 'NONE', #3028, .T. ) ;
#35055=ORIENTED_EDGE ( 'NONE', *, *, #19233, .T. ) ;
#35059=ADVANCED_FACE ( 'NONE', ( #4175 ), #38103, .T. ) ;
#35060=CARTESIAN_POINT ( 'NONE',  ( 14.86556419889027048, 20.43481210330100240, 7.000000000000000000 ) ) ;
#35066=CARTESIAN_POINT ( 'NONE',  ( 14.03291393139918597, 26.53383901973350589, 10.99387789255784220 ) ) ;
#35069=AXIS2_PLACEMENT_3D ( 'NONE', #8617, #15110, #24056 ) ;
#35073=VERTEX_POINT ( 'NONE', #22459 ) ;
#35082=ORIENTED_EDGE ( 'NONE', *, *, #34094, .F. ) ;
#35085=EDGE_CURVE ( 'NONE', #4444, #19049, #2955, .T. ) ;
#35088=ORIENTED_EDGE ( 'NONE', *, *, #32736, .F. ) ;
#35089=ORIENTED_EDGE ( 'NONE', *, *, #15247, .F. ) ;
#35092=VECTOR ( 'NONE', #20371, 999.9999999999998863 ) ;
#35093=CARTESIAN_POINT ( 'NONE',  ( 5.644276917315719899, 36.40655018617690786, 10.49999999999999822 ) ) ;
#35094=ORIENTED_EDGE ( 'NONE', *, *, #8676, .F. ) ;
#35096=AXIS2_PLACEMENT_3D ( 'NONE', #31148, #28688, #6740 ) ;
#35098=CARTESIAN_POINT ( 'NONE',  ( 10.36702044712426840, 31.16169077310587809, 9.500000000000000000 ) ) ;
#35100=CARTESIAN_POINT ( 'NONE',  ( 2.525645716490518389, 8.212903943950921715, 7.499999999999990230 ) ) ;
#35101=EDGE_CURVE ( 'NONE', #3204, #20104, #16176, .T. ) ;
#35102=CARTESIAN_POINT ( 'NONE',  ( 2.629601561899395534, 7.723830143584016206, 10.49999999999999822 ) ) ;
#35104=LINE ( 'NONE', #29, #5587 ) ;
#35105=ORIENTED_EDGE ( 'NONE', *, *, #22999, .T. ) ;
#35107=PLANE ( 'NONE',  #20039 ) ;
#35110=ADVANCED_FACE ( 'NONE', ( #35468 ), #7458, .T. ) ;
#35111=DIRECTION ( 'NONE',  ( -0.000000000000000000, -0.000000000000000000, 1.000000000000000000 ) ) ;
#35120=CARTESIAN_POINT ( 'NONE',  ( -2.568190708544555445, 12.82247983807085134, 10.50000000000000533 ) ) ;
#35121=CARTESIAN_POINT ( 'NONE',  ( 3.713592597587208832, 7.966960743906818188, 7.000000000000000000 ) ) ;
#35125=VECTOR ( 'NONE', #3814, 1000.000000000000000 ) ;
#35126=LINE ( 'NONE', #12982, #114 ) ;
#35130=CARTESIAN_POINT ( 'NONE',  ( -14.26377478793851061, 19.49255443956674583, 7.000000000000000000 ) ) ;
#35132=LINE ( 'NONE', #37776, #34905 ) ;
#35133=EDGE_CURVE ( 'NONE', #11406, #17826, #15270, .T. ) ;
#35136=CARTESIAN_POINT ( 'NONE',  ( -4.524139159579198655, 31.43208625488816566, 10.00000000000000000 ) ) ;
#35137=EDGE_LOOP ( 'NONE', ( #24193, #38180, #28124 ) ) ;
#35139=ORIENTED_EDGE ( 'NONE', *, *, #37446, .T. ) ;
#35140=VECTOR ( 'NONE', #33347, 1000.000000000000114 ) ;
#35142=CARTESIAN_POINT ( 'NONE',  ( 9.303655249773155944, 10.73386218874824216, 7.000000000000000000 ) ) ;
#35143=DIRECTION ( 'NONE',  ( -0.9945218953682730678, 0.1045284632676563991, 0.000000000000000000 ) ) ;
#35146=VERTEX_POINT ( 'NONE', #7416 ) ;
#35149=DIRECTION ( 'NONE',  ( -0.2079116908177663092, -0.9781476007338041345, 0.000000000000000000 ) ) ;
#35156=DIRECTION ( 'NONE',  ( -0.000000000000000000, -0.000000000000000000, -1.000000000000000000 ) ) ;
#35158=CARTESIAN_POINT ( 'NONE',  ( -2.525645716490710679, 8.212903943950959018, 7.499999999999997335 ) ) ;
#35160=ORIENTED_EDGE ( 'NONE', *, *, #14006, .F. ) ;
#35164=VECTOR ( 'NONE', #23895, 1000.000000000000000 ) ;
#35165=DIRECTION ( 'NONE',  ( -0.3583679495453008790, 0.9335804264972015210, 0.000000000000000000 ) ) ;
#35166=ORIENTED_EDGE ( 'NONE', *, *, #8732, .F. ) ;
#35167=ORIENTED_EDGE ( 'NONE', *, *, #21207, .T. ) ;
#35171=CIRCLE ( 'NONE', #12457, 6.000000000000001776 ) ;
#35173=CARTESIAN_POINT ( 'NONE',  ( 4.524139159579314118, 31.43208625488810171, 10.49999999999999822 ) ) ;
#35174=ORIENTED_EDGE ( 'NONE', *, *, #5073, .T. ) ;
#35178=ORIENTED_EDGE ( 'NONE', *, *, #4712, .T. ) ;
#35180=CYLINDRICAL_SURFACE ( 'NONE', #33901, 6.000000000000000888 ) ;
#35181=ORIENTED_EDGE ( 'NONE', *, *, #25127, .F. ) ;
#35182=EDGE_CURVE ( 'NONE', #7898, #12750, #26961, .T. ) ;
#35184=CARTESIAN_POINT ( 'NONE',  ( 0.6108529249776364356, 37.48755679569042343, 7.000000000000000000 ) ) ;
#35186=ORIENTED_EDGE ( 'NONE', *, *, #1227, .T. ) ;
#35188=CARTESIAN_POINT ( 'NONE',  ( -14.81329996725647469, 19.93755115561707569, 10.49999999999999467 ) ) ;
#35190=DIRECTION ( 'NONE',  ( -0.8660254037844432595, -0.4999999999999921729, 0.000000000000000000 ) ) ;
#35191=CIRCLE ( 'NONE', #8609, 0.5000000000000002220 ) ;
#35192=DIRECTION ( 'NONE',  ( 1.000000000000000000, 0.000000000000000000, 0.000000000000000000 ) ) ;
#35193=EDGE_CURVE ( 'NONE', #17610, #29868, #38305, .T. ) ;
#35194=CONICAL_SURFACE ( 'NONE', #12522, 0.9999999999999991118, 0.7853981633974502774 ) ;
#35202=VERTEX_POINT ( 'NONE', #31808 ) ;
#35208=VERTEX_POINT ( 'NONE', #10274 ) ;
#35210=PLANE ( 'NONE',  #9270 ) ;
#35215=LINE ( 'NONE', #23633, #9511 ) ;
#35216=VECTOR ( 'NONE', #15710, 1000.000000000000000 ) ;
#35217=VERTEX_POINT ( 'NONE', #35060 ) ;
#35222=ORIENTED_EDGE ( 'NONE', *, *, #11723, .F. ) ;
#35224=LINE ( 'NONE', #22828, #21309 ) ;
#35226=CARTESIAN_POINT ( 'NONE',  ( 14.42035624161478857, 26.65972665747660031, 10.49999999999999822 ) ) ;
#35227=EDGE_LOOP ( 'NONE', ( #30047, #19184, #14471, #1895 ) ) ;
#35228=EDGE_CURVE ( 'NONE', #40197, #13640, #7215, .T. ) ;
#35232=CIRCLE ( 'NONE', #20966, 0.5000000000000004441 ) ;
#35234=ORIENTED_EDGE ( 'NONE', *, *, #13517, .T. ) ;
#35236=AXIS2_PLACEMENT_3D ( 'NONE', #13709, #22446, #28750 ) ;
#35237=CARTESIAN_POINT ( 'NONE',  ( -14.04783364825881975, 26.18819932152426233, 10.66666666666667140 ) ) ;
#35238=VECTOR ( 'NONE', #14962, 1000.000000000000000 ) ;
#35239=FACE_OUTER_BOUND ( 'NONE', #1904, .T. ) ;
#35240=LINE ( 'NONE', #22435, #34048 ) ;
#35242=ADVANCED_FACE ( 'NONE', ( #4584 ), #28896, .T. ) ;
#35245=DIRECTION ( 'NONE',  ( -0.3090169943749450643, 0.9510565162951544194, -0.000000000000000000 ) ) ;
#35246=EDGE_CURVE ( 'NONE', #2697, #5248, #6083, .T. ) ;
#35247=DIRECTION ( 'NONE',  ( -0.8090169943749505599, -0.5877852522924689183, 0.000000000000000000 ) ) ;
#35248=VERTEX_POINT ( 'NONE', #39307 ) ;
#35249=CARTESIAN_POINT ( 'NONE',  ( -6.856875760696268252, 35.58019112794178795, 10.49999999999999822 ) ) ;
#35253=DIRECTION ( 'NONE',  ( -1.224646799147351235E-16, 1.000000000000000000, 0.000000000000000000 ) ) ;
#35255=LINE ( 'NONE', #23668, #24328 ) ;
#35258=AXIS2_PLACEMENT_3D ( 'NONE', #6299, #13399, #28841 ) ;
#35262=LINE ( 'NONE', #13114, #8133 ) ;
#35264=ORIENTED_EDGE ( 'NONE', *, *, #1631, .F. ) ;
#35266=ORIENTED_EDGE ( 'NONE', *, *, #34679, .T. ) ;
#35272=VECTOR ( 'NONE', #17531, 1000.000000000000114 ) ;
#35278=FACE_OUTER_BOUND ( 'NONE', #23979, .T. ) ;
#35282=CIRCLE ( 'NONE', #31388, 0.5000000000000004441 ) ;
#35284=ORIENTED_EDGE ( 'NONE', *, *, #38192, .T. ) ;
#35285=DIRECTION ( 'NONE',  ( 0.7431448254773954654, 0.6691306063588569053, -0.000000000000000000 ) ) ;
#35286=DIRECTION ( 'NONE',  ( -0.2079116908177663092, -0.9781476007338040235, 0.000000000000000000 ) ) ;
#35291=CIRCLE ( 'NONE', #15160, 1.000000000000000000 ) ;
#35293=CARTESIAN_POINT ( 'NONE',  ( 12.49038105676653743, 14.13397459621550745, 11.00000000000000000 ) ) ;
#35294=DIRECTION ( 'NONE',  ( 0.000000000000000000, -0.000000000000000000, -1.000000000000000000 ) ) ;
#35295=LINE ( 'NONE', #7453, #36341 ) ;
#35296=EDGE_LOOP ( 'NONE', ( #21635, #33232, #14696 ) ) ;
#35298=DIRECTION ( 'NONE',  ( 1.000000000000000000, -1.734723475976802361E-14, 0.000000000000000000 ) ) ;
#35299=CARTESIAN_POINT ( 'NONE',  ( -12.68475447279705648, 27.14725768220950286, 9.500000000000000000 ) ) ;
#35300=DIRECTION ( 'NONE',  ( 1.000000000000000000, 0.000000000000000000, -0.000000000000000000 ) ) ;
#35301=CYLINDRICAL_SURFACE ( 'NONE', #37900, 6.000000000000001776 ) ;
#35302=DIRECTION ( 'NONE',  ( -0.6691306063588671194, -0.7431448254773861395, 0.000000000000000000 ) ) ;
#35303=AXIS2_PLACEMENT_3D ( 'NONE', #22753, #10578, #16067 ) ;
#35305=DIRECTION ( 'NONE',  ( 0.000000000000000000, 0.000000000000000000, -1.000000000000000000 ) ) ;
#35308=LINE ( 'NONE', #29009, #10283 ) ;
#35310=EDGE_CURVE ( 'NONE', #11163, #21446, #36466, .T. ) ;
#35322=CARTESIAN_POINT ( 'NONE',  ( -6.354454053420243831, 35.54304081427989814, 7.000000000000000000 ) ) ;
#35326=B_SPLINE_CURVE_WITH_KNOTS ( 'NONE', 3,
 ( #15140, #6189, #39912, #5985 ),
 .UNSPECIFIED., .F., .F.,
 ( 4, 4 ),
 ( 8.673617379884035472E-19, 0.0006014480309583149914 ),
 .UNSPECIFIED. ) ;
#35328=CARTESIAN_POINT ( 'NONE',  ( -13.97557076678966403, 21.53386246193713305, 9.500000000000000000 ) ) ;
#35329=EDGE_LOOP ( 'NONE', ( #27504, #30391, #35089 ) ) ;
#35331=DIRECTION ( 'NONE',  ( -1.000000000000000000, 0.000000000000000000, 0.000000000000000000 ) ) ;
#35332=EDGE_CURVE ( 'NONE', #10420, #20455, #1746, .T. ) ;
#35333=DIRECTION ( 'NONE',  ( 0.9510565162951543083, 0.3090169943749450088, 0.000000000000000000 ) ) ;
#35335=ORIENTED_EDGE ( 'NONE', *, *, #29948, .T. ) ;
#35339=CIRCLE ( 'NONE', #30795, 6.000000000000005329 ) ;
#35340=EDGE_CURVE ( 'NONE', #13129, #6246, #36069, .T. ) ;
#35341=VERTEX_POINT ( 'NONE', #4986 ) ;
#35345=DIRECTION ( 'NONE',  ( 0.9135454576426059736, 0.4067366430757889395, -0.000000000000000000 ) ) ;
#35346=VECTOR ( 'NONE', #23998, 1000.000000000000000 ) ;
#35350=FACE_OUTER_BOUND ( 'NONE', #20850, .T. ) ;
#35351=ORIENTED_EDGE ( 'NONE', *, *, #25892, .F. ) ;
#35354=CARTESIAN_POINT ( 'NONE',  ( -8.472151273871419974, 28.78272654129072095, 10.49999999999999822 ) ) ;
#35355=FACE_OUTER_BOUND ( 'NONE', #18229, .T. ) ;
#35358=ORIENTED_EDGE ( 'NONE', *, *, #30515, .F. ) ;
#35360=CARTESIAN_POINT ( 'NONE',  ( -2.036571916123810055, 8.108948098542073879, 10.50000000000000355 ) ) ;
#35361=EDGE_CURVE ( 'NONE', #36944, #19274, #17397, .T. ) ;
#35362=EDGE_CURVE ( 'NONE', #17187, #24136, #34099, .T. ) ;
#35364=DIRECTION ( 'NONE',  ( 1.000000000000000000, 0.000000000000000000, 0.000000000000000000 ) ) ;
#35366=VERTEX_POINT ( 'NONE', #23872 ) ;
#35370=CARTESIAN_POINT ( 'NONE',  ( -9.356056665764020508, 26.06569820189716324, 10.50000000000000533 ) ) ;
#35371=ORIENTED_EDGE ( 'NONE', *, *, #712, .F. ) ;
#35372=ORIENTED_EDGE ( 'NONE', *, *, #27047, .F. ) ;
#35376=DIRECTION ( 'NONE',  ( 1.000000000000000000, 0.000000000000000000, 0.000000000000000000 ) ) ;
#35380=LINE ( 'NONE', #20346, #33217 ) ;
#35381=VERTEX_POINT ( 'NONE', #21028 ) ;
#35384=DIRECTION ( 'NONE',  ( 0.5000000000000039968, 0.8660254037844363761, 0.000000000000000000 ) ) ;
#35388=FACE_OUTER_BOUND ( 'NONE', #20370, .T. ) ;
#35391=CARTESIAN_POINT ( 'NONE',  ( -9.038010526469660633, 11.76154733104328010, 10.50000000000000000 ) ) ;
#35393=ORIENTED_EDGE ( 'NONE', *, *, #3462, .T. ) ;
#35396=DIRECTION ( 'NONE',  ( 0.5254827454987550661, -0.4731467892558230415, -0.7071067811865451302 ) ) ;
#35398=CARTESIAN_POINT ( 'NONE',  ( 13.53057405073934838, 22.08338764125490528, 10.50000000000000000 ) ) ;
#35399=CARTESIAN_POINT ( 'NONE',  ( 9.331903152615748098, 11.35703883385568780, 10.49999999999999645 ) ) ;
#35401=AXIS2_PLACEMENT_3D ( 'NONE', #2530, #39695, #21015 ) ;
#35409=EDGE_LOOP ( 'NONE', ( #30564, #8103, #8957 ) ) ;
#35411=EDGE_LOOP ( 'NONE', ( #30923, #28182, #118 ) ) ;
#35414=CARTESIAN_POINT ( 'NONE',  ( -13.94482798346716379, 26.50521816028930999, 10.99999999999999289 ) ) ;
#35419=VERTEX_POINT ( 'NONE', #29770 ) ;
#35427=DIRECTION ( 'NONE',  ( -0.000000000000000000, -0.000000000000000000, -1.000000000000000000 ) ) ;
#35429=EDGE_LOOP ( 'NONE', ( #9480, #27636, #11700, #35936 ) ) ;
#35431=LINE ( 'NONE', #10040, #14148 ) ;
#35433=CIRCLE ( 'NONE', #402, 0.5000000000000000000 ) ;
#35438=CIRCLE ( 'NONE', #17926, 1.000000000000004441 ) ;
#35442=VERTEX_POINT ( 'NONE', #8438 ) ;
#35443=ADVANCED_FACE ( 'NONE', ( #4784 ), #33236, .F. ) ;
#35446=PLANE ( 'NONE',  #33599 ) ;
#35447=ADVANCED_FACE ( 'NONE', ( #29363 ), #1540, .F. ) ;
#35448=DIRECTION ( 'NONE',  ( -0.7032331762534009822, 0.07391278520356894810, 0.7071067811865506814 ) ) ;
#35449=CARTESIAN_POINT ( 'NONE',  ( -2.518583951651248931, 7.712953814960721743, 7.499999999999997335 ) ) ;
#35450=LINE ( 'NONE', #4768, #21663 ) ;
#35453=DIRECTION ( 'NONE',  ( -0.9135454576426005335, 0.4067366430758009299, -0.000000000000000000 ) ) ;
#35454=CYLINDRICAL_SURFACE ( 'NONE', #25901, 0.4999999999999996669 ) ;
#35456=EDGE_CURVE ( 'NONE', #614, #30787, #10081, .T. ) ;
#35458=DIRECTION ( 'NONE',  ( 0.4156269377774612361, 0.5720614028176856936, -0.7071067811865417996 ) ) ;
#35459=LINE ( 'NONE', #32417, #5406 ) ;
#35460=EDGE_CURVE ( 'NONE', #15406, #30242, #18577, .T. ) ;
#35463=EDGE_LOOP ( 'NONE', ( #5108, #14809, #36231 ) ) ;
#35466=AXIS2_PLACEMENT_3D ( 'NONE', #32212, #7823, #4984 ) ;
#35468=FACE_OUTER_BOUND ( 'NONE', #28508, .T. ) ;
#35474=DIRECTION ( 'NONE',  ( 0.000000000000000000, 0.7071067811865500152, -0.7071067811865451302 ) ) ;
#35480=ORIENTED_EDGE ( 'NONE', *, *, #4069, .F. ) ;
#35482=LINE ( 'NONE', #7029, #32273 ) ;
#35484=CARTESIAN_POINT ( 'NONE',  ( 1.734965421685031872, 7.600674680189132282, 7.000000000000000000 ) ) ;
#35489=ORIENTED_EDGE ( 'NONE', *, *, #19664, .F. ) ;
#35490=EDGE_CURVE ( 'NONE', #2539, #7713, #6817, .T. ) ;
#35491=CARTESIAN_POINT ( 'NONE',  ( 14.47283171447379502, 21.48159823030311344, 7.000000000000000000 ) ) ;
#35493=DIRECTION ( 'NONE',  ( 0.04273212933193662466, -0.8153776007405469928, 0.5773502691896383876 ) ) ;
#35497=VERTEX_POINT ( 'NONE', #5577 ) ;
#35501=DIRECTION ( 'NONE',  ( 1.000000000000000000, 0.000000000000000000, 0.000000000000000000 ) ) ;
#35505=DIRECTION ( 'NONE',  ( -1.000000000000000000, 0.000000000000000000, 0.000000000000000000 ) ) ;
#35507=DIRECTION ( 'NONE',  ( 0.5000000000000039968, 0.8660254037844363761, 0.000000000000000000 ) ) ;
#35511=EDGE_LOOP ( 'NONE', ( #36753, #30258, #34677, #21572 ) ) ;
#35514=CARTESIAN_POINT ( 'NONE',  ( -0.6830608540011002816, 37.47223625998410057, 10.49999999999999822 ) ) ;
#35516=DIRECTION ( 'NONE',  ( 1.000000000000000000, 0.000000000000000000, 0.000000000000000000 ) ) ;
#35519=CARTESIAN_POINT ( 'NONE',  ( -1.158196024796639412, -0.5060543600718802049, 10.00000000000000000 ) ) ;
#35520=VECTOR ( 'NONE', #28879, 1000.000000000000227 ) ;
#35521=CIRCLE ( 'NONE', #16055, 0.4999999999999999445 ) ;
#35526=CARTESIAN_POINT ( 'NONE',  ( -2.672146553953452575, 12.33340603770394139, 10.50000000000000000 ) ) ;
#35527=ORIENTED_EDGE ( 'NONE', *, *, #26789, .T. ) ;
#35530=VERTEX_POINT ( 'NONE', #30964 ) ;
#35533=CARTESIAN_POINT ( 'NONE',  ( 5.464578388833499112, 36.46941714767122278, 7.485646746502379933 ) ) ;
#35535=DIRECTION ( 'NONE',  ( 0.5000000000000038858, 0.8660254037844364872, -0.000000000000000000 ) ) ;
#35536=LINE ( 'NONE', #29433, #5726 ) ;
#35537=ORIENTED_EDGE ( 'NONE', *, *, #18881, .F. ) ;
#35539=EDGE_LOOP ( 'NONE', ( #19890, #15489, #35371, #19106 ) ) ;
#35541=EDGE_LOOP ( 'NONE', ( #11825, #33908, #5013 ) ) ;
#35544=AXIS2_PLACEMENT_3D ( 'NONE', #830, #22555, #18525 ) ;
#35545=FACE_OUTER_BOUND ( 'NONE', #3896, .T. ) ;
#35546=DIRECTION ( 'NONE',  ( 1.000000000000000000, 0.000000000000000000, 0.000000000000000000 ) ) ;
#35548=VECTOR ( 'NONE', #16495, 1000.000000000000000 ) ;
#35550=CYLINDRICAL_SURFACE ( 'NONE', #3849, 6.000000000000005329 ) ;
#35552=CARTESIAN_POINT ( 'NONE',  ( 12.53024597560964359, 27.62278594035691626, 10.50000000000000000 ) ) ;
#35554=CARTESIAN_POINT ( 'NONE',  ( 6.811226782241714517, 35.33967249274190436, 11.00000000000000000 ) ) ;
#35558=ORIENTED_EDGE ( 'NONE', *, *, #10056, .F. ) ;
#35559=DIRECTION ( 'NONE',  ( 0.8090169943749426773, -0.5877852522924796874, 0.000000000000000000 ) ) ;
#35560=LINE ( 'NONE', #32924, #27250 ) ;
#35561=EDGE_CURVE ( 'NONE', #29026, #10996, #17228, .T. ) ;
#35563=CARTESIAN_POINT ( 'NONE',  ( 13.63581098909226874, 27.45627467658428955, 7.000000000000000000 ) ) ;
#35564=CARTESIAN_POINT ( 'NONE',  ( -14.49848586288629271, 20.47339359108951129, 11.00000000000000000 ) ) ;
#35565=VERTEX_POINT ( 'NONE', #12076 ) ;
#35570=CARTESIAN_POINT ( 'NONE',  ( -14.57486473880221745, 26.18419839932921533, 11.00000000000000000 ) ) ;
#35571=EDGE_CURVE ( 'NONE', #9605, #12345, #14931, .T. ) ;
#35572=ORIENTED_EDGE ( 'NONE', *, *, #21195, .T. ) ;
#35573=ORIENTED_EDGE ( 'NONE', *, *, #8812, .T. ) ;
#35576=CARTESIAN_POINT ( 'NONE',  ( -12.74038105676665467, 14.56698729810789850, 10.49999999999999822 ) ) ;
#35577=B_SPLINE_CURVE_WITH_KNOTS ( 'NONE', 3,
 ( #32908, #26797, #5060, #17472, #29843, #5262 ),
 .UNSPECIFIED., .F., .F.,
 ( 4, 2, 4 ),
 ( 0.000000000000000000, 0.5000000000000000000, 1.000000000000000000 ),
 .UNSPECIFIED. ) ;
#35578=AXIS2_PLACEMENT_3D ( 'NONE', #1767, #5211, #26342 ) ;
#35579=AXIS2_PLACEMENT_3D ( 'NONE', #10444, #13686, #16750 ) ;
#35581=CARTESIAN_POINT ( 'NONE',  ( -11.66932856646905314, 37.85852258240264234, 10.00000000000000000 ) ) ;
#35582=ORIENTED_EDGE ( 'NONE', *, *, #27318, .F. ) ;
#35584=CARTESIAN_POINT ( 'NONE',  ( -10.69300419909361466, 32.80084059136108721, 10.87262190629279424 ) ) ;
#35585=CARTESIAN_POINT ( 'NONE',  ( 6.651296319737278750, 27.81603774131160023, 7.000000000000000000 ) ) ;
#35595=EDGE_CURVE ( 'NONE', #23174, #18033, #24272, .T. ) ;
#35598=EDGE_CURVE ( 'NONE', #7720, #7701, #18381, .T. ) ;
#35600=CARTESIAN_POINT ( 'NONE',  ( 6.385371355716897845, 45.28367711306903942, 10.00000000000000000 ) ) ;
#35602=CARTESIAN_POINT ( 'NONE',  ( -12.37435565298220119, 15.93301270189233598, 9.500000000000000000 ) ) ;
#35603=EDGE_LOOP ( 'NONE', ( #34989, #34085, #30687, #14718 ) ) ;
#35604=CYLINDRICAL_SURFACE ( 'NONE', #4617, 0.5000000000000004441 ) ;
#35607=LINE ( 'NONE', #20168, #36575 ) ;
#35610=DIRECTION ( 'NONE',  ( -0.9135454576426048634, -0.4067366430757912710, 0.000000000000000000 ) ) ;
#35612=DIRECTION ( 'NONE',  ( -0.000000000000000000, -0.000000000000000000, 1.000000000000000000 ) ) ;
#35615=ORIENTED_EDGE ( 'NONE', *, *, #22556, .F. ) ;
#35620=DIRECTION ( 'NONE',  ( -0.4999999999999933942, 0.8660254037844425934, 0.000000000000000000 ) ) ;
#35622=ORIENTED_EDGE ( 'NONE', *, *, #16069, .T. ) ;
#35624=EDGE_LOOP ( 'NONE', ( #31538, #24190, #3485, #2660, #20757 ) ) ;
#35626=CARTESIAN_POINT ( 'NONE',  ( 13.05736835487433289, 16.11602540378438420, 7.000000000000000000 ) ) ;
#35628=CARTESIAN_POINT ( 'NONE',  ( -0.5000000000000004441, 36.50000000000000711, 7.000000000000000000 ) ) ;
#35640=AXIS2_PLACEMENT_3D ( 'NONE', #20693, #36522, #23727 ) ;
#35644=ADVANCED_FACE ( 'NONE', ( #88 ), #27319, .T. ) ;
#35645=ORIENTED_EDGE ( 'NONE', *, *, #10776, .T. ) ;
#35650=DIRECTION ( 'NONE',  ( 0.000000000000000000, 0.000000000000000000, 1.000000000000000000 ) ) ;
#35653=DIRECTION ( 'NONE',  ( 1.000000000000000000, 0.000000000000000000, 0.000000000000000000 ) ) ;
#35655=EDGE_LOOP ( 'NONE', ( #39587, #37038, #12025, #17145, #21577, #7529, #5948 ) ) ;
#35657=CARTESIAN_POINT ( 'NONE',  ( -6.513333500388862163, 35.89988989478917603, 10.82238861112326234 ) ) ;
#35658=DIRECTION ( 'NONE',  ( -0.9510565162951518658, 0.3090169943749528914, 0.000000000000000000 ) ) ;
#35660=DIRECTION ( 'NONE',  ( -0.000000000000000000, -0.000000000000000000, -1.000000000000000000 ) ) ;
#35661=CARTESIAN_POINT ( 'NONE',  ( -14.70550430380713003, 20.45163507617063203, 10.87262190629282799 ) ) ;
#35662=EDGE_CURVE ( 'NONE', #23702, #33679, #287, .T. ) ;
#35666=VERTEX_POINT ( 'NONE', #2543 ) ;
#35671=CARTESIAN_POINT ( 'NONE',  ( -8.118377661053488126, 10.47536095541708967, 7.000000000000000000 ) ) ;
#35677=DIRECTION ( 'NONE',  ( -0.000000000000000000, -0.000000000000000000, -1.000000000000000000 ) ) ;
#35683=ORIENTED_EDGE ( 'NONE', *, *, #11866, .T. ) ;
#35685=DIRECTION ( 'NONE',  ( -0.7071067811865517916, 0.000000000000000000, -0.7071067811865432429 ) ) ;
#35687=DIRECTION ( 'NONE',  ( 0.8090169943749504489, 0.5877852522924689183, 0.000000000000000000 ) ) ;
#35688=ORIENTED_EDGE ( 'NONE', *, *, #20615, .F. ) ;
#35691=ORIENTED_EDGE ( 'NONE', *, *, #24693, .T. ) ;
#35694=B_SPLINE_CURVE_WITH_KNOTS ( 'NONE', 3,
 ( #17892, #35970, #30071, #30274, #14632, #5880 ),
 .UNSPECIFIED., .F., .F.,
 ( 4, 2, 4 ),
 ( 0.000000000000000000, 0.5000000000000000000, 1.000000000000000000 ),
 .UNSPECIFIED. ) ;
#35698=ADVANCED_FACE ( 'NONE', ( #33635 ), #5782, .T. ) ;
#35700=AXIS2_PLACEMENT_3D ( 'NONE', #20125, #14219, #26610 ) ;
#35701=ORIENTED_EDGE ( 'NONE', *, *, #13218, .F. ) ;
#35708=DIRECTION ( 'NONE',  ( -0.8090169943749430104, 0.5877852522924791323, 0.000000000000000000 ) ) ;
#35709=DIRECTION ( 'NONE',  ( -0.7071067811865449082, 0.7071067811865501263, 0.000000000000000000 ) ) ;
#35713=CARTESIAN_POINT ( 'NONE',  ( 9.284827327736225655, 10.70480225628988791, 10.49999999999999822 ) ) ;
#35716=EDGE_LOOP ( 'NONE', ( #32181, #16403, #15970, #27118 ) ) ;
#35717=VECTOR ( 'NONE', #20262, 1000.000000000000114 ) ;
#35721=ADVANCED_FACE ( 'NONE', ( #38457 ), #31360, .T. ) ;
#35723=CARTESIAN_POINT ( 'NONE',  ( 14.84160187385922036, 20.32586711126977974, 7.000000000000000000 ) ) ;
#35727=EDGE_CURVE ( 'NONE', #29069, #16528, #15923, .T. ) ;
#35733=ORIENTED_EDGE ( 'NONE', *, *, #39089, .F. ) ;
#35734=VECTOR ( 'NONE', #25597, 1000.000000000000000 ) ;
#35736=ORIENTED_EDGE ( 'NONE', *, *, #28179, .T. ) ;
#35737=CARTESIAN_POINT ( 'NONE',  ( 14.70895476143395442, 21.92515157238277013, 10.49999999999999822 ) ) ;
#35738=ORIENTED_EDGE ( 'NONE', *, *, #37029, .F. ) ;
#35739=DIRECTION ( 'NONE',  ( 0.000000000000000000, 0.000000000000000000, -1.000000000000000000 ) ) ;
#35740=CARTESIAN_POINT ( 'NONE',  ( 9.067459072332447079, 10.87036407658120041, 10.94387467463491603 ) ) ;
#35741=ORIENTED_EDGE ( 'NONE', *, *, #9261, .F. ) ;
#35743=ADVANCED_FACE ( 'NONE', ( #22607 ), #37848, .T. ) ;
#35744=VERTEX_POINT ( 'NONE', #25855 ) ;
#35747=CIRCLE ( 'NONE', #39617, 15.00000000000000000 ) ;
#35748=ORIENTED_EDGE ( 'NONE', *, *, #1055, .F. ) ;
#35750=CARTESIAN_POINT ( 'NONE',  ( 10.67401460142006897, 33.03905331147102231, 7.485646746502373716 ) ) ;
#35751=ORIENTED_EDGE ( 'NONE', *, *, #36962, .F. ) ;
#35754=DIRECTION ( 'NONE',  ( 0.000000000000000000, 0.000000000000000000, 1.000000000000000000 ) ) ;
#35755=ORIENTED_EDGE ( 'NONE', *, *, #2575, .F. ) ;
#35757=CARTESIAN_POINT ( 'NONE',  ( 7.713869163865849643, 10.18146832927074996, 11.00000000000000000 ) ) ;
#35759=DIRECTION ( 'NONE',  ( -1.000000000000000000, 0.000000000000000000, 0.000000000000000000 ) ) ;
#35764=LINE ( 'NONE', #13814, #38267 ) ;
#35765=EDGE_CURVE ( 'NONE', #35530, #25471, #37371, .T. ) ;
#35767=CYLINDRICAL_SURFACE ( 'NONE', #19756, 0.5000000000000004441 ) ;
#35768=DIRECTION ( 'NONE',  ( 0.7032331762533998720, -0.07391278520356875381, -0.7071067811865517916 ) ) ;
#35769=VERTEX_POINT ( 'NONE', #6761 ) ;
#35771=AXIS2_PLACEMENT_3D ( 'NONE', #26247, #38645, #10819 ) ;
#35774=AXIS2_PLACEMENT_3D ( 'NONE', #21355, #15256, #24398 ) ;
#35775=CARTESIAN_POINT ( 'NONE',  ( -9.705584749708384251, 11.06314620770957013, 7.221809905720049549 ) ) ;
#35776=ORIENTED_EDGE ( 'NONE', *, *, #33112, .F. ) ;
#35779=LINE ( 'NONE', #20342, #24347 ) ;
#35782=DIRECTION ( 'NONE',  ( 0.000000000000000000, 0.000000000000000000, -1.000000000000000000 ) ) ;
#35783=ORIENTED_EDGE ( 'NONE', *, *, #6545, .F. ) ;
#35786=DIRECTION ( 'NONE',  ( 0.6037757019622738142, 0.000000000000000000, -0.7971542521494591194 ) ) ;
#35788=EDGE_LOOP ( 'NONE', ( #2333, #31520, #531, #39463, #465, #32643, #35582 ) ) ;
#35790=DIRECTION ( 'NONE',  ( -0.000000000000000000, 0.000000000000000000, 1.000000000000000000 ) ) ;
#35791=ORIENTED_EDGE ( 'NONE', *, *, #24166, .T. ) ;
#35802=VECTOR ( 'NONE', #11763, 999.9999999999998863 ) ;
#35805=CARTESIAN_POINT ( 'NONE',  ( -11.44473057578096764, 31.45924896672619298, 7.000000000000000000 ) ) ;
#35807=AXIS2_PLACEMENT_3D ( 'NONE', #3643, #15841, #28423 ) ;
#35809=DIRECTION ( 'NONE',  ( -0.000000000000000000, -0.000000000000000000, -1.000000000000000000 ) ) ;
#35810=CARTESIAN_POINT ( 'NONE',  ( -13.05736835487441994, 16.11602540378456538, 10.49999999999999822 ) ) ;
#35811=DIRECTION ( 'NONE',  ( 0.000000000000000000, -0.000000000000000000, 1.000000000000000000 ) ) ;
#35817=CARTESIAN_POINT ( 'NONE',  ( 4.244284213106223724, 8.112413639933444998, 7.203056206335832989 ) ) ;
#35819=VERTEX_POINT ( 'NONE', #4326 ) ;
#35826=ORIENTED_EDGE ( 'NONE', *, *, #12614, .F. ) ;
#35829=LINE ( 'NONE', #29531, #11862 ) ;
#35839=ADVANCED_FACE ( 'NONE', ( #16123 ), #19419, .T. ) ;
#35843=CARTESIAN_POINT ( 'NONE',  ( 7.126083911573381613, 10.99048532364570008, 9.500000000000000000 ) ) ;
#35846=ADVANCED_FACE ( 'NONE', ( #35014 ), #27623, .T. ) ;
#35847=CARTESIAN_POINT ( 'NONE',  ( -4.727507481117091181, 31.88885898370948269, 10.50000000000000000 ) ) ;
#35850=LINE ( 'NONE', #17176, #14643 ) ;
#35851=ORIENTED_EDGE ( 'NONE', *, *, #35571, .F. ) ;
#35853=CARTESIAN_POINT ( 'NONE',  ( 2.525645716490525494, 8.212903943950921715, 11.00000000000000000 ) ) ;
#35856=CARTESIAN_POINT ( 'NONE',  ( 10.44103466624280685, 32.57396620494213124, 7.000000000000000000 ) ) ;
#35857=FACE_OUTER_BOUND ( 'NONE', #9743, .T. ) ;
#35859=CIRCLE ( 'NONE', #37794, 15.00000000000000000 ) ;
#35860=CARTESIAN_POINT ( 'NONE',  ( 13.47830981910552062, 21.58612669357076896, 10.00000000000000000 ) ) ;
#35864=ADVANCED_FACE ( 'NONE', ( #26668 ), #6095, .T. ) ;
#35867=ADVANCED_FACE ( 'NONE', ( #30123 ), #23821, .T. ) ;
#35870=ORIENTED_EDGE ( 'NONE', *, *, #37409, .F. ) ;
#35871=DIRECTION ( 'NONE',  ( 0.5877852522924690293, -0.8090169943749504489, 0.000000000000000000 ) ) ;
#35877=VECTOR ( 'NONE', #846, 1000.000000000000114 ) ;
#35881=ORIENTED_EDGE ( 'NONE', *, *, #797, .T. ) ;
#35884=CARTESIAN_POINT ( 'NONE',  ( -12.51665927450813953, 14.23331522619103851, 7.382773698552465014 ) ) ;
#35886=ORIENTED_EDGE ( 'NONE', *, *, #4282, .T. ) ;
#35888=CIRCLE ( 'NONE', #37185, 0.5000000000000004441 ) ;
#35892=CARTESIAN_POINT ( 'NONE',  ( -5.362728154696096539, 13.41753630677062148, 10.50000000000000000 ) ) ;
#35894=CARTESIAN_POINT ( 'NONE',  ( -8.910254037844422825, 17.93301270189230223, 10.49999999999999822 ) ) ;
#35897=CARTESIAN_POINT ( 'NONE',  ( 7.133890061153794093, 30.26901619224539886, 10.50000000000000000 ) ) ;
#35898=ORIENTED_EDGE ( 'NONE', *, *, #17514, .F. ) ;
#35901=VECTOR ( 'NONE', #1221, 1000.000000000000000 ) ;
#35902=CARTESIAN_POINT ( 'NONE',  ( 6.856644039074955899, 35.52575270032630073, 10.49999999999999822 ) ) ;
#35906=DIRECTION ( 'NONE',  ( 0.2079116908177533751, -0.9781476007338069101, 0.000000000000000000 ) ) ;
#35907=LINE ( 'NONE', #5225, #40037 ) ;
#35912=CARTESIAN_POINT ( 'NONE',  ( -12.74038105676665289, 14.56698729810790027, 10.49999999999999822 ) ) ;
#35913=ORIENTED_EDGE ( 'NONE', *, *, #39393, .F. ) ;
#35915=DIRECTION ( 'NONE',  ( -0.9135454576426046414, -0.4067366430757919371, 0.000000000000000000 ) ) ;
#35923=EDGE_CURVE ( 'NONE', #10078, #34816, #39714, .T. ) ;
#35930=DIRECTION ( 'NONE',  ( -0.000000000000000000, -0.000000000000000000, -1.000000000000000000 ) ) ;
#35934=AXIS2_PLACEMENT_3D ( 'NONE', #30852, #8715, #39386 ) ;
#35935=LINE ( 'NONE', #8092, #18320 ) ;
#35936=ORIENTED_EDGE ( 'NONE', *, *, #14597, .T. ) ;
#35937=DIRECTION ( 'NONE',  ( 0.000000000000000000, -0.6729908358753734499, 0.7396508195275431907 ) ) ;
#35938=CYLINDRICAL_SURFACE ( 'NONE', #16108, 0.4999999999999988898 ) ;
#35939=EDGE_LOOP ( 'NONE', ( #24741, #18354, #37341 ) ) ;
#35941=EDGE_CURVE ( 'NONE', #24748, #19049, #23069, .T. ) ;
#35946=ORIENTED_EDGE ( 'NONE', *, *, #36882, .F. ) ;
#35949=ORIENTED_EDGE ( 'NONE', *, *, #16305, .T. ) ;
#35951=LINE ( 'NONE', #8106, #10474 ) ;
#35953=EDGE_CURVE ( 'NONE', #34728, #23552, #1487, .T. ) ;
#35963=EDGE_LOOP ( 'NONE', ( #20352, #16564, #38810, #19722 ) ) ;
#35965=LINE ( 'NONE', #17487, #5850 ) ;
#35969=EDGE_CURVE ( 'NONE', #1935, #24077, #8709, .T. ) ;
#35970=CARTESIAN_POINT ( 'NONE',  ( -9.004335565032201671, 10.95724613078633425, 11.00000000000000000 ) ) ;
#35976=CARTESIAN_POINT ( 'NONE',  ( -9.451751316756979548, 10.85217908230550599, 7.439083675050419231 ) ) ;
#35977=ORIENTED_EDGE ( 'NONE', *, *, #789, .F. ) ;
#35980=FACE_OUTER_BOUND ( 'NONE', #19475, .T. ) ;
#35982=AXIS2_PLACEMENT_3D ( 'NONE', #23971, #20128, #32725 ) ;
#35984=CARTESIAN_POINT ( 'NONE',  ( -13.48130249190472796, 27.93180293473203690, 7.499999999999993783 ) ) ;
#35985=ORIENTED_EDGE ( 'NONE', *, *, #31965, .T. ) ;
#35987=CARTESIAN_POINT ( 'NONE',  ( 9.892954722048902028, 20.95745441963929068, 10.00000000000000000 ) ) ;
#35988=CARTESIAN_POINT ( 'NONE',  ( -14.09933648065464062, 26.02968990214173317, 10.50000000000000533 ) ) ;
#35989=CARTESIAN_POINT ( 'NONE',  ( -2.036571916123811388, 8.108948098542073879, 10.49999999999999822 ) ) ;
#35990=ORIENTED_EDGE ( 'NONE', *, *, #6636, .F. ) ;
#35992=CARTESIAN_POINT ( 'NONE',  ( -5.440908595777636414, 35.94977745735568675, 10.99999999999999289 ) ) ;
#35993=EDGE_CURVE ( 'NONE', #29721, #33995, #8203, .T. ) ;
#35994=ORIENTED_EDGE ( 'NONE', *, *, #20742, .T. ) ;
#35996=VECTOR ( 'NONE', #28647, 1000.000000000000227 ) ;
#35999=EDGE_LOOP ( 'NONE', ( #4542, #26469, #20323 ) ) ;
#36004=CARTESIAN_POINT ( 'NONE',  ( -3.596545519285825776, 7.984450832230675310, 10.76099332938163755 ) ) ;
#36005=ORIENTED_EDGE ( 'NONE', *, *, #37701, .T. ) ;
#36006=DIRECTION ( 'NONE',  ( 0.000000000000000000, 0.000000000000000000, 1.000000000000000000 ) ) ;
#36007=DIRECTION ( 'NONE',  ( -1.000000000000000000, 0.000000000000000000, 0.000000000000000000 ) ) ;
#36010=DIRECTION ( 'NONE',  ( -0.000000000000000000, -0.000000000000000000, -1.000000000000000000 ) ) ;
#36013=CARTESIAN_POINT ( 'NONE',  ( -5.440908595777636414, 35.94977745735568675, 7.000000000000000000 ) ) ;
#36014=VECTOR ( 'NONE', #4577, 999.9999999999998863 ) ;
#36015=CARTESIAN_POINT ( 'NONE',  ( -13.13451774850164355, 16.06441397984658792, 10.49999999999999822 ) ) ;
#36016=LINE ( 'NONE', #3970, #7726 ) ;
#36017=ORIENTED_EDGE ( 'NONE', *, *, #25880, .T. ) ;
#36019=VERTEX_POINT ( 'NONE', #15078 ) ;
#36023=CARTESIAN_POINT ( 'NONE',  ( -14.09933648065463707, 26.02968990214174028, 10.49999999999999822 ) ) ;
#36025=ORIENTED_EDGE ( 'NONE', *, *, #15393, .F. ) ;
#36029=CARTESIAN_POINT ( 'NONE',  ( -12.99377146717201015, 26.19620116591435632, 9.500000000000000000 ) ) ;
#36031=DIRECTION ( 'NONE',  ( -0.000000000000000000, -0.000000000000000000, -1.000000000000000000 ) ) ;
#36035=DIRECTION ( 'NONE',  ( 0.000000000000000000, 0.000000000000000000, 1.000000000000000000 ) ) ;
#36038=CARTESIAN_POINT ( 'NONE',  ( -13.63581098909220479, 27.45627467658446008, 7.000000000000000000 ) ) ;
#36042=CIRCLE ( 'NONE', #18518, 1.000000000000003553 ) ;
#36045=ORIENTED_EDGE ( 'NONE', *, *, #8115, .T. ) ;
#36050=AXIS2_PLACEMENT_3D ( 'NONE', #37499, #22050, #31397 ) ;
#36053=CARTESIAN_POINT ( 'NONE',  ( -10.44103466624267185, 32.57396620494226624, 9.000000000000001776 ) ) ;
#36054=DIRECTION ( 'NONE',  ( 0.000000000000000000, 0.000000000000000000, -1.000000000000000000 ) ) ;
#36055=DIRECTION ( 'NONE',  ( -0.9945218953682745111, -0.1045284632676425907, 0.000000000000000000 ) ) ;
#36059=CARTESIAN_POINT ( 'NONE',  ( 3.914034194965611668, 30.06176806842419680, 9.000000000000001776 ) ) ;
#36068=EDGE_CURVE ( 'NONE', #490, #27538, #32458, .T. ) ;
#36069=LINE ( 'NONE', #20434, #30193 ) ;
#36074=VECTOR ( 'NONE', #28866, 1000.000000000000000 ) ;
#36076=CARTESIAN_POINT ( 'NONE',  ( -9.997483185316569987, 21.95197631500770896, 10.49999999999999467 ) ) ;
#36079=AXIS2_PLACEMENT_3D ( 'NONE', #3192, #21868, #19025 ) ;
#36082=CARTESIAN_POINT ( 'NONE',  ( 5.027400250556079975, 36.23526740290145653, 10.49999999999999822 ) ) ;
#36084=EDGE_CURVE ( 'NONE', #32234, #26241, #26993, .T. ) ;
#36085=ORIENTED_EDGE ( 'NONE', *, *, #18262, .F. ) ;
#36088=CARTESIAN_POINT ( 'NONE',  ( 6.282361020112163352, 14.70372268239673375, 10.50000000000000000 ) ) ;
#36090=EDGE_CURVE ( 'NONE', #22206, #37186, #37215, .T. ) ;
#36092=EDGE_LOOP ( 'NONE', ( #21502, #23476, #14231, #9360, #14564 ) ) ;
#36095=CARTESIAN_POINT ( 'NONE',  ( 14.47283171447379146, 21.48159823030311344, 7.000000000000000000 ) ) ;
#36097=DIRECTION ( 'NONE',  ( -0.1045284632676437703, 0.9945218953682745111, 0.000000000000000000 ) ) ;
#36098=DIRECTION ( 'NONE',  ( -0.000000000000000000, -0.000000000000000000, 1.000000000000000000 ) ) ;
#36099=LINE ( 'NONE', #14760, #10296 ) ;
#36103=DIRECTION ( 'NONE',  ( -0.000000000000000000, -0.000000000000000000, -1.000000000000000000 ) ) ;
#36104=VECTOR ( 'NONE', #36175, 1000.000000000000114 ) ;
#36105=AXIS2_PLACEMENT_3D ( 'NONE', #27128, #11493, #32837 ) ;
#36107=ORIENTED_EDGE ( 'NONE', *, *, #22736, .F. ) ;
#36111=DIRECTION ( 'NONE',  ( -0.000000000000000000, -0.000000000000000000, -1.000000000000000000 ) ) ;
#36112=CARTESIAN_POINT ( 'NONE',  ( 4.003810537522394242, 8.420815593655317954, 10.49999999999999822 ) ) ;
#36113=DIRECTION ( 'NONE',  ( -1.000000000000000000, 0.000000000000000000, 0.000000000000000000 ) ) ;
#36114=DIRECTION ( 'NONE',  ( 1.000000000000000000, 0.000000000000000000, 0.000000000000000000 ) ) ;
#36124=DIRECTION ( 'NONE',  ( -0.9781476007338041345, 0.2079116908177663092, 0.000000000000000000 ) ) ;
#36125=ADVANCED_FACE ( 'NONE', ( #15676 ), #2856, .T. ) ;
#36132=ORIENTED_EDGE ( 'NONE', *, *, #1183, .F. ) ;
#36135=VECTOR ( 'NONE', #33054, 1000.000000000000114 ) ;
#36136=VECTOR ( 'NONE', #7075, 1000.000000000000000 ) ;
#36137=CARTESIAN_POINT ( 'NONE',  ( 5.204598533297671636, 36.56827286999722304, 7.339470489435498735 ) ) ;
#36139=DIRECTION ( 'NONE',  ( 0.1470157664651934870, -0.6916548014802242905, -0.7071067811865497932 ) ) ;
#36140=CARTESIAN_POINT ( 'NONE',  ( 19.15807744002891155, 8.842452143891316396, 7.500000000000000000 ) ) ;
#36143=ORIENTED_EDGE ( 'NONE', *, *, #7253, .F. ) ;
#36145=ORIENTED_EDGE ( 'NONE', *, *, #19562, .T. ) ;
#36146=CARTESIAN_POINT ( 'NONE',  ( -11.44134295108998955, 15.31698729810788961, 9.500000000000000000 ) ) ;
#36147=ORIENTED_EDGE ( 'NONE', *, *, #8513, .T. ) ;
#36149=FACE_OUTER_BOUND ( 'NONE', #37671, .T. ) ;
#36151=CARTESIAN_POINT ( 'NONE',  ( 0.4999999999999990563, 31.00000000000000355, 7.000000000000000000 ) ) ;
#36155=CARTESIAN_POINT ( 'NONE',  ( -2.552861293176900137, 8.084864722426296169, 10.99999999999999822 ) ) ;
#36156=CARTESIAN_POINT ( 'NONE',  ( 11.70245575391219006, 4.690003899809237708, 9.500000000000000000 ) ) ;
#36161=ORIENTED_EDGE ( 'NONE', *, *, #35340, .T. ) ;
#36167=CIRCLE ( 'NONE', #8937, 1.000000000000004441 ) ;
#36168=CARTESIAN_POINT ( 'NONE',  ( -14.47283171447380035, 21.48159823030330884, 7.500000000000004441 ) ) ;
#36170=CIRCLE ( 'NONE', #14096, 0.5000000000000004441 ) ;
#36174=EDGE_CURVE ( 'NONE', #6531, #27384, #24023, .T. ) ;
#36175=DIRECTION ( 'NONE',  ( 0.6691306063588570163, -0.7431448254773952433, 0.000000000000000000 ) ) ;
#36176=ORIENTED_EDGE ( 'NONE', *, *, #21242, .T. ) ;
#36179=DIRECTION ( 'NONE',  ( -0.7431448254773850293, 0.6691306063588685626, 0.000000000000000000 ) ) ;
#36180=DIRECTION ( 'NONE',  ( 0.3090169943749572767, 0.9510565162951503115, -0.000000000000000000 ) ) ;
#36182=DIRECTION ( 'NONE',  ( -0.4999999999999921174, 0.8660254037844431485, 0.000000000000000000 ) ) ;
#36185=CARTESIAN_POINT ( 'NONE',  ( -5.400683141673551013, 15.91724817395922997, 7.000000000000000000 ) ) ;
#36186=DIRECTION ( 'NONE',  ( -0.8660254037844431485, -0.4999999999999921174, 0.000000000000000000 ) ) ;
#36190=ADVANCED_BREP_SHAPE_REPRESENTATION ( '', ( #8155, #24238 ), #11913 ) ;
#36191=CARTESIAN_POINT ( 'NONE',  ( 14.09933648065468503, 26.02968990214155198, 7.500000000000000888 ) ) ;
#36192=ORIENTED_EDGE ( 'NONE', *, *, #29090, .F. ) ;
#36194=TOROIDAL_SURFACE ( 'NONE', #22568, 1.000000000000000000, 0.5000000000000000000 ) ;
#36199=EDGE_CURVE ( 'NONE', #15690, #17187, #8163, .T. ) ;
#36203=LINE ( 'NONE', #29894, #39011 ) ;
#36204=EDGE_CURVE ( 'NONE', #37355, #27267, #9785, .T. ) ;
#36206=VECTOR ( 'NONE', #24684, 1000.000000000000000 ) ;
#36208=ORIENTED_EDGE ( 'NONE', *, *, #24142, .T. ) ;
#36209=CARTESIAN_POINT ( 'NONE',  ( -7.766013557953293400, 28.81973365084998306, 10.49999999999999822 ) ) ;
#36210=CARTESIAN_POINT ( 'NONE',  ( -13.48130249190472796, 27.93180293473203690, 11.00000000000000000 ) ) ;
#36212=CARTESIAN_POINT ( 'NONE',  ( -8.118377661053489902, 10.47536095541709322, 7.500000000000000888 ) ) ;
#36216=DIRECTION ( 'NONE',  ( 0.9135454576426005335, -0.4067366430758008744, 0.000000000000000000 ) ) ;
#36217=CARTESIAN_POINT ( 'NONE',  ( -3.813962023474485541, 32.29559562678526419, 11.00000000000000000 ) ) ;
#36219=EDGE_CURVE ( 'NONE', #36670, #20763, #19123, .T. ) ;
#36222=EDGE_CURVE ( 'NONE', #6988, #37631, #22358, .T. ) ;
#36223=VERTEX_POINT ( 'NONE', #15879 ) ;
#36226=ADVANCED_FACE ( 'NONE', ( #19727 ), #25218, .T. ) ;
#36227=CARTESIAN_POINT ( 'NONE',  ( -2.199596516246109523, 8.143600047011682719, 10.66666666666666607 ) ) ;
#36231=ORIENTED_EDGE ( 'NONE', *, *, #5088, .F. ) ;
#36237=VECTOR ( 'NONE', #38577, 1000.000000000000114 ) ;
#36238=ORIENTED_EDGE ( 'NONE', *, *, #10628, .T. ) ;
#36242=DIRECTION ( 'NONE',  ( -0.000000000000000000, -0.000000000000000000, -1.000000000000000000 ) ) ;
#36243=EDGE_LOOP ( 'NONE', ( #3020, #12870, #805 ) ) ;
#36245=CARTESIAN_POINT ( 'NONE',  ( -7.741055489194995864, 10.14404956260399615, 10.49999999999999822 ) ) ;
#36251=VERTEX_POINT ( 'NONE', #3483 ) ;
#36253=LINE ( 'NONE', #37040, #30059 ) ;
#36254=EDGE_CURVE ( 'NONE', #21244, #27921, #15944, .T. ) ;
#36255=DIRECTION ( 'NONE',  ( 0.1045284632676437703, -0.9945218953682745111, -0.000000000000000000 ) ) ;
#36256=AXIS2_PLACEMENT_3D ( 'NONE', #13566, #22906, #4018 ) ;
#36258=VECTOR ( 'NONE', #39492, 1000.000000000000000 ) ;
#36259=CARTESIAN_POINT ( 'NONE',  ( -2.165907168841142205, 7.657055764658191599, 7.339470489435488965 ) ) ;
#36260=CARTESIAN_POINT ( 'NONE',  ( 6.535904741238498517, 35.95058573176943639, 10.76099332938163755 ) ) ;
#36262=EDGE_LOOP ( 'NONE', ( #33342, #1868, #30088 ) ) ;
#36264=DIRECTION ( 'NONE',  ( 0.6691306063588671194, 0.7431448254773861395, 0.000000000000000000 ) ) ;
#36265=CARTESIAN_POINT ( 'NONE',  ( 8.007761790012084546, 9.776959832083274904, 11.00000000000000000 ) ) ;
#36267=CYLINDRICAL_SURFACE ( 'NONE', #18390, 0.5000000000000004441 ) ;
#36268=CARTESIAN_POINT ( 'NONE',  ( -14.36203778474861181, 19.98498072221388000, 10.49999999999999822 ) ) ;
#36271=ORIENTED_EDGE ( 'NONE', *, *, #24947, .F. ) ;
#36277=EDGE_LOOP ( 'NONE', ( #26650, #35977 ) ) ;
#36278=DIRECTION ( 'NONE',  ( 0.8090169943749503378, 0.5877852522924691403, 0.000000000000000000 ) ) ;
#36279=ORIENTED_EDGE ( 'NONE', *, *, #18557, .F. ) ;
#36285=CIRCLE ( 'NONE', #31083, 0.5000000000000004441 ) ;
#36294=VECTOR ( 'NONE', #16304, 1000.000000000000000 ) ;
#36295=EDGE_LOOP ( 'NONE', ( #17157, #16436, #1918, #3777 ) ) ;
#36298=DIRECTION ( 'NONE',  ( 0.9945218953682730678, -0.1045284632676564962, 0.000000000000000000 ) ) ;
#36304=ORIENTED_EDGE ( 'NONE', *, *, #33845, .F. ) ;
#36306=CARTESIAN_POINT ( 'NONE',  ( 6.843305518951320998, 35.42677428760913472, 10.49999999999999822 ) ) ;
#36307=ORIENTED_EDGE ( 'NONE', *, *, #9937, .F. ) ;
#36311=EDGE_CURVE ( 'NONE', #13704, #21433, #1713, .T. ) ;
#36312=DIRECTION ( 'NONE',  ( -0.8090169943749505599, -0.5877852522924689183, 0.000000000000000000 ) ) ;
#36314=CARTESIAN_POINT ( 'NONE',  ( 9.356056665764066693, 26.06569820189703535, 10.00000000000000000 ) ) ;
#36315=FACE_OUTER_BOUND ( 'NONE', #23014, .T. ) ;
#36317=CARTESIAN_POINT ( 'NONE',  ( -10.10646936306323518, 32.94553861768095970, 7.500000000000004441 ) ) ;
#36320=DIRECTION ( 'NONE',  ( 0.4067366430757913820, -0.9135454576426049744, -7.055756032835740798E-16 ) ) ;
#36331=FACE_OUTER_BOUND ( 'NONE', #19902, .T. ) ;
#36333=ORIENTED_EDGE ( 'NONE', *, *, #37077, .F. ) ;
#36336=AXIS2_PLACEMENT_3D ( 'NONE', #6359, #37052, #7515 ) ;
#36338=ORIENTED_EDGE ( 'NONE', *, *, #18087, .F. ) ;
#36339=CARTESIAN_POINT ( 'NONE',  ( -5.034171952701854025, 35.03623199971307400, 9.500000000000000000 ) ) ;
#36340=CARTESIAN_POINT ( 'NONE',  ( 9.221287281574507944, 10.65863771052197784, 10.49999999999999822 ) ) ;
#36341=VECTOR ( 'NONE', #1369, 1000.000000000000227 ) ;
#36343=B_SPLINE_CURVE_WITH_KNOTS ( 'NONE', 3,
 ( #8341, #33135, #35976, #26218, #23379, #35775 ),
 .UNSPECIFIED., .F., .F.,
 ( 4, 2, 4 ),
 ( 0.000000000000000000, 0.0002970590326188848234, 0.0005941180652377696467 ),
 .UNSPECIFIED. ) ;
#36346=EDGE_LOOP ( 'NONE', ( #11037, #22577, #17562, #19242 ) ) ;
#36347=CARTESIAN_POINT ( 'NONE',  ( 11.44134295108989363, 15.31698729810773152, 9.500000000000000000 ) ) ;
#36349=FACE_OUTER_BOUND ( 'NONE', #31579, .T. ) ;
#36350=LINE ( 'NONE', #8515, #1405 ) ;
#36352=VERTEX_POINT ( 'NONE', #7122 ) ;
#36353=EDGE_CURVE ( 'NONE', #23354, #11801, #18926, .T. ) ;
#36355=LINE ( 'NONE', #30860, #27576 ) ;
#36356=CARTESIAN_POINT ( 'NONE',  ( 11.48173768534035943, 32.16538668264416145, 10.50000000000000000 ) ) ;
#36357=EDGE_CURVE ( 'NONE', #12690, #3600, #10383, .T. ) ;
#36358=DIRECTION ( 'NONE',  ( 0.7071067811865479058, 0.000000000000000000, -0.7071067811865472397 ) ) ;
#36361=ORIENTED_EDGE ( 'NONE', *, *, #28655, .F. ) ;
#36367=AXIS2_PLACEMENT_3D ( 'NONE', #35847, #8009, #5366 ) ;
#36372=EDGE_CURVE ( 'NONE', #36487, #38004, #26013, .T. ) ;
#36373=CARTESIAN_POINT ( 'NONE',  ( 0.5000000000000000000, 37.00000000000000711, 7.000000000000000000 ) ) ;
#36378=DIRECTION ( 'NONE',  ( 1.000000000000000000, 0.000000000000000000, 0.000000000000000000 ) ) ;
#36379=CARTESIAN_POINT ( 'NONE',  ( -12.69365875748883710, 14.48606190191228116, 10.49999999999999822 ) ) ;
#36381=FACE_OUTER_BOUND ( 'NONE', #33249, .T. ) ;
#36382=ORIENTED_EDGE ( 'NONE', *, *, #39444, .F. ) ;
#36386=DIRECTION ( 'NONE',  ( 0.5000000000000039968, 0.8660254037844363761, 0.000000000000000000 ) ) ;
#36387=ORIENTED_EDGE ( 'NONE', *, *, #37220, .T. ) ;
#36390=ORIENTED_EDGE ( 'NONE', *, *, #10041, .F. ) ;
#36393=ORIENTED_EDGE ( 'NONE', *, *, #29011, .T. ) ;
#36395=CONICAL_SURFACE ( 'NONE', #33797, 1.000000000000004441, 0.7853981633974522758 ) ;
#36397=DIRECTION ( 'NONE',  ( -0.7071067811865511255, 0.000000000000000000, -0.7071067811865440200 ) ) ;
#36398=ADVANCED_FACE ( 'NONE', ( #38412 ), #38032, .T. ) ;
#36401=ORIENTED_EDGE ( 'NONE', *, *, #10758, .T. ) ;
#36402=CARTESIAN_POINT ( 'NONE',  ( 10.10646936306337729, 32.94553861768082470, 10.49999999999999645 ) ) ;
#36403=FACE_OUTER_BOUND ( 'NONE', #8496, .T. ) ;
#36405=DIRECTION ( 'NONE',  ( 0.000000000000000000, 0.000000000000000000, -1.000000000000000000 ) ) ;
#36407=VECTOR ( 'NONE', #27893, 1000.000000000000000 ) ;
#36410=CARTESIAN_POINT ( 'NONE',  ( 5.473344025737210572, 14.11593743010426394, 10.49999999999999822 ) ) ;
#36414=ORIENTED_EDGE ( 'NONE', *, *, #14721, .T. ) ;
#36417=CARTESIAN_POINT ( 'NONE',  ( -9.331903152615899089, 11.35703883385581037, 11.00000000000000000 ) ) ;
#36419=VERTEX_POINT ( 'NONE', #26420 ) ;
#36426=DIRECTION ( 'NONE',  ( 0.000000000000000000, 0.000000000000000000, 1.000000000000000000 ) ) ;
#36427=EDGE_CURVE ( 'NONE', #31487, #6543, #1852, .T. ) ;
#36428=ORIENTED_EDGE ( 'NONE', *, *, #21931, .F. ) ;
#36431=CARTESIAN_POINT ( 'NONE',  ( 14.96930490892014554, 21.54088032874971859, 7.500000000000010658 ) ) ;
#36432=ORIENTED_EDGE ( 'NONE', *, *, #36703, .T. ) ;
#36436=ORIENTED_EDGE ( 'NONE', *, *, #4837, .T. ) ;
#36440=CIRCLE ( 'NONE', #18915, 1.000000000000000444 ) ;
#36442=AXIS2_PLACEMENT_3D ( 'NONE', #22738, #35143, #13802 ) ;
#36443=VERTEX_POINT ( 'NONE', #26823 ) ;
#36445=DIRECTION ( 'NONE',  ( 0.000000000000000000, 0.000000000000000000, -1.000000000000000000 ) ) ;
#36446=ADVANCED_FACE ( 'NONE', ( #4887 ), #38815, .T. ) ;
#36447=CARTESIAN_POINT ( 'NONE',  ( -11.94134295108998423, 16.18301270189233421, 9.500000000000000000 ) ) ;
#36449=EDGE_CURVE ( 'NONE', #37593, #19542, #36343, .T. ) ;
#36450=AXIS2_PLACEMENT_3D ( 'NONE', #12190, #5489, #6 ) ;
#36451=FACE_OUTER_BOUND ( 'NONE', #29673, .T. ) ;
#36452=EDGE_CURVE ( 'NONE', #39537, #17600, #31539, .T. ) ;
#36453=DIRECTION ( 'NONE',  ( 0.000000000000000000, 0.000000000000000000, 1.000000000000000000 ) ) ;
#36455=VERTEX_POINT ( 'NONE', #23775 ) ;
#36460=LINE ( 'NONE', #14725, #4108 ) ;
#36466=LINE ( 'NONE', #11686, #31483 ) ;
#36468=ORIENTED_EDGE ( 'NONE', *, *, #31754, .T. ) ;
#36469=CARTESIAN_POINT ( 'NONE',  ( 5.767236651883444587, 13.71142893291679243, 10.50000000000000000 ) ) ;
#36470=VERTEX_POINT ( 'NONE', #20539 ) ;
#36472=DIRECTION ( 'NONE',  ( 0.000000000000000000, 0.000000000000000000, 1.000000000000000000 ) ) ;
#36475=CARTESIAN_POINT ( 'NONE',  ( 9.221287281574507944, 10.65863771052197784, 10.49999999999999822 ) ) ;
#36476=EDGE_CURVE ( 'NONE', #21371, #18984, #13382, .T. ) ;
#36481=ORIENTED_EDGE ( 'NONE', *, *, #25437, .F. ) ;
#36483=DIRECTION ( 'NONE',  ( 0.9876883405951372152, -0.1564344650402341719, 0.000000000000000000 ) ) ;
#36484=VECTOR ( 'NONE', #8703, 999.9999999999998863 ) ;
#36486=CARTESIAN_POINT ( 'NONE',  ( 4.096822963000107620, 8.035697679810645866, 7.000000000000000000 ) ) ;
#36487=VERTEX_POINT ( 'NONE', #35370 ) ;
#36490=AXIS2_PLACEMENT_3D ( 'NONE', #4032, #25569, #12977 ) ;
#36491=DIRECTION ( 'NONE',  ( 0.4067366430758009854, 0.9135454576426005335, 0.000000000000000000 ) ) ;
#36493=VECTOR ( 'NONE', #36445, 1000.000000000000000 ) ;
#36495=ADVANCED_FACE ( 'NONE', ( #29273 ), #17925, .T. ) ;
#36497=CIRCLE ( 'NONE', #1463, 0.5000000000000004441 ) ;
#36498=EDGE_CURVE ( 'NONE', #1779, #10635, #14428, .T. ) ;
#36501=CARTESIAN_POINT ( 'NONE',  ( 6.713764256189890922, 35.89999254728742528, 10.49999999999999822 ) ) ;
#36502=DIRECTION ( 'NONE',  ( -1.000000000000000000, 0.000000000000000000, 0.000000000000000000 ) ) ;
#36506=DIRECTION ( 'NONE',  ( -0.3090169943749573878, -0.9510565162951503115, 0.000000000000000000 ) ) ;
#36507=DIRECTION ( 'NONE',  ( -0.000000000000000000, -0.000000000000000000, -1.000000000000000000 ) ) ;
#36508=DIRECTION ( 'NONE',  ( 0.9510565162951543083, 0.3090169943749450088, 0.000000000000000000 ) ) ;
#36511=DIRECTION ( 'NONE',  ( 1.000000000000000000, 0.000000000000000000, 0.000000000000000000 ) ) ;
#36512=ORIENTED_EDGE ( 'NONE', *, *, #38029, .T. ) ;
#36513=VECTOR ( 'NONE', #37626, 1000.000000000000227 ) ;
#36516=DIRECTION ( 'NONE',  ( 0.1045284632676437842, -0.9945218953682744001, 0.000000000000000000 ) ) ;
#36521=CARTESIAN_POINT ( 'NONE',  ( 0.5000000000000035527, 32.50000000000000000, 10.50000000000000178 ) ) ;
#36522=DIRECTION ( 'NONE',  ( -0.000000000000000000, -0.000000000000000000, -1.000000000000000000 ) ) ;
#36527=DIRECTION ( 'NONE',  ( 0.07391278520356295290, -0.7032331762534080877, -0.7071067811865440200 ) ) ;
#36528=ADVANCED_FACE ( 'NONE', ( #14229 ), #23172, .F. ) ;
#36530=ORIENTED_EDGE ( 'NONE', *, *, #5088, .T. ) ;
#36534=FACE_OUTER_BOUND ( 'NONE', #37189, .T. ) ;
#36542=DIRECTION ( 'NONE',  ( 1.000000000000000000, 0.000000000000000000, 0.000000000000000000 ) ) ;
#36543=ORIENTED_EDGE ( 'NONE', *, *, #1303, .T. ) ;
#36545=CYLINDRICAL_SURFACE ( 'NONE', #32561, 0.5000000000000004441 ) ;
#36547=FACE_OUTER_BOUND ( 'NONE', #23874, .T. ) ;
#36548=ORIENTED_EDGE ( 'NONE', *, *, #34355, .T. ) ;
#36551=DIRECTION ( 'NONE',  ( -0.000000000000000000, -0.000000000000000000, -1.000000000000000000 ) ) ;
#36552=CARTESIAN_POINT ( 'NONE',  ( 13.37378135583786332, 20.59160479820249634, 9.500000000000000000 ) ) ;
#36555=AXIS2_PLACEMENT_3D ( 'NONE', #178, #383, #25156 ) ;
#36557=ORIENTED_EDGE ( 'NONE', *, *, #39560, .F. ) ;
#36560=CARTESIAN_POINT ( 'NONE',  ( 14.52509594610761923, 21.97885917798724975, 10.50000000000000355 ) ) ;
#36562=CARTESIAN_POINT ( 'NONE',  ( 12.30736835487432579, 14.81698729810772619, 7.499999999999997335 ) ) ;
#36565=VECTOR ( 'NONE', #15209, 1000.000000000000114 ) ;
#36568=EDGE_CURVE ( 'NONE', #35341, #28707, #2052, .T. ) ;
#36569=CARTESIAN_POINT ( 'NONE',  ( 10.10646936306337729, 32.94553861768082470, 7.499999999999997335 ) ) ;
#36570=VERTEX_POINT ( 'NONE', #17498 ) ;
#36571=VERTEX_POINT ( 'NONE', #20743 ) ;
#36573=CARTESIAN_POINT ( 'NONE',  ( -13.47830981910551529, 21.58612669357095371, 7.000000000000000000 ) ) ;
#36574=DIRECTION ( 'NONE',  ( 0.9135454576426005335, -0.4067366430758009299, 0.000000000000000000 ) ) ;
#36575=VECTOR ( 'NONE', #39246, 1000.000000000000000 ) ;
#36576=LINE ( 'NONE', #3250, #29946 ) ;
#36577=VERTEX_POINT ( 'NONE', #16685 ) ;
#36579=ADVANCED_FACE ( 'NONE', ( #1245 ), #13626, .T. ) ;
#36580=DIRECTION ( 'NONE',  ( 1.000000000000000000, 0.000000000000000000, 0.000000000000000000 ) ) ;
#36581=CARTESIAN_POINT ( 'NONE',  ( -2.525645716490712012, 8.212903943950955465, 10.99999999999999289 ) ) ;
#36582=ADVANCED_FACE ( 'NONE', ( #39409 ), #24375, .F. ) ;
#36583=ORIENTED_EDGE ( 'NONE', *, *, #13464, .T. ) ;
#36586=ORIENTED_EDGE ( 'NONE', *, *, #37807, .F. ) ;
#36590=ORIENTED_EDGE ( 'NONE', *, *, #23586, .F. ) ;
#36593=CARTESIAN_POINT ( 'NONE',  ( -3.992867117591420545, 8.524771480177605554, 7.499999999999997335 ) ) ;
#36596=VECTOR ( 'NONE', #18613, 1000.000000000000000 ) ;
#36598=ORIENTED_EDGE ( 'NONE', *, *, #37103, .F. ) ;
#36600=EDGE_CURVE ( 'NONE', #3501, #400, #38680, .T. ) ;
#36601=CARTESIAN_POINT ( 'NONE',  ( -14.57486473880221745, 26.18419839932921533, 11.00000000000000000 ) ) ;
#36602=EDGE_CURVE ( 'NONE', #23885, #9748, #18094, .T. ) ;
#36605=VECTOR ( 'NONE', #17929, 1000.000000000000114 ) ;
#36608=CARTESIAN_POINT ( 'NONE',  ( 8.412270287199559604, 10.07085245822950981, 10.49999999999999822 ) ) ;
#36609=CARTESIAN_POINT ( 'NONE',  ( -12.80736835487442349, 15.68301270189233954, 11.00000000000000000 ) ) ;
#36610=CARTESIAN_POINT ( 'NONE',  ( -14.06524961900331583, 27.71236540882611976, 7.000000000000000000 ) ) ;
#36611=ORIENTED_EDGE ( 'NONE', *, *, #14867, .F. ) ;
#36613=VECTOR ( 'NONE', #14875, 1000.000000000000114 ) ;
#36614=VERTEX_POINT ( 'NONE', #15433 ) ;
#36620=ORIENTED_EDGE ( 'NONE', *, *, #35595, .T. ) ;
#36622=ORIENTED_EDGE ( 'NONE', *, *, #9617, .T. ) ;
#36624=CARTESIAN_POINT ( 'NONE',  ( -6.864468484317908903, 35.45925531351075222, 10.49999999999999645 ) ) ;
#36626=ADVANCED_FACE ( 'NONE', ( #30680 ), #21722, .T. ) ;
#36628=VECTOR ( 'NONE', #4470, 1000.000000000000114 ) ;
#36629=ORIENTED_EDGE ( 'NONE', *, *, #8407, .T. ) ;
#36633=LINE ( 'NONE', #21189, #13796 ) ;
#36636=DIRECTION ( 'NONE',  ( 0.6445931928399499800, 0.000000000000000000, 0.7645257456386926886 ) ) ;
#36637=DIRECTION ( 'NONE',  ( 0.4067366430758009299, 0.9135454576426005335, 0.000000000000000000 ) ) ;
#36638=ORIENTED_EDGE ( 'NONE', *, *, #31263, .F. ) ;
#36643=EDGE_LOOP ( 'NONE', ( #19432, #27957, #34045, #38688 ) ) ;
#36645=DIRECTION ( 'NONE',  ( 0.1045284632676437703, -0.9945218953682742891, 0.000000000000000000 ) ) ;
#36647=DIRECTION ( 'NONE',  ( -0.000000000000000000, -0.000000000000000000, -1.000000000000000000 ) ) ;
#36649=PLANE ( 'NONE',  #9115 ) ;
#36650=ADVANCED_FACE ( 'NONE', ( #12381 ), #2843, .T. ) ;
#36652=VECTOR ( 'NONE', #19651, 1000.000000000000114 ) ;
#36655=ORIENTED_EDGE ( 'NONE', *, *, #30468, .T. ) ;
#36660=CARTESIAN_POINT ( 'NONE',  ( 11.87435565298210882, 15.06698729810772619, 10.00000000000000000 ) ) ;
#36668=ORIENTED_EDGE ( 'NONE', *, *, #26974, .F. ) ;
#36669=CARTESIAN_POINT ( 'NONE',  ( -14.47283171447380212, 21.48159823030330884, 11.00000000000000355 ) ) ;
#36670=VERTEX_POINT ( 'NONE', #27028 ) ;
#36674=EDGE_CURVE ( 'NONE', #31582, #2112, #24174, .T. ) ;
#36675=CARTESIAN_POINT ( 'NONE',  ( -5.947717410344456113, 34.62949535663729250, 10.50000000000000000 ) ) ;
#36684=DIRECTION ( 'NONE',  ( 1.000000000000000000, 0.000000000000000000, 0.000000000000000000 ) ) ;
#36685=EDGE_CURVE ( 'NONE', #21498, #13490, #35433, .T. ) ;
#36686=DIRECTION ( 'NONE',  ( -0.1045284632676422437, 0.9945218953682746221, 0.000000000000000000 ) ) ;
#36687=DIRECTION ( 'NONE',  ( 0.5254827454987509583, -0.4731467892558243182, -0.7071067811865472397 ) ) ;
#36688=VECTOR ( 'NONE', #2736, 1000.000000000000000 ) ;
#36693=ADVANCED_FACE ( 'NONE', ( #24772 ), #21671, .T. ) ;
#36694=VECTOR ( 'NONE', #3045, 1000.000000000000114 ) ;
#36695=CARTESIAN_POINT ( 'NONE',  ( 5.034171952702014785, 35.03623199971300295, 10.50000000000000000 ) ) ;
#36697=CARTESIAN_POINT ( 'NONE',  ( -14.09933648065464062, 26.02968990214173317, 7.000000000000000000 ) ) ;
#36698=DIRECTION ( 'NONE',  ( 0.000000000000000000, 0.000000000000000000, -1.000000000000000000 ) ) ;
#36700=ADVANCED_FACE ( 'NONE', ( #30482 ), #17896, .T. ) ;
#36701=LINE ( 'NONE', #24304, #22315 ) ;
#36703=EDGE_CURVE ( 'NONE', #21181, #37730, #27052, .T. ) ;
#36704=CARTESIAN_POINT ( 'NONE',  ( -11.44134295108998955, 15.31698729810788784, 10.00000000000000000 ) ) ;
#36707=PLANE ( 'NONE',  #32153 ) ;
#36708=CARTESIAN_POINT ( 'NONE',  ( -7.713869163866016621, 10.18146832927085121, 10.49999999999999822 ) ) ;
#36709=CARTESIAN_POINT ( 'NONE',  ( -13.87104230352202272, 20.53934056656885687, 9.500000000000000000 ) ) ;
#36711=DIRECTION ( 'NONE',  ( -0.1045284632676437564, 0.9945218953682744001, 0.000000000000000000 ) ) ;
#36715=LINE ( 'NONE', #39947, #25613 ) ;
#36718=DIRECTION ( 'NONE',  ( 0.6724985119639513842, 0.2185080122244070777, -0.7071067811865541231 ) ) ;
#36720=CARTESIAN_POINT ( 'NONE',  ( 4.955893845527869601, 31.78717482294046093, 10.74999999999999289 ) ) ;
#36725=ORIENTED_EDGE ( 'NONE', *, *, #2698, .T. ) ;
#36726=DIRECTION ( 'NONE',  ( 0.9781476007338072431, 0.2079116908177517375, 0.000000000000000000 ) ) ;
#36727=CARTESIAN_POINT ( 'NONE',  ( -9.892954722048926897, 20.95745441963943279, 10.49999999999999289 ) ) ;
#36732=EDGE_CURVE ( 'NONE', #38335, #32089, #16238, .T. ) ;
#36739=ORIENTED_EDGE ( 'NONE', *, *, #10527, .F. ) ;
#36740=CARTESIAN_POINT ( 'NONE',  ( 2.518583951651050867, 7.712953814960687104, 7.499999999999990230 ) ) ;
#36741=CARTESIAN_POINT ( 'NONE',  ( 9.892954722048896699, 20.95745441963929423, 10.50000000000000533 ) ) ;
#36742=VECTOR ( 'NONE', #8129, 1000.000000000000000 ) ;
#36746=CONICAL_SURFACE ( 'NONE', #11428, 1.000000000000004441, 0.7853981633974522758 ) ;
#36747=ORIENTED_EDGE ( 'NONE', *, *, #7096, .T. ) ;
#36749=VERTEX_POINT ( 'NONE', #15835 ) ;
#36751=DIRECTION ( 'NONE',  ( 0.4999999999999921174, -0.8660254037844431485, -0.000000000000000000 ) ) ;
#36753=ORIENTED_EDGE ( 'NONE', *, *, #9062, .T. ) ;
#36755=CARTESIAN_POINT ( 'NONE',  ( -12.67417846324130259, 14.47720745114830443, 7.499999999999993783 ) ) ;
#36761=ORIENTED_EDGE ( 'NONE', *, *, #2944, .F. ) ;
#36763=CARTESIAN_POINT ( 'NONE',  ( -3.503793317224518145, 8.420815634768723967, 11.00000000000000000 ) ) ;
#36768=VECTOR ( 'NONE', #26475, 1000.000000000000000 ) ;
#36771=CARTESIAN_POINT ( 'NONE',  ( -6.404490139165758933, 34.42612703509939820, 9.500000000000000000 ) ) ;
#36772=EDGE_LOOP ( 'NONE', ( #29427, #10157, #30532, #7172 ) ) ;
#36775=CARTESIAN_POINT ( 'NONE',  ( -14.78469161520108699, 20.18088120075973535, 10.49999999999999467 ) ) ;
#36777=DIRECTION ( 'NONE',  ( 0.9945218953682729568, -0.1045284632676570929, -0.000000000000000000 ) ) ;
#36778=EDGE_LOOP ( 'NONE', ( #25920, #32548, #31244, #1247, #14945 ) ) ;
#36781=CARTESIAN_POINT ( 'NONE',  ( -14.52509594610762456, 21.97885917798744870, 11.00000000000000000 ) ) ;
#36784=DIRECTION ( 'NONE',  ( -1.000000000000000000, 0.000000000000000000, 0.000000000000000000 ) ) ;
#36785=ORIENTED_EDGE ( 'NONE', *, *, #3168, .F. ) ;
#36793=CARTESIAN_POINT ( 'NONE',  ( -3.503793317224520365, 8.420815634768723967, 11.00000000000000000 ) ) ;
#36794=ORIENTED_EDGE ( 'NONE', *, *, #5319, .F. ) ;
#36795=ADVANCED_FACE ( 'NONE', ( #22515 ), #13174, .F. ) ;
#36797=CARTESIAN_POINT ( 'NONE',  ( 5.473344025737211460, 14.11593743010426394, 10.49999999999999822 ) ) ;
#36801=CARTESIAN_POINT ( 'NONE',  ( -14.99905852611806445, 22.33194247983213643, 7.000000000000000000 ) ) ;
#36802=EDGE_CURVE ( 'NONE', #9003, #39481, #28021, .T. ) ;
#36803=CARTESIAN_POINT ( 'NONE',  ( 2.036571916123615100, 8.108948098542045457, 10.49999999999999467 ) ) ;
#36806=CARTESIAN_POINT ( 'NONE',  ( -9.705584749708384251, 11.06314620770957013, 7.221809905720049549 ) ) ;
#36807=CARTESIAN_POINT ( 'NONE',  ( -3.161220354320354531, 12.43736188311282653, 10.50000000000000000 ) ) ;
#36808=CARTESIAN_POINT ( 'NONE',  ( 10.21799113078985677, 32.82168114676792925, 10.66666666666666430 ) ) ;
#36809=VERTEX_POINT ( 'NONE', #9742 ) ;
#36810=VERTEX_POINT ( 'NONE', #7076 ) ;
#36814=CARTESIAN_POINT ( 'NONE',  ( 3.607749162633204332, 7.931741834401770497, 10.49999999999999822 ) ) ;
#36815=ORIENTED_EDGE ( 'NONE', *, *, #36498, .T. ) ;
#36816=ORIENTED_EDGE ( 'NONE', *, *, #27719, .T. ) ;
#36818=CARTESIAN_POINT ( 'NONE',  ( 13.57128027507778789, 27.95460132399998443, 10.49999999999999822 ) ) ;
#36820=DIRECTION ( 'NONE',  ( -0.000000000000000000, -0.000000000000000000, -1.000000000000000000 ) ) ;
#36822=VERTEX_POINT ( 'NONE', #197 ) ;
#36828=DIRECTION ( 'NONE',  ( 1.000000000000000000, 0.000000000000000000, 0.000000000000000000 ) ) ;
#36832=VERTEX_POINT ( 'NONE', #791 ) ;
#36834=ORIENTED_EDGE ( 'NONE', *, *, #35969, .F. ) ;
#36836=AXIS2_PLACEMENT_3D ( 'NONE', #4803, #26336, #29584 ) ;
#36838=ORIENTED_EDGE ( 'NONE', *, *, #18485, .T. ) ;
#36840=CARTESIAN_POINT ( 'NONE',  ( -8.910254037844422825, 17.93301270189230223, 10.49999999999999822 ) ) ;
#36842=CARTESIAN_POINT ( 'NONE',  ( -2.525645716490712012, 8.212903943950955465, 11.00000000000000000 ) ) ;
#36845=EDGE_CURVE ( 'NONE', #36810, #5091, #25176, .T. ) ;
#36846=AXIS2_PLACEMENT_3D ( 'NONE', #20148, #10194, #38227 ) ;
#36847=CIRCLE ( 'NONE', #33656, 6.000000000000005329 ) ;
#36848=CARTESIAN_POINT ( 'NONE',  ( 0.000000000000000000, 22.50000000000000355, 7.000000000000000000 ) ) ;
#36849=CARTESIAN_POINT ( 'NONE',  ( -17.05532387642082526, 7.816133769664412867, 11.00000000000000000 ) ) ;
#36850=ORIENTED_EDGE ( 'NONE', *, *, #24010, .F. ) ;
#36852=PLANE ( 'NONE',  #28809 ) ;
#36854=DIRECTION ( 'NONE',  ( -0.8090169943749504489, -0.5877852522924691403, 0.000000000000000000 ) ) ;
#36856=CIRCLE ( 'NONE', #6991, 0.4999999999999995559 ) ;
#36859=CIRCLE ( 'NONE', #6992, 0.5000000000000004441 ) ;
#36870=CARTESIAN_POINT ( 'NONE',  ( -0.5000000000000004441, 37.00000000000000711, 7.000000000000000000 ) ) ;
#36872=LINE ( 'NONE', #9043, #21739 ) ;
#36875=CARTESIAN_POINT ( 'NONE',  ( -14.64659974985906210, 21.96608861361228904, 10.49999999999999822 ) ) ;
#36879=DIRECTION ( 'NONE',  ( 1.000000000000000000, 0.000000000000000000, 0.000000000000000000 ) ) ;
#36880=EDGE_CURVE ( 'NONE', #32024, #659, #17678, .T. ) ;
#36881=CARTESIAN_POINT ( 'NONE',  ( -11.44473057578096942, 31.45924896672619298, 10.49999999999999822 ) ) ;
#36882=EDGE_CURVE ( 'NONE', #10398, #16279, #9545, .T. ) ;
#36883=PLANE ( 'NONE',  #14800 ) ;
#36884=ORIENTED_EDGE ( 'NONE', *, *, #5871, .T. ) ;
#36886=TOROIDAL_SURFACE ( 'NONE', #20038, 1.000000000000000000, 0.5000000000000000000 ) ;
#36889=FACE_OUTER_BOUND ( 'NONE', #2094, .T. ) ;
#36891=EDGE_LOOP ( 'NONE', ( #13220, #40020, #1030, #39372, #18251 ) ) ;
#36898=ADVANCED_FACE ( 'NONE', ( #21922 ), #10009, .T. ) ;
#36900=DIRECTION ( 'NONE',  ( 1.000000000000000000, 0.000000000000000000, 0.000000000000000000 ) ) ;
#36903=LINE ( 'NONE', #27754, #22732 ) ;
#36904=CARTESIAN_POINT ( 'NONE',  ( 14.04642159563909942, 39.70023260537602994, 10.00000000000000000 ) ) ;
#36905=DIRECTION ( 'NONE',  ( -1.000000000000000000, 0.000000000000000000, 0.000000000000000000 ) ) ;
#36907=CARTESIAN_POINT ( 'NONE',  ( 14.46080647158823318, 26.53523365061236561, 10.49999999999999645 ) ) ;
#36911=AXIS2_PLACEMENT_3D ( 'NONE', #38626, #20147, #32546 ) ;
#36912=ORIENTED_EDGE ( 'NONE', *, *, #21061, .F. ) ;
#36915=AXIS2_PLACEMENT_3D ( 'NONE', #21791, #267, #38033 ) ;
#36916=DIRECTION ( 'NONE',  ( 1.533293416683372906E-16, -0.7071067811865474617, -0.7071067811865474617 ) ) ;
#36923=VERTEX_POINT ( 'NONE', #14943 ) ;
#36931=DIRECTION ( 'NONE',  ( -0.8660254037844432595, -0.4999999999999920064, 0.000000000000000000 ) ) ;
#36943=VECTOR ( 'NONE', #21861, 999.9999999999998863 ) ;
#36944=VERTEX_POINT ( 'NONE', #38366 ) ;
#36945=DIRECTION ( 'NONE',  ( -0.000000000000000000, -0.000000000000000000, -1.000000000000000000 ) ) ;
#36948=CARTESIAN_POINT ( 'NONE',  ( 14.97191702109865297, 21.44669161452667794, 10.49999999999999822 ) ) ;
#36949=CARTESIAN_POINT ( 'NONE',  ( -11.87435565298220652, 15.06698729810788961, 7.499999999999993783 ) ) ;
#36951=FACE_OUTER_BOUND ( 'NONE', #216, .T. ) ;
#36953=ADVANCED_FACE ( 'NONE', ( #32071 ), #4695, .T. ) ;
#36955=CARTESIAN_POINT ( 'NONE',  ( 13.05736835487433289, 16.11602540378438420, 9.500000000000000000 ) ) ;
#36957=CARTESIAN_POINT ( 'NONE',  ( 2.525645716490518389, 8.212903943950921715, 7.000000000000000000 ) ) ;
#36961=ORIENTED_EDGE ( 'NONE', *, *, #38535, .T. ) ;
#36962=EDGE_CURVE ( 'NONE', #25278, #163, #26086, .T. ) ;
#36972=CARTESIAN_POINT ( 'NONE',  ( 11.40045258775034931, 32.09219725203293194, 10.82238833324614191 ) ) ;
#36979=EDGE_CURVE ( 'NONE', #32514, #16315, #21567, .T. ) ;
#36980=DIRECTION ( 'NONE',  ( -0.6724985119639524944, 0.2185080122244146827, -0.7071067811865507924 ) ) ;
#36981=VERTEX_POINT ( 'NONE', #19887 ) ;
#36983=LINE ( 'NONE', #410, #8969 ) ;
#36984=FACE_OUTER_BOUND ( 'NONE', #39181, .T. ) ;
#36988=EDGE_LOOP ( 'NONE', ( #21201, #31448, #25327 ) ) ;
#36993=CARTESIAN_POINT ( 'NONE',  ( -0.6108529249775870307, 37.48755679569043053, 7.500000000000000888 ) ) ;
#36996=CARTESIAN_POINT ( 'NONE',  ( 5.136393443230283573, 36.08535633838087620, 10.66666666666666607 ) ) ;
#36997=VERTEX_POINT ( 'NONE', #35121 ) ;
#36998=ADVANCED_FACE ( 'NONE', ( #4239 ), #24150, .T. ) ;
#36999=CARTESIAN_POINT ( 'NONE',  ( -10.44103466624267540, 32.57396620494226624, 11.00000000000000000 ) ) ;
#37000=LINE ( 'NONE', #36797, #37705 ) ;
#37001=AXIS2_PLACEMENT_3D ( 'NONE', #32662, #21063, #29802 ) ;
#37002=CARTESIAN_POINT ( 'NONE',  ( 12.31033848243464668, 14.30014505118389145, 10.49999999999999467 ) ) ;
#37004=DIRECTION ( 'NONE',  ( -0.000000000000000000, -0.000000000000000000, -1.000000000000000000 ) ) ;
#37006=DIRECTION ( 'NONE',  ( -1.000000000000000000, 0.000000000000000000, 0.000000000000000000 ) ) ;
#37009=VERTEX_POINT ( 'NONE', #1199 ) ;
#37011=AXIS2_PLACEMENT_3D ( 'NONE', #2721, #28895, #7151 ) ;
#37014=CARTESIAN_POINT ( 'NONE',  ( -3.992867117591419213, 8.524771480177605554, 10.49999999999999822 ) ) ;
#37015=ORIENTED_EDGE ( 'NONE', *, *, #35460, .F. ) ;
#37018=B_SPLINE_CURVE_WITH_KNOTS ( 'NONE', 3,
 ( #34594, #1075, #19153, #16110, #28495, #13452 ),
 .UNSPECIFIED., .F., .F.,
 ( 4, 2, 4 ),
 ( 0.000000000000000000, 0.5000000000000000000, 1.000000000000000000 ),
 .UNSPECIFIED. ) ;
#37024=CARTESIAN_POINT ( 'NONE',  ( 13.96188064734268686, 27.98367808437124538, 7.382773698552470343 ) ) ;
#37027=DIRECTION ( 'NONE',  ( 0.000000000000000000, 0.000000000000000000, 1.000000000000000000 ) ) ;
#37029=EDGE_CURVE ( 'NONE', #1914, #16860, #10741, .T. ) ;
#37030=B_SPLINE_CURVE_WITH_KNOTS ( 'NONE', 3,
 ( #31248, #37742, #34690, #19245 ),
 .UNSPECIFIED., .F., .F.,
 ( 4, 4 ),
 ( 0.000000000000000000, 1.000000000000000000 ),
 .UNSPECIFIED. ) ;
#37031=VECTOR ( 'NONE', #29256, 1000.000000000000000 ) ;
#37032=EDGE_LOOP ( 'NONE', ( #22208, #20899, #13987, #10045 ) ) ;
#37034=EDGE_LOOP ( 'NONE', ( #14171, #27673, #9962, #32950 ) ) ;
#37038=ORIENTED_EDGE ( 'NONE', *, *, #34484, .T. ) ;
#37040=CARTESIAN_POINT ( 'NONE',  ( 7.096882951594522204, 29.56287847632727050, 10.50000000000000000 ) ) ;
#37041=CARTESIAN_POINT ( 'NONE',  ( -11.44134295108998955, 15.31698729810788784, 10.50000000000000000 ) ) ;
#37042=AXIS2_PLACEMENT_3D ( 'NONE', #22345, #19110, #31896 ) ;
#37043=PLANE ( 'NONE',  #38218 ) ;
#37044=CIRCLE ( 'NONE', #7155, 0.5000000000000007772 ) ;
#37045=CARTESIAN_POINT ( 'NONE',  ( -2.140527761532693418, 7.619874298175171035, 10.50000000000000000 ) ) ;
#37048=ORIENTED_EDGE ( 'NONE', *, *, #1844, .F. ) ;
#37050=CYLINDRICAL_SURFACE ( 'NONE', #21680, 0.4999999999999998335 ) ;
#37051=ADVANCED_FACE ( 'NONE', ( #18982 ), #300, .F. ) ;
#37052=DIRECTION ( 'NONE',  ( -0.9945218953682730678, 0.1045284632676566905, 7.253119165527330602E-16 ) ) ;
#37054=VECTOR ( 'NONE', #30060, 1000.000000000000227 ) ;
#37055=CARTESIAN_POINT ( 'NONE',  ( -13.30736835483215508, 15.77027916469387847, 10.49999999999999645 ) ) ;
#37057=ORIENTED_EDGE ( 'NONE', *, *, #26202, .F. ) ;
#37062=EDGE_LOOP ( 'NONE', ( #4855, #15954, #3552, #20540 ) ) ;
#37064=ORIENTED_EDGE ( 'NONE', *, *, #29193, .F. ) ;
#37066=DIRECTION ( 'NONE',  ( 0.7431448254773961315, 0.6691306063588561281, 0.000000000000000000 ) ) ;
#37068=LINE ( 'NONE', #30973, #15339 ) ;
#37072=CARTESIAN_POINT ( 'NONE',  ( -14.52509594610762456, 21.97885917798744870, 10.49999999999999467 ) ) ;
#37076=CIRCLE ( 'NONE', #39647, 0.5000000000000004441 ) ;
#37077=EDGE_CURVE ( 'NONE', #13835, #13564, #24284, .T. ) ;
#37078=DIRECTION ( 'NONE',  ( 0.000000000000000000, 0.000000000000000000, 1.000000000000000000 ) ) ;
#37079=CARTESIAN_POINT ( 'NONE',  ( -13.28401428810686724, 15.50858767547201822, 10.49999999999999822 ) ) ;
#37081=EDGE_LOOP ( 'NONE', ( #10025, #12925, #11035, #13512, #38176 ) ) ;
#37086=EDGE_CURVE ( 'NONE', #32089, #747, #27531, .T. ) ;
#37088=ORIENTED_EDGE ( 'NONE', *, *, #4369, .T. ) ;
#37090=EDGE_CURVE ( 'NONE', #12080, #13281, #1447, .T. ) ;
#37092=DIRECTION ( 'NONE',  ( 0.000000000000000000, -0.000000000000000000, -1.000000000000000000 ) ) ;
#37095=VECTOR ( 'NONE', #35709, 1000.000000000000000 ) ;
#37097=DIRECTION ( 'NONE',  ( -0.9781476007338042455, 0.2079116908177664758, 0.000000000000000000 ) ) ;
#37098=ADVANCED_FACE ( 'NONE', ( #12682 ), #27724, .F. ) ;
#37101=ADVANCED_FACE ( 'NONE', ( #18197 ), #25077, .F. ) ;
#37102=DIRECTION ( 'NONE',  ( -0.000000000000000000, -0.000000000000000000, -1.000000000000000000 ) ) ;
#37103=EDGE_CURVE ( 'NONE', #16182, #7701, #11829, .T. ) ;
#37104=DIRECTION ( 'NONE',  ( -0.9986295347545740553, 0.05233595624294183624, -1.941170045126910451E-16 ) ) ;
#37105=LINE ( 'NONE', #37502, #39405 ) ;
#37106=CARTESIAN_POINT ( 'NONE',  ( 11.96428041830149169, 31.54822188126892613, 7.102474990965860435 ) ) ;
#37109=CARTESIAN_POINT ( 'NONE',  ( 9.303655249773111535, 10.73386218874820663, 7.500000000000000888 ) ) ;
#37110=ORIENTED_EDGE ( 'NONE', *, *, #17569, .F. ) ;
#37112=DIRECTION ( 'NONE',  ( 0.000000000000000000, -0.5778781230733920360, -0.8161230758122046680 ) ) ;
#37113=CARTESIAN_POINT ( 'NONE',  ( 8.796116341590819232, 23.42450908139080568, 9.000000000000001776 ) ) ;
#37114=CIRCLE ( 'NONE', #29983, 0.5000000000000004441 ) ;
#37119=ORIENTED_EDGE ( 'NONE', *, *, #38079, .T. ) ;
#37127=DIRECTION ( 'NONE',  ( 1.000000000000000000, -4.163336342344304841E-14, 0.000000000000000000 ) ) ;
#37131=ADVANCED_FACE ( 'NONE', ( #6576 ), #34426, .F. ) ;
#37133=ORIENTED_EDGE ( 'NONE', *, *, #15603, .F. ) ;
#37139=CIRCLE ( 'NONE', #24807, 0.5000000000000004441 ) ;
#37142=DIRECTION ( 'NONE',  ( 0.8090169943749426773, -0.5877852522924796874, -0.000000000000000000 ) ) ;
#37144=AXIS2_PLACEMENT_3D ( 'NONE', #13682, #35427, #22415 ) ;
#37148=DIRECTION ( 'NONE',  ( -0.7431448254773953543, -0.6691306063588570163, 0.000000000000000000 ) ) ;
#37150=EDGE_CURVE ( 'NONE', #21371, #22721, #33837, .T. ) ;
#37153=EDGE_CURVE ( 'NONE', #31037, #29721, #21628, .T. ) ;
#37156=ORIENTED_EDGE ( 'NONE', *, *, #19689, .T. ) ;
#37160=LINE ( 'NONE', #21911, #20413 ) ;
#37162=CARTESIAN_POINT ( 'NONE',  ( -10.72501808743014884, 33.00580893829974372, 10.49999999999999645 ) ) ;
#37167=AXIS2_PLACEMENT_3D ( 'NONE', #16530, #28913, #12611 ) ;
#37168=CARTESIAN_POINT ( 'NONE',  ( 11.58426073497340880, 31.66040656113755603, 10.49999999999999822 ) ) ;
#37169=ORIENTED_EDGE ( 'NONE', *, *, #16006, .T. ) ;
#37171=DIRECTION ( 'NONE',  ( -0.4999999999999933942, 0.8660254037844425934, 0.000000000000000000 ) ) ;
#37172=ADVANCED_FACE ( 'NONE', ( #2747 ), #24815, .T. ) ;
#37173=CARTESIAN_POINT ( 'NONE',  ( -8.169448529985462670, 9.961039561530412811, 10.49999999999999467 ) ) ;
#37174=VECTOR ( 'NONE', #26682, 1000.000000000000114 ) ;
#37175=CARTESIAN_POINT ( 'NONE',  ( -9.331903152615897312, 11.35703883385580859, 10.49999999999999822 ) ) ;
#37176=ORIENTED_EDGE ( 'NONE', *, *, #37229, .T. ) ;
#37178=EDGE_CURVE ( 'NONE', #21244, #17938, #35326, .T. ) ;
#37179=DIRECTION ( 'NONE',  ( -0.2079116908177533474, 0.9781476007338067991, -0.000000000000000000 ) ) ;
#37180=EDGE_CURVE ( 'NONE', #481, #14680, #9134, .T. ) ;
#37181=CARTESIAN_POINT ( 'NONE',  ( 4.527363138135212850, 36.35651410043141141, 7.000000000000000000 ) ) ;
#37184=DIRECTION ( 'NONE',  ( -0.1470157664651947915, 0.6916548014802283983, -0.7071067811865455743 ) ) ;
#37185=AXIS2_PLACEMENT_3D ( 'NONE', #7410, #10066, #19817 ) ;
#37186=VERTEX_POINT ( 'NONE', #30978 ) ;
#37188=EDGE_CURVE ( 'NONE', #1779, #13010, #3144, .T. ) ;
#37189=EDGE_LOOP ( 'NONE', ( #17912, #33519, #31639, #3695, #28861 ) ) ;
#37192=DIRECTION ( 'NONE',  ( 0.000000000000000000, 0.000000000000000000, 1.000000000000000000 ) ) ;
#37194=AXIS2_PLACEMENT_3D ( 'NONE', #7058, #38144, #16415 ) ;
#37196=ORIENTED_EDGE ( 'NONE', *, *, #15393, .T. ) ;
#37197=CARTESIAN_POINT ( 'NONE',  ( -13.63581098909220479, 27.45627467658446008, 7.499999999999993783 ) ) ;
#37198=CARTESIAN_POINT ( 'NONE',  ( -10.54700836463452340, 22.39697303105802106, 10.50000000000000000 ) ) ;
#37200=EDGE_CURVE ( 'NONE', #31380, #18974, #18788, .T. ) ;
#37201=EDGE_CURVE ( 'NONE', #24961, #2306, #9254, .T. ) ;
#37202=LINE ( 'NONE', #35554, #35734 ) ;
#37205=AXIS2_PLACEMENT_3D ( 'NONE', #1737, #33029, #23864 ) ;
#37208=FACE_OUTER_BOUND ( 'NONE', #25516, .T. ) ;
#37209=CARTESIAN_POINT ( 'NONE',  ( -4.987329993433320396E-14, 13.65543219052647927, 9.000000000000001776 ) ) ;
#37210=EDGE_LOOP ( 'NONE', ( #31519, #35335, #26190, #1688 ) ) ;
#37215=LINE ( 'NONE', #21375, #6843 ) ;
#37216=ORIENTED_EDGE ( 'NONE', *, *, #34083, .T. ) ;
#37217=ORIENTED_EDGE ( 'NONE', *, *, #29513, .F. ) ;
#37220=EDGE_CURVE ( 'NONE', #24016, #32625, #22216, .T. ) ;
#37223=ORIENTED_EDGE ( 'NONE', *, *, #20816, .T. ) ;
#37226=CARTESIAN_POINT ( 'NONE',  ( 14.84160187385922036, 20.32586711126977619, 7.500000000000010658 ) ) ;
#37227=ORIENTED_EDGE ( 'NONE', *, *, #35456, .F. ) ;
#37229=EDGE_CURVE ( 'NONE', #13902, #12954, #25868, .T. ) ;
#37230=CARTESIAN_POINT ( 'NONE',  ( -14.36830325120615548, 20.48707633493503621, 9.000000000000001776 ) ) ;
#37231=LINE ( 'NONE', #9002, #25130 ) ;
#37236=VECTOR ( 'NONE', #39188, 1000.000000000000000 ) ;
#37241=CARTESIAN_POINT ( 'NONE',  ( -14.61143855090110932, 25.89393895760251851, 7.097463131219505783 ) ) ;
#37244=FACE_OUTER_BOUND ( 'NONE', #13344, .T. ) ;
#37245=CARTESIAN_POINT ( 'NONE',  ( 8.118377661053324701, 10.47536095541698486, 7.000000000000000000 ) ) ;
#37246=B_SPLINE_SURFACE_WITH_KNOTS ( 'NONE', 1, 3, ( 
 ( #17428, #38947, #36501, #8264, #23904, #11718, #35902, #36306, #33469, #8469 ),
 ( #20263, #11119, #11322, #39139, #23503, #7858, #5611, #23705, #29598, #4818 ) ),
 .UNSPECIFIED., .F., .F., .F.,
 ( 2, 2 ),
 ( 4, 2, 2, 2, 4 ),
 ( 0.000000000000000000, 1.000000000000000000 ),
 ( 1.875797233020323640, 2.268496314719047557, 2.661195396417771697, 3.053894478116495836, 3.446593559815219976 ),
 .UNSPECIFIED. ) ;
#37253=CARTESIAN_POINT ( 'NONE',  ( -2.140527761532693418, 7.619874298175171035, 11.00000000000000000 ) ) ;
#37262=DIRECTION ( 'NONE',  ( 0.000000000000000000, 0.000000000000000000, 1.000000000000000000 ) ) ;
#37263=VERTEX_POINT ( 'NONE', #19578 ) ;
#37267=CARTESIAN_POINT ( 'NONE',  ( 12.74038105676654453, 14.56698729810772264, 10.50000000000000178 ) ) ;
#37270=VECTOR ( 'NONE', #36508, 1000.000000000000114 ) ;
#37272=DIRECTION ( 'NONE',  ( -0.5877852522924796874, -0.8090169943749426773, 0.000000000000000000 ) ) ;
#37276=DIRECTION ( 'NONE',  ( -0.000000000000000000, -0.000000000000000000, -1.000000000000000000 ) ) ;
#37277=DIRECTION ( 'NONE',  ( 0.000000000000000000, 0.000000000000000000, -1.000000000000000000 ) ) ;
#37281=AXIS2_PLACEMENT_3D ( 'NONE', #36562, #21124, #8936 ) ;
#37286=AXIS2_PLACEMENT_3D ( 'NONE', #39101, #16573, #38907 ) ;
#37288=LINE ( 'NONE', #5812, #27091 ) ;
#37290=ORIENTED_EDGE ( 'NONE', *, *, #442, .T. ) ;
#37291=CARTESIAN_POINT ( 'NONE',  ( -6.576253646258509278, 14.29921418520934218, 10.50000000000000000 ) ) ;
#37293=CARTESIAN_POINT ( 'NONE',  ( 12.97403502154100607, 15.97168783648697499, 10.66666666666666252 ) ) ;
#37296=EDGE_CURVE ( 'NONE', #11885, #27294, #35171, .T. ) ;
#37297=LINE ( 'NONE', #9471, #39621 ) ;
#37298=DIRECTION ( 'NONE',  ( 1.000000000000000000, 0.000000000000000000, 0.000000000000000000 ) ) ;
#37299=FACE_OUTER_BOUND ( 'NONE', #7405, .T. ) ;
#37300=DIRECTION ( 'NONE',  ( -0.000000000000000000, -0.000000000000000000, -1.000000000000000000 ) ) ;
#37302=VECTOR ( 'NONE', #1250, 1000.000000000000000 ) ;
#37304=DIRECTION ( 'NONE',  ( 1.000000000000000000, 0.000000000000000000, 0.000000000000000000 ) ) ;
#37307=LINE ( 'NONE', #11930, #24610 ) ;
#37309=CARTESIAN_POINT ( 'NONE',  ( 12.97058434440062769, 15.58877990640313449, 10.96580508970283141 ) ) ;
#37311=ADVANCED_FACE ( 'NONE', ( #16540 ), #7587, .T. ) ;
#37316=VECTOR ( 'NONE', #8027, 1000.000000000000000 ) ;
#37321=CONICAL_SURFACE ( 'NONE', #19804, 1.000000000000002665, 0.7853981633974579379 ) ;
#37326=DIRECTION ( 'NONE',  ( -1.000000000000000000, -1.224646799147353947E-16, 0.000000000000000000 ) ) ;
#37330=ORIENTED_EDGE ( 'NONE', *, *, #39241, .T. ) ;
#37331=DIRECTION ( 'NONE',  ( 1.000000000000000000, 0.000000000000000000, 0.000000000000000000 ) ) ;
#37332=EDGE_CURVE ( 'NONE', #13142, #6492, #40135, .T. ) ;
#37337=VECTOR ( 'NONE', #23583, 999.9999999999998863 ) ;
#37340=DIRECTION ( 'NONE',  ( 1.000000000000000000, 0.000000000000000000, 0.000000000000000000 ) ) ;
#37341=ORIENTED_EDGE ( 'NONE', *, *, #31848, .F. ) ;
#37344=AXIS2_PLACEMENT_3D ( 'NONE', #32411, #14109, #4971 ) ;
#37346=FACE_OUTER_BOUND ( 'NONE', #30582, .T. ) ;
#37349=CARTESIAN_POINT ( 'NONE',  ( 8.412270287199559604, 10.07085245822951158, 10.63089969389957545 ) ) ;
#37351=LINE ( 'NONE', #6852, #22776 ) ;
#37352=EDGE_CURVE ( 'NONE', #7643, #10090, #3387, .T. ) ;
#37353=CARTESIAN_POINT ( 'NONE',  ( -10.81260707898136708, 32.90853150812170469, 10.49999999999999822 ) ) ;
#37355=VERTEX_POINT ( 'NONE', #32179 ) ;
#37359=DIRECTION ( 'NONE',  ( 0.9945218953682746221, 0.1045284632676422437, 0.000000000000000000 ) ) ;
#37362=CARTESIAN_POINT ( 'NONE',  ( 9.427394655416197367, 11.16786596286755362, 10.49999999999999822 ) ) ;
#37368=CARTESIAN_POINT ( 'NONE',  ( -9.625795778762141097, 10.95253033666833886, 10.49999999999999822 ) ) ;
#37369=EDGE_LOOP ( 'NONE', ( #2238, #37619, #3358 ) ) ;
#37371=CIRCLE ( 'NONE', #9473, 0.9999999999999986677 ) ;
#37372=CARTESIAN_POINT ( 'NONE',  ( 0.9461134518049061359, 37.26099332938164821, 10.49999999999999467 ) ) ;
#37373=LINE ( 'NONE', #37575, #31636 ) ;
#37374=CIRCLE ( 'NONE', #30248, 15.00000000000000000 ) ;
#37375=CYLINDRICAL_SURFACE ( 'NONE', #5958, 0.5000000000000004441 ) ;
#37378=CARTESIAN_POINT ( 'NONE',  ( -14.42035624161473883, 26.65972665747678860, 10.49999999999999822 ) ) ;
#37384=CARTESIAN_POINT ( 'NONE',  ( -14.09933648065464062, 26.02968990214173317, 7.499999999999993783 ) ) ;
#37385=ORIENTED_EDGE ( 'NONE', *, *, #35993, .F. ) ;
#37387=VERTEX_POINT ( 'NONE', #4135 ) ;
#37389=CARTESIAN_POINT ( 'NONE',  ( 11.48173768534036121, 32.16538668264416145, 11.00000000000000000 ) ) ;
#37392=DIRECTION ( 'NONE',  ( 0.8660254037844362651, -0.5000000000000041078, 0.000000000000000000 ) ) ;
#37393=ORIENTED_EDGE ( 'NONE', *, *, #17865, .T. ) ;
#37394=CARTESIAN_POINT ( 'NONE',  ( 3.992867117591238468, 8.524771480177550487, 10.49999999999999822 ) ) ;
#37397=DIRECTION ( 'NONE',  ( 1.000000000000000000, 0.000000000000000000, 0.000000000000000000 ) ) ;
#37400=CIRCLE ( 'NONE', #10145, 0.5000000000000000000 ) ;
#37402=CIRCLE ( 'NONE', #10150, 0.4999999999999998335 ) ;
#37403=ADVANCED_FACE ( 'NONE', ( #38065 ), #29127, .T. ) ;
#37409=EDGE_CURVE ( 'NONE', #39304, #25736, #19647, .T. ) ;
#37413=VERTEX_POINT ( 'NONE', #25463 ) ;
#37414=ORIENTED_EDGE ( 'NONE', *, *, #3069, .T. ) ;
#37418=VERTEX_POINT ( 'NONE', #11053 ) ;
#37421=LINE ( 'NONE', #9597, #170 ) ;
#37422=ORIENTED_EDGE ( 'NONE', *, *, #8934, .T. ) ;
#37425=LINE ( 'NONE', #9601, #34210 ) ;
#37427=EDGE_CURVE ( 'NONE', #5336, #12231, #32793, .T. ) ;
#37429=EDGE_LOOP ( 'NONE', ( #19055, #7752, #1774 ) ) ;
#37430=EDGE_CURVE ( 'NONE', #18869, #19973, #17556, .T. ) ;
#37432=VECTOR ( 'NONE', #23292, 1000.000000000000000 ) ;
#37436=EDGE_LOOP ( 'NONE', ( #24836, #28646, #4964 ) ) ;
#37438=CARTESIAN_POINT ( 'NONE',  ( 9.343266739736582949, 17.68301270189218855, 10.50000000000000000 ) ) ;
#37440=VECTOR ( 'NONE', #24906, 1000.000000000000114 ) ;
#37441=DIRECTION ( 'NONE',  ( -0.8660254037844432595, -0.4999999999999921729, 0.000000000000000000 ) ) ;
#37442=DIRECTION ( 'NONE',  ( -1.000000000000000000, 0.000000000000000000, 0.000000000000000000 ) ) ;
#37444=EDGE_CURVE ( 'NONE', #19849, #34816, #35829, .T. ) ;
#37446=EDGE_CURVE ( 'NONE', #20131, #9944, #7986, .T. ) ;
#37452=CARTESIAN_POINT ( 'NONE',  ( -14.47283171447380035, 21.48159823030330884, 7.000000000000000000 ) ) ;
#37455=ORIENTED_EDGE ( 'NONE', *, *, #4660, .F. ) ;
#37457=CIRCLE ( 'NONE', #16704, 0.5000000000000000000 ) ;
#37460=DIRECTION ( 'NONE',  ( 0.000000000000000000, 0.000000000000000000, -1.000000000000000000 ) ) ;
#37462=ORIENTED_EDGE ( 'NONE', *, *, #14214, .F. ) ;
#37463=DIRECTION ( 'NONE',  ( 1.000000000000000000, 0.000000000000000000, -0.000000000000000000 ) ) ;
#37464=EDGE_LOOP ( 'NONE', ( #29774, #4249, #32571 ) ) ;
#37468=CARTESIAN_POINT ( 'NONE',  ( -5.440908595777639079, 35.94977745735568675, 9.500000000000000000 ) ) ;
#37477=CARTESIAN_POINT ( 'NONE',  ( -7.353987181296344211, 35.57359447655193208, 7.000000000000000000 ) ) ;
#37479=CARTESIAN_POINT ( 'NONE',  ( 2.525645716490518833, 8.212903943950921715, 7.499999999999990230 ) ) ;
#37480=ORIENTED_EDGE ( 'NONE', *, *, #4369, .F. ) ;
#37481=EDGE_CURVE ( 'NONE', #36809, #22627, #14462, .T. ) ;
#37483=EDGE_CURVE ( 'NONE', #32345, #35666, #24036, .T. ) ;
#37486=VERTEX_POINT ( 'NONE', #26279 ) ;
#37488=CARTESIAN_POINT ( 'NONE',  ( 1.000000000000000000, 37.00000000000000711, 10.50000000000000178 ) ) ;
#37489=CONICAL_SURFACE ( 'NONE', #8959, 1.000000000000007772, 0.7853981633974557175 ) ;
#37490=CONICAL_SURFACE ( 'NONE', #25159, 1.000000000000000444, 0.7853981633974482790 ) ;
#37492=CARTESIAN_POINT ( 'NONE',  ( -11.77929587896040786, 31.08767655398749596, 7.000000000000000000 ) ) ;
#37493=AXIS2_PLACEMENT_3D ( 'NONE', #31149, #30753, #14913 ) ;
#37494=CIRCLE ( 'NONE', #22548, 1.000000000000000888 ) ;
#37499=CARTESIAN_POINT ( 'NONE',  ( -5.187504188494229673, 36.60991850771488743, 10.50000000000000533 ) ) ;
#37500=FACE_OUTER_BOUND ( 'NONE', #38115, .T. ) ;
#37501=DIRECTION ( 'NONE',  ( 0.9781476007338036904, -0.2079116908177680301, 0.000000000000000000 ) ) ;
#37502=CARTESIAN_POINT ( 'NONE',  ( 0.5000000000000006661, 32.50000000000000000, 10.00000000000000000 ) ) ;
#37503=CARTESIAN_POINT ( 'NONE',  ( -0.4999999999999998890, 37.50000000000000711, 10.49999999999999822 ) ) ;
#37504=DIRECTION ( 'NONE',  ( -0.000000000000000000, -0.000000000000000000, -1.000000000000000000 ) ) ;
#37506=DIRECTION ( 'NONE',  ( 0.000000000000000000, 0.000000000000000000, 1.000000000000000000 ) ) ;
#37509=CARTESIAN_POINT ( 'NONE',  ( 13.97557076678965693, 21.53386246193694475, 7.500000000000010658 ) ) ;
#37510=CARTESIAN_POINT ( 'NONE',  ( 14.36830325120613061, 20.48707633493482660, 11.00000000000000000 ) ) ;
#37524=EDGE_LOOP ( 'NONE', ( #9257, #21227, #20771, #7442 ) ) ;
#37526=CARTESIAN_POINT ( 'NONE',  ( 13.49038105676655164, 15.86602540378438064, 11.00000000000000000 ) ) ;
#37532=VERTEX_POINT ( 'NONE', #36431 ) ;
#37533=LINE ( 'NONE', #12346, #29753 ) ;
#37534=EDGE_CURVE ( 'NONE', #23608, #36809, #2154, .T. ) ;
#37541=DIRECTION ( 'NONE',  ( 1.000000000000000000, 0.000000000000000000, 0.000000000000000000 ) ) ;
#37542=ORIENTED_EDGE ( 'NONE', *, *, #18359, .F. ) ;
#37543=EDGE_CURVE ( 'NONE', #28556, #9089, #12505, .T. ) ;
#37545=CARTESIAN_POINT ( 'NONE',  ( -10.47804177580193041, 33.28010392086039104, 11.00000000000000000 ) ) ;
#37547=AXIS2_PLACEMENT_3D ( 'NONE', #10396, #32745, #10800 ) ;
#37549=ORIENTED_EDGE ( 'NONE', *, *, #8377, .T. ) ;
#37551=CARTESIAN_POINT ( 'NONE',  ( -4.524139159579194214, 31.43208625488816566, 10.50000000000000711 ) ) ;
#37554=LINE ( 'NONE', #12959, #33372 ) ;
#37555=CARTESIAN_POINT ( 'NONE',  ( -2.525645716490712012, 8.212903943950955465, 7.000000000000000000 ) ) ;
#37557=EDGE_LOOP ( 'NONE', ( #34529, #23755, #13385, #40098 ) ) ;
#37560=EDGE_CURVE ( 'NONE', #6246, #13267, #31311, .T. ) ;
#37562=DIRECTION ( 'NONE',  ( -0.5720614028176850274, 0.4156269377774632345, -0.7071067811865411334 ) ) ;
#37565=LINE ( 'NONE', #21718, #16791 ) ;
#37570=CARTESIAN_POINT ( 'NONE',  ( 7.713869163865845202, 10.18146832927074641, 10.49999999999999822 ) ) ;
#37571=DIRECTION ( 'NONE',  ( -0.1045284632676422437, 0.9945218953682746221, 0.000000000000000000 ) ) ;
#37574=CARTESIAN_POINT ( 'NONE',  ( -12.47973198054747890, 14.17771442864374443, 7.339470489435493405 ) ) ;
#37575=CARTESIAN_POINT ( 'NONE',  ( 5.167086843766643511, 44.40436517110171621, 11.00000000000000000 ) ) ;
#37577=AXIS2_PLACEMENT_3D ( 'NONE', #5224, #23910, #24505 ) ;
#37578=DIRECTION ( 'NONE',  ( 0.000000000000000000, 0.000000000000000000, 1.000000000000000000 ) ) ;
#37581=DIRECTION ( 'NONE',  ( -0.8090169943749497827, -0.5877852522924698064, 0.000000000000000000 ) ) ;
#37582=EDGE_CURVE ( 'NONE', #34828, #26924, #32382, .T. ) ;
#37593=VERTEX_POINT ( 'NONE', #30932 ) ;
#37595=EDGE_CURVE ( 'NONE', #13490, #28177, #10556, .T. ) ;
#37596=CARTESIAN_POINT ( 'NONE',  ( 9.997483185316555776, 21.95197631500757041, 10.50000000000000355 ) ) ;
#37599=CARTESIAN_POINT ( 'NONE',  ( 5.184280209938512129, 31.68549066217151022, 10.50000000000000000 ) ) ;
#37600=VERTEX_POINT ( 'NONE', #37226 ) ;
#37601=CARTESIAN_POINT ( 'NONE',  ( 3.601976756503082910, 7.958898870085707067, 10.68306085400107186 ) ) ;
#37604=FACE_OUTER_BOUND ( 'NONE', #7291, .T. ) ;
#37607=CIRCLE ( 'NONE', #6448, 0.5000000000000013323 ) ;
#37608=ADVANCED_FACE ( 'NONE', ( #34180 ), #35194, .T. ) ;
#37609=EDGE_CURVE ( 'NONE', #9898, #22876, #30016, .T. ) ;
#37613=CARTESIAN_POINT ( 'NONE',  ( -10.10646936306323518, 32.94553861768095970, 11.00000000000000000 ) ) ;
#37619=ORIENTED_EDGE ( 'NONE', *, *, #25976, .T. ) ;
#37622=CARTESIAN_POINT ( 'NONE',  ( -6.535904741238326210, 35.95058573176953587, 10.76099332938163400 ) ) ;
#37626=DIRECTION ( 'NONE',  ( -0.9335804264971983013, -0.3583679495453093722, 6.429803227988806504E-16 ) ) ;
#37630=CARTESIAN_POINT ( 'NONE',  ( 3.597409820281487480, 14.42008525284347087, 9.000000000000001776 ) ) ;
#37631=VERTEX_POINT ( 'NONE', #24234 ) ;
#37633=EDGE_CURVE ( 'NONE', #5601, #6401, #37421, .T. ) ;
#37634=ORIENTED_EDGE ( 'NONE', *, *, #86, .F. ) ;
#37639=ORIENTED_EDGE ( 'NONE', *, *, #20865, .F. ) ;
#37644=DIRECTION ( 'NONE',  ( 1.000000000000000000, 0.000000000000000000, 0.000000000000000000 ) ) ;
#37645=AXIS2_PLACEMENT_3D ( 'NONE', #2228, #14613, #24149 ) ;
#37650=CARTESIAN_POINT ( 'NONE',  ( -0.4999999999999950040, -6.123233995736694545E-17, 11.00000000000000000 ) ) ;
#37651=EDGE_CURVE ( 'NONE', #26489, #39789, #36633, .T. ) ;
#37653=VERTEX_POINT ( 'NONE', #15890 ) ;
#37656=CARTESIAN_POINT ( 'NONE',  ( 10.14084140100273146, 32.97648733965218071, 10.49999999999999822 ) ) ;
#37658=ORIENTED_EDGE ( 'NONE', *, *, #4814, .F. ) ;
#37660=CIRCLE ( 'NONE', #6535, 1.000000000000005329 ) ;
#37663=CARTESIAN_POINT ( 'NONE',  ( 12.80736835487433289, 15.68301270189216545, 7.000000000000000000 ) ) ;
#37665=FACE_OUTER_BOUND ( 'NONE', #19617, .T. ) ;
#37666=ORIENTED_EDGE ( 'NONE', *, *, #1427, .F. ) ;
#37669=DIRECTION ( 'NONE',  ( 0.000000000000000000, 0.000000000000000000, 1.000000000000000000 ) ) ;
#37671=EDGE_LOOP ( 'NONE', ( #17326, #20612, #38478, #23052 ) ) ;
#37673=CARTESIAN_POINT ( 'NONE',  ( -3.992867117591420545, 8.524771480177605554, 7.499999999999997335 ) ) ;
#37675=FACE_OUTER_BOUND ( 'NONE', #27713, .T. ) ;
#37678=ADVANCED_FACE ( 'NONE', ( #25618 ), #1050, .F. ) ;
#37681=EDGE_CURVE ( 'NONE', #16160, #40105, #21597, .T. ) ;
#37683=AXIS2_PLACEMENT_3D ( 'NONE', #16971, #10670, #38700 ) ;
#37684=ORIENTED_EDGE ( 'NONE', *, *, #20314, .F. ) ;
#37686=FACE_OUTER_BOUND ( 'NONE', #289, .T. ) ;
#37689=AXIS2_PLACEMENT_3D ( 'NONE', #31061, #30664, #39990 ) ;
#37691=CARTESIAN_POINT ( 'NONE',  ( -11.46110488303199126, 32.14680882400074324, 10.68306159501106656 ) ) ;
#37692=CARTESIAN_POINT ( 'NONE',  ( 12.53024597560964537, 27.62278594035691626, 9.500000000000000000 ) ) ;
#37694=CARTESIAN_POINT ( 'NONE',  ( -7.766013557953296953, 28.81973365084997951, 10.00000000000000000 ) ) ;
#37695=CARTESIAN_POINT ( 'NONE',  ( 14.60528968261095173, 20.46216805729368460, 10.94387467463493380 ) ) ;
#37697=EDGE_CURVE ( 'NONE', #29830, #11555, #39115, .T. ) ;
#37698=CYLINDRICAL_SURFACE ( 'NONE', #39138, 0.5000000000000004441 ) ;
#37699=DIRECTION ( 'NONE',  ( 0.7431448254773953543, 0.6691306063588570163, 0.000000000000000000 ) ) ;
#37700=DIRECTION ( 'NONE',  ( -0.000000000000000000, -0.000000000000000000, -1.000000000000000000 ) ) ;
#37701=EDGE_CURVE ( 'NONE', #22687, #7627, #25419, .T. ) ;
#37703=DIRECTION ( 'NONE',  ( -0.000000000000000000, -0.000000000000000000, -1.000000000000000000 ) ) ;
#37704=ORIENTED_EDGE ( 'NONE', *, *, #16957, .T. ) ;
#37705=VECTOR ( 'NONE', #30512, 1000.000000000000114 ) ;
#37709=VECTOR ( 'NONE', #3860, 1000.000000000000000 ) ;
#37713=ORIENTED_EDGE ( 'NONE', *, *, #33660, .T. ) ;
#37715=VERTEX_POINT ( 'NONE', #19133 ) ;
#37722=VERTEX_POINT ( 'NONE', #3689 ) ;
#37724=DIRECTION ( 'NONE',  ( -1.000000000000000000, 0.000000000000000000, 0.000000000000000000 ) ) ;
#37728=EDGE_CURVE ( 'NONE', #9701, #12080, #28671, .T. ) ;
#37730=VERTEX_POINT ( 'NONE', #13028 ) ;
#37731=ADVANCED_FACE ( 'NONE', ( #9794 ), #31724, .T. ) ;
#37733=DIRECTION ( 'NONE',  ( -0.000000000000000000, -0.000000000000000000, -1.000000000000000000 ) ) ;
#37737=CIRCLE ( 'NONE', #8534, 6.000000000000012434 ) ;
#37738=CIRCLE ( 'NONE', #20229, 0.5000000000000004441 ) ;
#37741=CARTESIAN_POINT ( 'NONE',  ( -13.05736835487441994, 16.11602540378456183, 7.499999999999993783 ) ) ;
#37742=CARTESIAN_POINT ( 'NONE',  ( -0.6666666666666682950, 37.00000000000000711, 10.83333333333333215 ) ) ;
#37743=FACE_OUTER_BOUND ( 'NONE', #29876, .T. ) ;
#37746=CARTESIAN_POINT ( 'NONE',  ( 8.271785691010562047, 10.26421291652873968, 10.94611345180490680 ) ) ;
#37747=CARTESIAN_POINT ( 'NONE',  ( -6.811226782241546651, 35.33967249274200384, 7.500000000000000888 ) ) ;
#37749=DIRECTION ( 'NONE',  ( 0.7431448254773862505, -0.6691306063588670083, -0.000000000000000000 ) ) ;
#37750=DIRECTION ( 'NONE',  ( -0.5254827454987616164, -0.4731467892558160471, -0.7071067811865446862 ) ) ;
#37751=DIRECTION ( 'NONE',  ( 0.000000000000000000, 0.000000000000000000, 1.000000000000000000 ) ) ;
#37753=CARTESIAN_POINT ( 'NONE',  ( 3.503793317224327186, 8.420815634768674229, 11.00000000000000000 ) ) ;
#37754=VERTEX_POINT ( 'NONE', #38223 ) ;
#37758=DIRECTION ( 'NONE',  ( -0.000000000000000000, -0.000000000000000000, -1.000000000000000000 ) ) ;
#37759=ADVANCED_FACE ( 'NONE', ( #647 ), #34980, .F. ) ;
#37767=CARTESIAN_POINT ( 'NONE',  ( 14.02836544648986994, 27.77630492435572407, 10.49999999999999822 ) ) ;
#37771=CARTESIAN_POINT ( 'NONE',  ( 14.94248101481482038, 21.43223609974773325, 10.68306085400105232 ) ) ;
#37772=ORIENTED_EDGE ( 'NONE', *, *, #35133, .F. ) ;
#37774=FACE_OUTER_BOUND ( 'NONE', #1696, .T. ) ;
#37775=CIRCLE ( 'NONE', #20268, 15.00000000000000000 ) ;
#37776=CARTESIAN_POINT ( 'NONE',  ( 22.42900687741999732, 24.35462947583786075, 11.00000000000000000 ) ) ;
#37777=ORIENTED_EDGE ( 'NONE', *, *, #210, .F. ) ;
#37779=CARTESIAN_POINT ( 'NONE',  ( -8.796116341590805021, 23.42450908139092647, 9.000000000000001776 ) ) ;
#37780=VERTEX_POINT ( 'NONE', #38017 ) ;
#37782=AXIS2_PLACEMENT_3D ( 'NONE', #31373, #11895, #21235 ) ;
#37789=ORIENTED_EDGE ( 'NONE', *, *, #3200, .T. ) ;
#37791=CARTESIAN_POINT ( 'NONE',  ( 12.30253635578773341, 13.91734747557917728, 7.102474990965858659 ) ) ;
#37792=LINE ( 'NONE', #31303, #10430 ) ;
#37794=AXIS2_PLACEMENT_3D ( 'NONE', #30162, #11277, #23661 ) ;
#37796=ORIENTED_EDGE ( 'NONE', *, *, #22897, .T. ) ;
#37797=EDGE_CURVE ( 'NONE', #11320, #25929, #1253, .T. ) ;
#37798=TOROIDAL_SURFACE ( 'NONE', #13790, 1.000000000000000000, 0.5000000000000000000 ) ;
#37800=DIRECTION ( 'NONE',  ( 0.2079116908177533474, -0.9781476007338067991, 0.000000000000000000 ) ) ;
#37801=CARTESIAN_POINT ( 'NONE',  ( 1.160606217761757097, 37.45558278363897386, 7.202682876670053247 ) ) ;
#37804=AXIS2_PLACEMENT_3D ( 'NONE', #28875, #31919, #13226 ) ;
#37807=EDGE_CURVE ( 'NONE', #26812, #22931, #22571, .T. ) ;
#37816=DIRECTION ( 'NONE',  ( 0.6691306063588569053, -0.7431448254773954654, 0.000000000000000000 ) ) ;
#37819=LINE ( 'NONE', #7332, #1859 ) ;
#37820=CARTESIAN_POINT ( 'NONE',  ( 14.52509594610761923, 21.97885917798724975, 10.50000000000000355 ) ) ;
#37823=ORIENTED_EDGE ( 'NONE', *, *, #35953, .F. ) ;
#37827=EDGE_CURVE ( 'NONE', #16446, #22627, #7099, .T. ) ;
#37830=EDGE_CURVE ( 'NONE', #18426, #19145, #4075, .T. ) ;
#37831=CARTESIAN_POINT ( 'NONE',  ( 9.201548168576595188, 26.54122646004460861, 10.50000000000000533 ) ) ;
#37835=CARTESIAN_POINT ( 'NONE',  ( -15.34554945454190467, 9.014796822355112482, 10.00000000000000000 ) ) ;
#37841=DIRECTION ( 'NONE',  ( 0.000000000000000000, 0.000000000000000000, 1.000000000000000000 ) ) ;
#37844=ORIENTED_EDGE ( 'NONE', *, *, #25976, .F. ) ;
#37848=CYLINDRICAL_SURFACE ( 'NONE', #4921, 0.5000000000000004441 ) ;
#37850=B_SPLINE_CURVE_WITH_KNOTS ( 'NONE', 3,
 ( #9143, #12981, #6677, #37173, #201, #33931 ),
 .UNSPECIFIED., .F., .F.,
 ( 4, 2, 4 ),
 ( 0.000000000000000000, 0.5000000000000000000, 1.000000000000000000 ),
 .UNSPECIFIED. ) ;
#37851=ORIENTED_EDGE ( 'NONE', *, *, #13593, .F. ) ;
#37859=AXIS2_PLACEMENT_3D ( 'NONE', #16007, #371, #25535 ) ;
#37863=DIRECTION ( 'NONE',  ( 0.000000000000000000, 0.000000000000000000, -1.000000000000000000 ) ) ;
#37865=EDGE_LOOP ( 'NONE', ( #34534, #39576, #7438, #12043, #29237 ) ) ;
#37868=CARTESIAN_POINT ( 'NONE',  ( 7.249670636309310190, 35.63227325353309283, 7.102474990965859547 ) ) ;
#37869=CARTESIAN_POINT ( 'NONE',  ( -10.51560177358055803, 33.07492339674077186, 10.49999999999999822 ) ) ;
#37870=EDGE_LOOP ( 'NONE', ( #6501, #36668, #1925 ) ) ;
#37873=CIRCLE ( 'NONE', #20374, 0.5000000000000004441 ) ;
#37876=EDGE_CURVE ( 'NONE', #25343, #18018, #34574, .T. ) ;
#37879=DIRECTION ( 'NONE',  ( 1.000000000000000000, 0.000000000000000000, 0.000000000000000000 ) ) ;
#37880=ORIENTED_EDGE ( 'NONE', *, *, #10113, .F. ) ;
#37881=LINE ( 'NONE', #119, #21025 ) ;
#37883=CARTESIAN_POINT ( 'NONE',  ( -11.28725060478854303, 31.99026972875184427, 10.94387467463334396 ) ) ;
#37884=DIRECTION ( 'NONE',  ( -0.000000000000000000, -0.000000000000000000, -1.000000000000000000 ) ) ;
#37886=PLANE ( 'NONE',  #36050 ) ;
#37889=DIRECTION ( 'NONE',  ( 0.9781476007338067991, 0.2079116908177533751, 0.000000000000000000 ) ) ;
#37891=DIRECTION ( 'NONE',  ( -0.4067366430757888840, 0.9135454576426058626, 0.000000000000000000 ) ) ;
#37892=PLANE ( 'NONE',  #31984 ) ;
#37896=CARTESIAN_POINT ( 'NONE',  ( -6.913051850451354952, 35.81219556108709412, 7.382773698552463237 ) ) ;
#37899=CARTESIAN_POINT ( 'NONE',  ( 2.538198952020652044, 7.704401919100519081, 10.49999999999999822 ) ) ;
#37900=AXIS2_PLACEMENT_3D ( 'NONE', #34903, #31651, #26358 ) ;
#37901=CARTESIAN_POINT ( 'NONE',  ( 13.30684945990800649, 15.76689945427723138, 10.49999999999999822 ) ) ;
#37902=EDGE_CURVE ( 'NONE', #3653, #16261, #17061, .T. ) ;
#37909=ORIENTED_EDGE ( 'NONE', *, *, #23072, .T. ) ;
#37910=LINE ( 'NONE', #741, #6877 ) ;
#37918=ORIENTED_EDGE ( 'NONE', *, *, #30628, .T. ) ;
#37922=ORIENTED_EDGE ( 'NONE', *, *, #6409, .T. ) ;
#37926=ORIENTED_EDGE ( 'NONE', *, *, #37150, .T. ) ;
#37927=CARTESIAN_POINT ( 'NONE',  ( 11.11016527260166420, 31.83082137946473367, 7.000000000000000000 ) ) ;
#37928=DIRECTION ( 'NONE',  ( 1.000000000000000000, 0.000000000000000000, 0.000000000000000000 ) ) ;
#37929=ADVANCED_FACE ( 'NONE', ( #5295 ), #11002, .T. ) ;
#37930=EDGE_CURVE ( 'NONE', #22181, #9989, #1449, .T. ) ;
#37932=EDGE_CURVE ( 'NONE', #26220, #26306, #17101, .T. ) ;
#37934=VERTEX_POINT ( 'NONE', #11601 ) ;
#37936=PLANE ( 'NONE',  #37859 ) ;
#37938=B_SPLINE_CURVE_WITH_KNOTS ( 'NONE', 3,
 ( #19878, #29616, #14584, #11137, #8284, #17650 ),
 .UNSPECIFIED., .F., .F.,
 ( 4, 2, 4 ),
 ( 0.000000000000000000, 0.5000000000000000000, 1.000000000000000000 ),
 .UNSPECIFIED. ) ;
#37939=CARTESIAN_POINT ( 'NONE',  ( 5.644276917315718123, 36.40655018617690786, 10.63089969389957368 ) ) ;
#37940=ORIENTED_EDGE ( 'NONE', *, *, #39089, .T. ) ;
#37942=CARTESIAN_POINT ( 'NONE',  ( 8.195318570657093460, 10.36946087849375076, 11.00000000000000000 ) ) ;
#37948=CARTESIAN_POINT ( 'NONE',  ( 10.72918489117954088, 32.98258515686300996, 7.000000000000000000 ) ) ;
#37950=DIRECTION ( 'NONE',  ( -0.000000000000000000, -0.000000000000000000, 1.000000000000000000 ) ) ;
#37952=ORIENTED_EDGE ( 'NONE', *, *, #36703, .F. ) ;
#37954=LINE ( 'NONE', #34708, #19386 ) ;
#37956=EDGE_CURVE ( 'NONE', #22041, #9605, #7936, .T. ) ;
#37958=CARTESIAN_POINT ( 'NONE',  ( -0.9999999999999993339, 33.00000000000000000, 10.50000000000000178 ) ) ;
#37961=CARTESIAN_POINT ( 'NONE',  ( 6.557822374958316658, 35.99981354310111215, 10.49999999999999822 ) ) ;
#37970=VECTOR ( 'NONE', #31859, 1000.000000000000114 ) ;
#37971=CARTESIAN_POINT ( 'NONE',  ( 14.97986028244560508, 21.52226669793674318, 10.49999999999999822 ) ) ;
#37972=VERTEX_POINT ( 'NONE', #17707 ) ;
#37974=CARTESIAN_POINT ( 'NONE',  ( 14.63635198741554788, 25.78286467897733303, 7.000000000000000000 ) ) ;
#37975=DIRECTION ( 'NONE',  ( -0.000000000000000000, -0.000000000000000000, -1.000000000000000000 ) ) ;
#37977=AXIS2_PLACEMENT_3D ( 'NONE', #1952, #13924, #14125 ) ;
#37982=EDGE_CURVE ( 'NONE', #481, #4731, #35380, .T. ) ;
#37983=VECTOR ( 'NONE', #27306, 1000.000000000000000 ) ;
#37984=CONICAL_SURFACE ( 'NONE', #375, 1.000000000000013101, 0.7853981633974579379 ) ;
#37991=DIRECTION ( 'NONE',  ( -0.000000000000000000, -0.000000000000000000, -1.000000000000000000 ) ) ;
#37994=LINE ( 'NONE', #10364, #35996 ) ;
#37996=CARTESIAN_POINT ( 'NONE',  ( -4.096822963000303019, 8.035697679810709815, 10.50000000000000533 ) ) ;
#37999=VERTEX_POINT ( 'NONE', #29478 ) ;
#38001=DIRECTION ( 'NONE',  ( 0.3535533905932766174, 0.6123724356957975790, -0.7071067811865433539 ) ) ;
#38003=CARTESIAN_POINT ( 'NONE',  ( 10.44103466624280685, 32.57396620494213124, 7.000000000000000000 ) ) ;
#38004=VERTEX_POINT ( 'NONE', #17305 ) ;
#38005=CIRCLE ( 'NONE', #10783, 0.5000000000000004441 ) ;
#38007=AXIS2_PLACEMENT_3D ( 'NONE', #18832, #2994, #31220 ) ;
#38011=EDGE_LOOP ( 'NONE', ( #9201, #28672, #17347, #13235 ) ) ;
#38012=ORIENTED_EDGE ( 'NONE', *, *, #9790, .T. ) ;
#38017=CARTESIAN_POINT ( 'NONE',  ( 9.593266739736579396, 18.11602540378440196, 10.50000000000000000 ) ) ;
#38018=ORIENTED_EDGE ( 'NONE', *, *, #36090, .F. ) ;
#38020=CARTESIAN_POINT ( 'NONE',  ( 6.572794801194151049, 16.58182897866491956, 9.000000000000001776 ) ) ;
#38021=DIRECTION ( 'NONE',  ( 1.000000000000000000, 0.000000000000000000, 0.000000000000000000 ) ) ;
#38022=EDGE_LOOP ( 'NONE', ( #16005, #31442, #30459, #24842, #12936, #35573, #12252 ) ) ;
#38025=ORIENTED_EDGE ( 'NONE', *, *, #18834, .T. ) ;
#38029=EDGE_CURVE ( 'NONE', #42, #18984, #24120, .T. ) ;
#38030=ORIENTED_EDGE ( 'NONE', *, *, #10865, .F. ) ;
#38032=CONICAL_SURFACE ( 'NONE', #22444, 0.4999999999999980571, 0.7853981633974552734 ) ;
#38033=DIRECTION ( 'NONE',  ( -0.6691306063588570163, 0.7431448254773952433, 0.000000000000000000 ) ) ;
#38035=AXIS2_PLACEMENT_3D ( 'NONE', #29971, #26726, #14938 ) ;
#38036=DIRECTION ( 'NONE',  ( 0.5000000000000038858, 0.8660254037844364872, -0.000000000000000000 ) ) ;
#38039=CYLINDRICAL_SURFACE ( 'NONE', #1997, 0.5000000000000004441 ) ;
#38045=DIRECTION ( 'NONE',  ( 0.9781476007338042455, -0.2079116908177664758, 0.000000000000000000 ) ) ;
#38050=EDGE_CURVE ( 'NONE', #22627, #22029, #8548, .T. ) ;
#38051=CARTESIAN_POINT ( 'NONE',  ( 10.75008043808897185, 32.97797437800703335, 10.49999999999999822 ) ) ;
#38055=DIRECTION ( 'NONE',  ( 1.000000000000000000, -3.469446951953598806E-15, 0.000000000000000000 ) ) ;
#38056=ORIENTED_EDGE ( 'NONE', *, *, #15225, .F. ) ;
#38060=CARTESIAN_POINT ( 'NONE',  ( 12.41469063302487363, 14.32475803611739273, 10.49999999999999822 ) ) ;
#38061=CIRCLE ( 'NONE', #17986, 0.9999999999999988898 ) ;
#38062=ORIENTED_EDGE ( 'NONE', *, *, #13443, .F. ) ;
#38065=FACE_OUTER_BOUND ( 'NONE', #3086, .T. ) ;
#38069=CARTESIAN_POINT ( 'NONE',  ( 13.94482798346721353, 26.50521816028912525, 7.000000000000000000 ) ) ;
#38070=CARTESIAN_POINT ( 'NONE',  ( 10.72918489117958174, 32.98258515686296732, 7.499999999999997335 ) ) ;
#38071=ORIENTED_EDGE ( 'NONE', *, *, #37427, .T. ) ;
#38075=ORIENTED_EDGE ( 'NONE', *, *, #8309, .T. ) ;
#38078=CARTESIAN_POINT ( 'NONE',  ( -12.67417846324126174, 14.47720745114824226, 7.000000000000000000 ) ) ;
#38079=EDGE_CURVE ( 'NONE', #28707, #36352, #21506, .T. ) ;
#38080=CARTESIAN_POINT ( 'NONE',  ( -10.36702044712415116, 31.16169077310601665, 9.500000000000000000 ) ) ;
#38082=AXIS2_PLACEMENT_3D ( 'NONE', #550, #22079, #28575 ) ;
#38083=CARTESIAN_POINT ( 'NONE',  ( -11.48173768534043404, 32.16538668264409040, 10.59344404201838152 ) ) ;
#38086=ORIENTED_EDGE ( 'NONE', *, *, #33717, .T. ) ;
#38087=CARTESIAN_POINT ( 'NONE',  ( 5.947717410344607103, 34.62949535663720724, 9.500000000000000000 ) ) ;
#38088=DIRECTION ( 'NONE',  ( 0.000000000000000000, -0.000000000000000000, -1.000000000000000000 ) ) ;
#38090=VECTOR ( 'NONE', #1161, 1000.000000000000000 ) ;
#38091=FACE_OUTER_BOUND ( 'NONE', #34617, .T. ) ;
#38094=AXIS2_PLACEMENT_3D ( 'NONE', #3368, #34454, #5825 ) ;
#38095=FACE_OUTER_BOUND ( 'NONE', #33989, .T. ) ;
#38096=VERTEX_POINT ( 'NONE', #7536 ) ;
#38098=DIRECTION ( 'NONE',  ( 1.000000000000000000, 0.000000000000000000, 0.000000000000000000 ) ) ;
#38099=FACE_OUTER_BOUND ( 'NONE', #35603, .T. ) ;
#38100=ADVANCED_FACE ( 'NONE', ( #14645 ), #19939, .F. ) ;
#38102=ADVANCED_FACE ( 'NONE', ( #39618 ), #9353, .T. ) ;
#38103=PLANE ( 'NONE',  #30853 ) ;
#38107=VERTEX_POINT ( 'NONE', #9348 ) ;
#38109=CARTESIAN_POINT ( 'NONE',  ( 14.26729173199937861, 26.60999298350824560, 10.87262190629280845 ) ) ;
#38115=EDGE_LOOP ( 'NONE', ( #24623, #6437, #25033, #15172 ) ) ;
#38119=ORIENTED_EDGE ( 'NONE', *, *, #25740, .F. ) ;
#38122=AXIS2_PLACEMENT_3D ( 'NONE', #9653, #31180, #15340 ) ;
#38124=ORIENTED_EDGE ( 'NONE', *, *, #33997, .T. ) ;
#38125=LINE ( 'NONE', #19236, #38191 ) ;
#38127=CIRCLE ( 'NONE', #23199, 0.5000000000000004441 ) ;
#38131=AXIS2_PLACEMENT_3D ( 'NONE', #37479, #29481, #25470 ) ;
#38132=ORIENTED_EDGE ( 'NONE', *, *, #35993, .T. ) ;
#38133=ORIENTED_EDGE ( 'NONE', *, *, #26435, .F. ) ;
#38137=ORIENTED_EDGE ( 'NONE', *, *, #25292, .F. ) ;
#38139=FACE_OUTER_BOUND ( 'NONE', #8803, .T. ) ;
#38140=CARTESIAN_POINT ( 'NONE',  ( -4.141337746071314996, 43.73298676078094616, 10.00000000000000000 ) ) ;
#38142=PLANE ( 'NONE',  #3323 ) ;
#38143=CARTESIAN_POINT ( 'NONE',  ( -3.295881626406750975, 9.398963235502531433, 10.50000000000000000 ) ) ;
#38144=DIRECTION ( 'NONE',  ( 0.1277282058446098378, 0.8064441531181054668, 0.5773502691896305050 ) ) ;
#38147=CARTESIAN_POINT ( 'NONE',  ( -9.331903152615899089, 11.35703883385581037, 11.00000000000000000 ) ) ;
#38148=AXIS2_PLACEMENT_3D ( 'NONE', #34624, #6777, #19179 ) ;
#38151=DIRECTION ( 'NONE',  ( -0.7275037805840933736, 0.3706816908110012188, 0.5773502691896389427 ) ) ;
#38154=LINE ( 'NONE', #34914, #34726 ) ;
#38156=CIRCLE ( 'NONE', #13499, 1.000000000000000888 ) ;
#38159=EDGE_CURVE ( 'NONE', #29611, #16505, #8748, .T. ) ;
#38168=ORIENTED_EDGE ( 'NONE', *, *, #33215, .F. ) ;
#38170=ORIENTED_EDGE ( 'NONE', *, *, #4307, .F. ) ;
#38174=DIRECTION ( 'NONE',  ( 0.5000000000000039968, 0.8660254037844363761, 0.000000000000000000 ) ) ;
#38175=LINE ( 'NONE', #28428, #24554 ) ;
#38176=ORIENTED_EDGE ( 'NONE', *, *, #37430, .F. ) ;
#38178=DIRECTION ( 'NONE',  ( -0.4067366430757888840, 0.9135454576426058626, 0.000000000000000000 ) ) ;
#38179=EDGE_CURVE ( 'NONE', #40188, #14045, #7230, .T. ) ;
#38180=ORIENTED_EDGE ( 'NONE', *, *, #17341, .T. ) ;
#38182=AXIS2_PLACEMENT_3D ( 'NONE', #28614, #9338, #22507 ) ;
#38183=EDGE_CURVE ( 'NONE', #24444, #18928, #31084, .T. ) ;
#38187=AXIS2_PLACEMENT_3D ( 'NONE', #27303, #5166, #11466 ) ;
#38188=DIRECTION ( 'NONE',  ( -0.3090169943749434545, 0.9510565162951548634, 0.000000000000000000 ) ) ;
#38189=DIRECTION ( 'NONE',  ( 0.9135454576426059736, 0.4067366430757888285, 0.000000000000000000 ) ) ;
#38191=VECTOR ( 'NONE', #3797, 999.9999999999997726 ) ;
#38192=EDGE_CURVE ( 'NONE', #27233, #27267, #36576, .T. ) ;
#38194=VERTEX_POINT ( 'NONE', #21138 ) ;
#38195=FILL_AREA_STYLE ('',( #19910 ) ) ;
#38196=DIRECTION ( 'NONE',  ( -0.000000000000000000, 0.000000000000000000, -1.000000000000000000 ) ) ;
#38197=DIRECTION ( 'NONE',  ( 0.4999999999999919509, -0.8660254037844432595, 0.000000000000000000 ) ) ;
#38201=EDGE_LOOP ( 'NONE', ( #4347, #38170, #1957 ) ) ;
#38206=EDGE_CURVE ( 'NONE', #33852, #36571, #5929, .T. ) ;
#38208=ADVANCED_FACE ( 'NONE', ( #36381 ), #32566, .T. ) ;
#38210=ORIENTED_EDGE ( 'NONE', *, *, #19815, .F. ) ;
#38215=DIRECTION ( 'NONE',  ( -0.9945218953682729568, 0.1045284632676569958, 0.000000000000000000 ) ) ;
#38216=ORIENTED_EDGE ( 'NONE', *, *, #23647, .T. ) ;
#38217=ORIENTED_EDGE ( 'NONE', *, *, #21800, .T. ) ;
#38218=AXIS2_PLACEMENT_3D ( 'NONE', #31542, #3707, #22385 ) ;
#38220=CARTESIAN_POINT ( 'NONE',  ( -18.91388186588683240, 35.25980436007201035, 10.00000000000000000 ) ) ;
#38223=CARTESIAN_POINT ( 'NONE',  ( -10.44103466624267540, 32.57396620494226624, 11.00000000000000000 ) ) ;
#38224=ORIENTED_EDGE ( 'NONE', *, *, #40163, .T. ) ;
#38226=CARTESIAN_POINT ( 'NONE',  ( 8.118377661053333583, 10.47536095541699197, 11.00000000000000000 ) ) ;
#38227=DIRECTION ( 'NONE',  ( -1.000000000000000000, 0.000000000000000000, 0.000000000000000000 ) ) ;
#38228=ORIENTED_EDGE ( 'NONE', *, *, #32101, .F. ) ;
#38230=DIRECTION ( 'NONE',  ( -0.9135454576426059736, -0.4067366430757887730, 0.000000000000000000 ) ) ;
#38231=EDGE_CURVE ( 'NONE', #38004, #25412, #8948, .T. ) ;
#38232=ORIENTED_EDGE ( 'NONE', *, *, #23281, .T. ) ;
#38236=EDGE_CURVE ( 'NONE', #14728, #17047, #2851, .T. ) ;
#38237=ORIENTED_EDGE ( 'NONE', *, *, #6469, .F. ) ;
#38241=CIRCLE ( 'NONE', #18784, 6.000000000000003553 ) ;
#38243=DIRECTION ( 'NONE',  ( 1.000000000000000000, 0.000000000000000000, 0.000000000000000000 ) ) ;
#38244=CIRCLE ( 'NONE', #29172, 0.5000000000000011102 ) ;
#38251=ORIENTED_EDGE ( 'NONE', *, *, #24420, .T. ) ;
#38253=EDGE_LOOP ( 'NONE', ( #11218, #6464, #39214, #34220 ) ) ;
#38258=VERTEX_POINT ( 'NONE', #27831 ) ;
#38260=EDGE_CURVE ( 'NONE', #21617, #36923, #202, .T. ) ;
#38262=ORIENTED_EDGE ( 'NONE', *, *, #33904, .F. ) ;
#38264=CARTESIAN_POINT ( 'NONE',  ( 8.118377661053324701, 10.47536095541698486, 7.000000000000000000 ) ) ;
#38266=LINE ( 'NONE', #29123, #7467 ) ;
#38267=VECTOR ( 'NONE', #17082, 1000.000000000000000 ) ;
#38268=ORIENTED_EDGE ( 'NONE', *, *, #5617, .F. ) ;
#38273=ORIENTED_EDGE ( 'NONE', *, *, #5642, .F. ) ;
#38275=CARTESIAN_POINT ( 'NONE',  ( 13.30736835491658887, 15.59574623945385596, 10.49999999999999822 ) ) ;
#38277=VECTOR ( 'NONE', #9519, 1000.000000000000114 ) ;
#38278=ORIENTED_EDGE ( 'NONE', *, *, #12384, .F. ) ;
#38282=EDGE_LOOP ( 'NONE', ( #37851, #33154, #23958, #25605 ) ) ;
#38284=DIRECTION ( 'NONE',  ( 0.9510565162951504226, -0.3090169943749573322, -0.000000000000000000 ) ) ;
#38285=CARTESIAN_POINT ( 'NONE',  ( -8.339609403135952448, 11.87216320208451314, 9.500000000000000000 ) ) ;
#38286=EDGE_CURVE ( 'NONE', #32239, #36997, #28639, .T. ) ;
#38287=LINE ( 'NONE', #30105, #18475 ) ;
#38288=FACE_OUTER_BOUND ( 'NONE', #32284, .T. ) ;
#38289=DIRECTION ( 'NONE',  ( 0.4731467892558158250, -0.5254827454987615054, 0.7071067811865450192 ) ) ;
#38292=CARTESIAN_POINT ( 'NONE',  ( -6.643188263509865799, 35.96180620077112167, 10.49999999999999822 ) ) ;
#38295=AXIS2_PLACEMENT_3D ( 'NONE', #18218, #2768, #15161 ) ;
#38296=DIRECTION ( 'NONE',  ( -0.9135454576426059736, -0.4067366430757888285, 0.000000000000000000 ) ) ;
#38297=CARTESIAN_POINT ( 'NONE',  ( -12.30736835487443415, 14.81698729810790560, 11.00000000000000000 ) ) ;
#38299=PLANE ( 'NONE',  #18500 ) ;
#38300=VERTEX_POINT ( 'NONE', #18494 ) ;
#38303=EDGE_CURVE ( 'NONE', #27240, #2755, #18300, .T. ) ;
#38305=LINE ( 'NONE', #13313, #343 ) ;
#38307=VERTEX_POINT ( 'NONE', #27232 ) ;
#38309=VERTEX_POINT ( 'NONE', #7280 ) ;
#38317=ADVANCED_FACE ( 'NONE', ( #34332 ), #22164, .T. ) ;
#38320=AXIS2_PLACEMENT_3D ( 'NONE', #38087, #35453, #20218 ) ;
#38321=CARTESIAN_POINT ( 'NONE',  ( 9.441034666242805073, 32.57396620494213124, 7.000000000000000000 ) ) ;
#38323=ADVANCED_FACE ( 'NONE', ( #28827 ), #37375, .T. ) ;
#38325=ORIENTED_EDGE ( 'NONE', *, *, #15074, .F. ) ;
#38330=CYLINDRICAL_SURFACE ( 'NONE', #32979, 0.4999999999999999445 ) ;
#38331=VECTOR ( 'NONE', #6902, 1000.000000000000000 ) ;
#38335=VERTEX_POINT ( 'NONE', #34929 ) ;
#38336=EDGE_CURVE ( 'NONE', #36223, #30328, #19279, .T. ) ;
#38339=CARTESIAN_POINT ( 'NONE',  ( -1.653273178848927853E-15, 36.00000000000000711, 7.000000000000000000 ) ) ;
#38343=CARTESIAN_POINT ( 'NONE',  ( -14.99905852611806445, 22.33194247983213643, 7.000000000000000000 ) ) ;
#38344=CARTESIAN_POINT ( 'NONE',  ( 10.44103466624280685, 32.57396620494213124, 7.000000000000000000 ) ) ;
#38345=CARTESIAN_POINT ( 'NONE',  ( -22.84654430795398028, 26.73830628268968823, 10.00000000000000000 ) ) ;
#38346=DIRECTION ( 'NONE',  ( 1.000000000000000000, 0.000000000000000000, 0.000000000000000000 ) ) ;
#38347=CARTESIAN_POINT ( 'NONE',  ( 7.713869163865849643, 10.18146832927074996, 7.500000000000000888 ) ) ;
#38353=CARTESIAN_POINT ( 'NONE',  ( -0.4999999999999998890, 37.04625217320466390, 10.99999999999999645 ) ) ;
#38355=DIRECTION ( 'NONE',  ( -0.5000000000000039968, -0.8660254037844363761, 0.000000000000000000 ) ) ;
#38356=VECTOR ( 'NONE', #25348, 1000.000000000000000 ) ;
#38365=FACE_OUTER_BOUND ( 'NONE', #5946, .T. ) ;
#38366=CARTESIAN_POINT ( 'NONE',  ( 13.97557076678965693, 21.53386246193694475, 9.500000000000000000 ) ) ;
#38369=ORIENTED_EDGE ( 'NONE', *, *, #19282, .F. ) ;
#38372=DIRECTION ( 'NONE',  ( 1.000000000000000000, 0.000000000000000000, 0.000000000000000000 ) ) ;
#38373=EDGE_LOOP ( 'NONE', ( #28085, #31316, #28632, #31230, #26103 ) ) ;
#38375=CIRCLE ( 'NONE', #27989, 0.9999999999999991118 ) ;
#38376=CARTESIAN_POINT ( 'NONE',  ( -8.843266739736657556, 16.81698729810786830, 10.00000000000000000 ) ) ;
#38377=FACE_OUTER_BOUND ( 'NONE', #9354, .T. ) ;
#38378=ORIENTED_EDGE ( 'NONE', *, *, #662, .F. ) ;
#38384=VECTOR ( 'NONE', #17051, 1000.000000000000000 ) ;
#38386=EDGE_CURVE ( 'NONE', #22563, #28022, #35126, .T. ) ;
#38388=DIRECTION ( 'NONE',  ( -0.4067366430758009299, -0.9135454576426005335, -0.000000000000000000 ) ) ;
#38390=DIRECTION ( 'NONE',  ( 0.000000000000000000, 0.000000000000000000, -1.000000000000000000 ) ) ;
#38391=ORIENTED_EDGE ( 'NONE', *, *, #21800, .F. ) ;
#38392=( NAMED_UNIT ( * ) PLANE_ANGLE_UNIT ( ) SI_UNIT ( $, .RADIAN. ) );
#38395=CARTESIAN_POINT ( 'NONE',  ( -9.356056665764020508, 26.06569820189714903, 10.00000000000000000 ) ) ;
#38399=FACE_OUTER_BOUND ( 'NONE', #35624, .T. ) ;
#38400=CARTESIAN_POINT ( 'NONE',  ( -0.9461134518049056918, 37.26099332938166242, 10.49999999999999822 ) ) ;
#38403=LINE ( 'NONE', #32726, #17928 ) ;
#38404=ADVANCED_FACE ( 'NONE', ( #25573 ), #18925, .T. ) ;
#38409=ADVANCED_FACE ( 'NONE', ( #19681 ), #24981, .T. ) ;
#38410=AXIS2_PLACEMENT_3D ( 'NONE', #13540, #25928, #28981 ) ;
#38411=EDGE_CURVE ( 'NONE', #9357, #18134, #15041, .T. ) ;
#38412=FACE_OUTER_BOUND ( 'NONE', #37436, .T. ) ;
#38413=VERTEX_POINT ( 'NONE', #31675 ) ;
#38414=ORIENTED_EDGE ( 'NONE', *, *, #40194, .F. ) ;
#38419=AXIS2_PLACEMENT_3D ( 'NONE', #34819, #31774, #19992 ) ;
#38421=DIRECTION ( 'NONE',  ( -0.6691306063588569053, 0.7431448254773954654, 0.000000000000000000 ) ) ;
#38422=ORIENTED_EDGE ( 'NONE', *, *, #38231, .F. ) ;
#38425=CARTESIAN_POINT ( 'NONE',  ( -6.354454053420248272, 35.54304081427989814, 7.000000000000000000 ) ) ;
#38426=UNCERTAINTY_MEASURE_WITH_UNIT (LENGTH_MEASURE( 1.000000000000000082E-05 ), #7912, 'distance_accuracy_value', 'NONE');
#38427=VERTEX_POINT ( 'NONE', #16038 ) ;
#38429=CARTESIAN_POINT ( 'NONE',  ( -11.87435565298220652, 15.06698729810788961, 7.000000000000000000 ) ) ;
#38430=EDGE_LOOP ( 'NONE', ( #24592, #32350, #6633, #33620, #39523 ) ) ;
#38432=CARTESIAN_POINT ( 'NONE',  ( -2.525645716490710679, 8.212903943950959018, 7.000000000000000000 ) ) ;
#38433=AXIS2_PLACEMENT_3D ( 'NONE', #11431, #7566, #4930 ) ;
#38435=ORIENTED_EDGE ( 'NONE', *, *, #15204, .F. ) ;
#38439=ADVANCED_FACE ( 'NONE', ( #4035 ), #6679, .T. ) ;
#38441=ADVANCED_FACE ( 'NONE', ( #602 ), #25911, .T. ) ;
#38444=AXIS2_PLACEMENT_3D ( 'NONE', #17313, #30295, #7747 ) ;
#38445=CARTESIAN_POINT ( 'NONE',  ( -7.645071344821658954, 9.594463043616254794, 7.000000000000000000 ) ) ;
#38446=LINE ( 'NONE', #23411, #28796 ) ;
#38450=CARTESIAN_POINT ( 'NONE',  ( -11.11016527260153097, 31.83082137946489354, 11.00000000000000000 ) ) ;
#38451=EDGE_CURVE ( 'NONE', #7627, #30348, #1206, .T. ) ;
#38457=FACE_OUTER_BOUND ( 'NONE', #26695, .T. ) ;
#38462=ORIENTED_EDGE ( 'NONE', *, *, #14664, .F. ) ;
#38464=FACE_OUTER_BOUND ( 'NONE', #24247, .T. ) ;
#38466=CARTESIAN_POINT ( 'NONE',  ( 13.41748865645068811, 15.79359748466640667, 7.382773698552464126 ) ) ;
#38467=CONICAL_SURFACE ( 'NONE', #30037, 1.000000000000002665, 0.7853981633974509435 ) ;
#38468=ORIENTED_EDGE ( 'NONE', *, *, #9384, .F. ) ;
#38473=ORIENTED_EDGE ( 'NONE', *, *, #26393, .F. ) ;
#38475=DIRECTION ( 'NONE',  ( 0.9135454576426005335, -0.4067366430758009299, 0.000000000000000000 ) ) ;
#38476=AXIS2_PLACEMENT_3D ( 'NONE', #7369, #25658, #19981 ) ;
#38478=ORIENTED_EDGE ( 'NONE', *, *, #31236, .F. ) ;
#38482=VERTEX_POINT ( 'NONE', #10746 ) ;
#38485=AXIS2_PLACEMENT_3D ( 'NONE', #25305, #22646, #22245 ) ;
#38487=DIRECTION ( 'NONE',  ( -1.000000000000000000, 0.000000000000000000, 0.000000000000000000 ) ) ;
#38488=VECTOR ( 'NONE', #17011, 1000.000000000000000 ) ;
#38489=CARTESIAN_POINT ( 'NONE',  ( -11.56190694343544045, 31.61076883254029113, 10.49999999999999822 ) ) ;
#38490=DIRECTION ( 'NONE',  ( -0.000000000000000000, -0.000000000000000000, -1.000000000000000000 ) ) ;
#38491=DIRECTION ( 'NONE',  ( -0.000000000000000000, 0.000000000000000000, -1.000000000000000000 ) ) ;
#38493=CARTESIAN_POINT ( 'NONE',  ( -6.830039222088849726, 35.38192592444590900, 10.49999999999999822 ) ) ;
#38497=CARTESIAN_POINT ( 'NONE',  ( 14.36830325120613239, 20.48707633493482660, 11.00000000000000000 ) ) ;
#38500=DIRECTION ( 'NONE',  ( 0.7431448254773855844, -0.6691306063588678965, 0.000000000000000000 ) ) ;
#38501=EDGE_LOOP ( 'NONE', ( #5962, #22094, #35683, #1620 ) ) ;
#38506=DIRECTION ( 'NONE',  ( -0.000000000000000000, -0.000000000000000000, -1.000000000000000000 ) ) ;
#38508=EDGE_LOOP ( 'NONE', ( #36192, #38025, #35160, #27187 ) ) ;
#38510=ORIENTED_EDGE ( 'NONE', *, *, #21293, .F. ) ;
#38512=CARTESIAN_POINT ( 'NONE',  ( 3.596545519285629933, 7.984450832230633566, 10.76099332938164288 ) ) ;
#38526=VECTOR ( 'NONE', #17435, 1000.000000000000114 ) ;
#38531=LINE ( 'NONE', #32655, #26810 ) ;
#38535=EDGE_CURVE ( 'NONE', #26241, #37722, #10955, .T. ) ;
#38536=VERTEX_POINT ( 'NONE', #7487 ) ;
#38537=B_SPLINE_CURVE_WITH_KNOTS ( 'NONE', 3,
 ( #11927, #8879, #21268, #39553, #24511, #20879, #33281, #37109 ),
 .UNSPECIFIED., .F., .F.,
 ( 4, 2, 2, 4 ),
 ( 0.000000000000000000, 0.0004726692273637176397, 0.0007090038410455758904, 0.0009453384547274341953 ),
 .UNSPECIFIED. ) ;
#38538=PLANE ( 'NONE',  #21003 ) ;
#38540=CARTESIAN_POINT ( 'NONE',  ( 9.697889840765411051, 31.90483559858327212, 10.50000000000000000 ) ) ;
#38541=ORIENTED_EDGE ( 'NONE', *, *, #28985, .T. ) ;
#38542=AXIS2_PLACEMENT_3D ( 'NONE', #18128, #11627, #24407 ) ;
#38543=ADVANCED_FACE ( 'NONE', ( #26782 ), #23737, .T. ) ;
#38546=DIRECTION ( 'NONE',  ( -0.9510565162951497564, 0.3090169943749591086, 3.469446951953608667E-15 ) ) ;
#38547=ADVANCED_FACE ( 'NONE', ( #32897 ), #1810, .T. ) ;
#38548=CARTESIAN_POINT ( 'NONE',  ( 14.49025312501839657, 21.64735187953116480, 10.83333333333333393 ) ) ;
#38549=LINE ( 'NONE', #7057, #6742 ) ;
#38552=CARTESIAN_POINT ( 'NONE',  ( -4.940908595777636414, 35.94977745735568675, 11.00000000000000000 ) ) ;
#38555=CARTESIAN_POINT ( 'NONE',  ( 19.73557158514996601, 33.31698729810761250, 11.00000000000000000 ) ) ;
#38556=CARTESIAN_POINT ( 'NONE',  ( -0.4999999999999998890, 37.18846563620834189, 10.96580507645519909 ) ) ;
#38558=CARTESIAN_POINT ( 'NONE',  ( 13.94482798346721175, 26.50521816028912525, 11.00000000000000000 ) ) ;
#38569=CARTESIAN_POINT ( 'NONE',  ( 12.80736835487433112, 15.68301270189216545, 9.500000000000000000 ) ) ;
#38570=EDGE_CURVE ( 'NONE', #29211, #1824, #35935, .T. ) ;
#38573=ORIENTED_EDGE ( 'NONE', *, *, #36979, .F. ) ;
#38575=CARTESIAN_POINT ( 'NONE',  ( 14.57109471128388378, 21.97402451295022630, 10.49999999999999822 ) ) ;
#38577=DIRECTION ( 'NONE',  ( -0.2079116908177533751, 0.9781476007338067991, 0.000000000000000000 ) ) ;
#38578=CARTESIAN_POINT ( 'NONE',  ( 10.70158575030369796, 30.79011836036717753, 10.50000000000000000 ) ) ;
#38581=ORIENTED_EDGE ( 'NONE', *, *, #30613, .T. ) ;
#38584=VERTEX_POINT ( 'NONE', #35328 ) ;
#38587=AXIS2_PLACEMENT_3D ( 'NONE', #28555, #37703, #728 ) ;
#38592=DIRECTION ( 'NONE',  ( 0.1470157664651866314, 0.6916548014802309519, -0.7071067811865446862 ) ) ;
#38593=ORIENTED_EDGE ( 'NONE', *, *, #8773, .T. ) ;
#38595=CARTESIAN_POINT ( 'NONE',  ( -2.618397918552020975, 7.776539141412908585, 10.76099332938163755 ) ) ;
#38599=ORIENTED_EDGE ( 'NONE', *, *, #20583, .T. ) ;
#38601=DIRECTION ( 'NONE',  ( 1.000000000000000000, 0.000000000000000000, 0.000000000000000000 ) ) ;
#38605=AXIS2_PLACEMENT_3D ( 'NONE', #32479, #26573, #4432 ) ;
#38606=ORIENTED_EDGE ( 'NONE', *, *, #30545, .T. ) ;
#38610=ADVANCED_FACE ( 'NONE', ( #26379 ), #20500, .F. ) ;
#38612=EDGE_CURVE ( 'NONE', #6323, #1436, #38630, .T. ) ;
#38614=ORIENTED_EDGE ( 'NONE', *, *, #21652, .T. ) ;
#38619=AXIS2_PLACEMENT_3D ( 'NONE', #33319, #17878, #30261 ) ;
#38622=DIRECTION ( 'NONE',  ( 1.000000000000000000, 0.000000000000000000, 0.000000000000000000 ) ) ;
#38623=VERTEX_POINT ( 'NONE', #17663 ) ;
#38625=CARTESIAN_POINT ( 'NONE',  ( -10.10646936306323340, 32.94553861768096681, 10.49999999999999822 ) ) ;
#38626=CARTESIAN_POINT ( 'NONE',  ( -8.927394655428429360, 11.06314620770957013, 11.00000000000000000 ) ) ;
#38627=LINE ( 'NONE', #13032, #35520 ) ;
#38628=ORIENTED_EDGE ( 'NONE', *, *, #11364, .F. ) ;
#38630=B_SPLINE_CURVE_WITH_KNOTS ( 'NONE', 3,
 ( #10544, #39175, #11354, #36137, #20704, #4847, #35533, #5251 ),
 .UNSPECIFIED., .F., .F.,
 ( 4, 2, 2, 4 ),
 ( 8.673617379884035472E-19, 0.0004726692273637259339, 0.0007090038410455884671, 0.0009453384547274510004 ),
 .UNSPECIFIED. ) ;
#38634=CARTESIAN_POINT ( 'NONE',  ( -5.947717410344457001, 34.62949535663729250, 10.00000000000000000 ) ) ;
#38639=CARTESIAN_POINT ( 'NONE',  ( 2.036571916123615100, 8.108948098542045457, 7.499999999999990230 ) ) ;
#38640=EDGE_CURVE ( 'NONE', #22764, #2610, #28691, .T. ) ;
#38642=DIRECTION ( 'NONE',  ( -0.8090169943749426773, 0.5877852522924797984, 0.000000000000000000 ) ) ;
#38644=ADVANCED_FACE ( 'NONE', ( #13584 ), #25971, .T. ) ;
#38645=DIRECTION ( 'NONE',  ( -0.000000000000000000, -0.000000000000000000, -1.000000000000000000 ) ) ;
#38648=AXIS2_PLACEMENT_3D ( 'NONE', #7115, #13620, #1435 ) ;
#38649=CARTESIAN_POINT ( 'NONE',  ( 9.593820794837855104, 26.14295245049076755, 10.75000000000000000 ) ) ;
#38657=ORIENTED_EDGE ( 'NONE', *, *, #34640, .T. ) ;
#38662=ORIENTED_EDGE ( 'NONE', *, *, #22388, .F. ) ;
#38664=EDGE_LOOP ( 'NONE', ( #19159, #10913, #24258, #27870 ) ) ;
#38666=CARTESIAN_POINT ( 'NONE',  ( -2.525645716490712012, 8.212903943950955465, 7.000000000000000000 ) ) ;
#38667=EDGE_CURVE ( 'NONE', #34838, #26378, #22835, .T. ) ;
#38669=LINE ( 'NONE', #10841, #13388 ) ;
#38670=EDGE_CURVE ( 'NONE', #31336, #20131, #5453, .T. ) ;
#38678=CARTESIAN_POINT ( 'NONE',  ( -10.81260707898136708, 32.90853150812170469, 10.49999999999999822 ) ) ;
#38679=DIRECTION ( 'NONE',  ( 0.1045284632676564129, 0.9945218953682731788, 0.000000000000000000 ) ) ;
#38680=CIRCLE ( 'NONE', #30245, 1.000000000000000222 ) ;
#38684=CIRCLE ( 'NONE', #4194, 0.5000000000000004441 ) ;
#38685=VECTOR ( 'NONE', #15727, 1000.000000000000227 ) ;
#38688=ORIENTED_EDGE ( 'NONE', *, *, #4837, .F. ) ;
#38694=EDGE_CURVE ( 'NONE', #26220, #14950, #8048, .T. ) ;
#38695=ADVANCED_FACE ( 'NONE', ( #11313 ), #16601, .T. ) ;
#38696=CARTESIAN_POINT ( 'NONE',  ( 3.399837471815453593, 8.909889435135580626, 9.500000000000000000 ) ) ;
#38697=DIRECTION ( 'NONE',  ( -0.9945218953682748442, -0.1045284632676391490, 0.000000000000000000 ) ) ;
#38698=PLANE ( 'NONE',  #15948 ) ;
#38699=VERTEX_POINT ( 'NONE', #10498 ) ;
#38700=DIRECTION ( 'NONE',  ( 0.5000000000000041078, 0.8660254037844362651, 0.000000000000000000 ) ) ;
#38703=CARTESIAN_POINT ( 'NONE',  ( 7.468455364333220103, 29.89744377950669474, 10.00000000000000000 ) ) ;
#38704=CARTESIAN_POINT ( 'NONE',  ( 8.796116341590819232, 23.42450908139080568, 7.000000000000000000 ) ) ;
#38707=ORIENTED_EDGE ( 'NONE', *, *, #14263, .F. ) ;
#38709=VECTOR ( 'NONE', #39064, 1000.000000000000000 ) ;
#38712=DIRECTION ( 'NONE',  ( -0.07391278520355985815, 0.7032331762534049791, -0.7071067811865475727 ) ) ;
#38716=ORIENTED_EDGE ( 'NONE', *, *, #22669, .F. ) ;
#38718=CARTESIAN_POINT ( 'NONE',  ( 13.98881638187875787, 26.51951085733867330, 10.99999999999999289 ) ) ;
#38719=ADVANCED_FACE ( 'NONE', ( #13741 ), #19848, .F. ) ;
#38726=ORIENTED_EDGE ( 'NONE', *, *, #16307, .F. ) ;
#38729=LINE ( 'NONE', #13939, #37432 ) ;
#38730=LINE ( 'NONE', #27141, #19308 ) ;
#38731=ORIENTED_EDGE ( 'NONE', *, *, #37153, .F. ) ;
#38736=DIRECTION ( 'NONE',  ( -0.000000000000000000, -0.000000000000000000, -1.000000000000000000 ) ) ;
#38737=CARTESIAN_POINT ( 'NONE',  ( -11.54666566735214772, 32.07468077621344094, 7.000000000000000000 ) ) ;
#38741=ADVANCED_FACE ( 'NONE', ( #24489 ), #27147, .F. ) ;
#38743=DIRECTION ( 'NONE',  ( 1.000000000000000000, 0.000000000000000000, 0.000000000000000000 ) ) ;
#38746=ORIENTED_EDGE ( 'NONE', *, *, #7907, .F. ) ;
#38748=LINE ( 'NONE', #26354, #36652 ) ;
#38751=DIRECTION ( 'NONE',  ( -0.9945218953682742891, -0.1045284632676437425, 0.000000000000000000 ) ) ;
#38752=FACE_OUTER_BOUND ( 'NONE', #5459, .T. ) ;
#38755=ORIENTED_EDGE ( 'NONE', *, *, #19410, .F. ) ;
#38764=VECTOR ( 'NONE', #16342, 1000.000000000000000 ) ;
#38771=EDGE_CURVE ( 'NONE', #18941, #20144, #24144, .T. ) ;
#38772=ORIENTED_EDGE ( 'NONE', *, *, #16957, .F. ) ;
#38775=EDGE_LOOP ( 'NONE', ( #39389, #2663, #2362, #20066 ) ) ;
#38778=ORIENTED_EDGE ( 'NONE', *, *, #14101, .T. ) ;
#38779=CARTESIAN_POINT ( 'NONE',  ( -10.81260707898136353, 32.90853150812170469, 10.50000000000000000 ) ) ;
#38780=CARTESIAN_POINT ( 'NONE',  ( 9.038171950369859431, 10.91067434175320017, 10.96580508970280654 ) ) ;
#38782=ORIENTED_EDGE ( 'NONE', *, *, #25268, .T. ) ;
#38786=ORIENTED_EDGE ( 'NONE', *, *, #38303, .F. ) ;
#38788=ORIENTED_EDGE ( 'NONE', *, *, #3667, .T. ) ;
#38789=CIRCLE ( 'NONE', #18125, 0.5000000000000004441 ) ;
#38791=CARTESIAN_POINT ( 'NONE',  ( -4.591666147298613332, 15.32946292166675306, 7.000000000000000000 ) ) ;
#38793=AXIS2_PLACEMENT_3D ( 'NONE', #25977, #34934, #7491 ) ;
#38794=CIRCLE ( 'NONE', #515, 15.00000000000000000 ) ;
#38795=DIRECTION ( 'NONE',  ( -0.6123724356957894743, 0.3535533905932873311, -0.7071067811865451302 ) ) ;
#38798=CARTESIAN_POINT ( 'NONE',  ( -6.811226782241547539, 35.33967249274200384, 7.000000000000000000 ) ) ;
#38802=VECTOR ( 'NONE', #37179, 1000.000000000000227 ) ;
#38804=ORIENTED_EDGE ( 'NONE', *, *, #1611, .T. ) ;
#38805=CARTESIAN_POINT ( 'NONE',  ( -13.63581098909220302, 27.45627467658446719, 11.00000000000000000 ) ) ;
#38806=CARTESIAN_POINT ( 'NONE',  ( 5.440908595777817602, 35.94977745735560859, 11.00000000000000000 ) ) ;
#38809=CARTESIAN_POINT ( 'NONE',  ( -14.86556419889029534, 20.43481210330121556, 10.49999999999999822 ) ) ;
#38810=ORIENTED_EDGE ( 'NONE', *, *, #22230, .F. ) ;
#38814=EDGE_CURVE ( 'NONE', #21971, #23024, #30797, .T. ) ;
#38815=CYLINDRICAL_SURFACE ( 'NONE', #20530, 0.5000000000000015543 ) ;
#38819=CARTESIAN_POINT ( 'NONE',  ( -2.518583951651200081, 7.712953814960714638, 7.000000000000000000 ) ) ;
#38820=CARTESIAN_POINT ( 'NONE',  ( 2.025645716490518389, 8.212903943950921715, 7.499999999999990230 ) ) ;
#38824=VERTEX_POINT ( 'NONE', #2961 ) ;
#38826=EDGE_CURVE ( 'NONE', #22802, #38413, #17023, .T. ) ;
#38829=LINE ( 'NONE', #8146, #14147 ) ;
#38830=ADVANCED_FACE ( 'NONE', ( #36889 ), #39724, .T. ) ;
#38832=ORIENTED_EDGE ( 'NONE', *, *, #21456, .T. ) ;
#38834=CARTESIAN_POINT ( 'NONE',  ( 2.421689871081641687, 8.701977744317826335, 10.00000000000000000 ) ) ;
#38835=VERTEX_POINT ( 'NONE', #11906 ) ;
#38844=LINE ( 'NONE', #7348, #14206 ) ;
#38845=ORIENTED_EDGE ( 'NONE', *, *, #34431, .T. ) ;
#38846=ADVANCED_FACE ( 'NONE', ( #33060 ), #21053, .T. ) ;
#38848=EDGE_CURVE ( 'NONE', #32089, #24654, #4010, .T. ) ;
#38849=VECTOR ( 'NONE', #22584, 1000.000000000000000 ) ;
#38852=LINE ( 'NONE', #38649, #8686 ) ;
#38855=CARTESIAN_POINT ( 'NONE',  ( -3.057264508911469392, 12.92643568347973826, 10.50000000000000533 ) ) ;
#38864=CARTESIAN_POINT ( 'NONE',  ( -2.362621116368410323, 8.178251995481311099, 10.83333333333333215 ) ) ;
#38872=EDGE_CURVE ( 'NONE', #27126, #4300, #5998, .T. ) ;
#38873=CARTESIAN_POINT ( 'NONE',  ( 13.28503138821876917, 15.53523575316134142, 7.499999999999997335 ) ) ;
#38874=ORIENTED_EDGE ( 'NONE', *, *, #23760, .F. ) ;
#38877=DIRECTION ( 'NONE',  ( -0.000000000000000000, -0.000000000000000000, -1.000000000000000000 ) ) ;
#38881=CARTESIAN_POINT ( 'NONE',  ( -7.852310722359095330, 10.04909572729077105, 10.49999999999999822 ) ) ;
#38883=ORIENTED_EDGE ( 'NONE', *, *, #26033, .F. ) ;
#38885=AXIS2_PLACEMENT_3D ( 'NONE', #14789, #11541, #5840 ) ;
#38887=VECTOR ( 'NONE', #38960, 1000.000000000000227 ) ;
#38889=ORIENTED_EDGE ( 'NONE', *, *, #39336, .T. ) ;
#38891=AXIS2_PLACEMENT_3D ( 'NONE', #18905, #27848, #3465 ) ;
#38893=LINE ( 'NONE', #14506, #24536 ) ;
#38894=DIRECTION ( 'NONE',  ( 0.3090169943749573322, 0.9510565162951505336, -0.000000000000000000 ) ) ;
#38895=EDGE_CURVE ( 'NONE', #20144, #20763, #5604, .T. ) ;
#38896=CARTESIAN_POINT ( 'NONE',  ( -2.440759101148431309, 7.699698400927159625, 7.485646746502371940 ) ) ;
#38898=FACE_OUTER_BOUND ( 'NONE', #12196, .T. ) ;
#38901=LINE ( 'NONE', #35853, #32623 ) ;
#38905=DIRECTION ( 'NONE',  ( 0.5000000000000038858, 0.8660254037844364872, -0.000000000000000000 ) ) ;
#38907=DIRECTION ( 'NONE',  ( -0.7431448254773846962, 0.6691306063588690067, -6.938893903907220489E-15 ) ) ;
#38908=ORIENTED_EDGE ( 'NONE', *, *, #27283, .F. ) ;
#38912=DIRECTION ( 'NONE',  ( 0.000000000000000000, 0.000000000000000000, -1.000000000000000000 ) ) ;
#38914=VERTEX_POINT ( 'NONE', #14755 ) ;
#38918=CARTESIAN_POINT ( 'NONE',  ( -3.713592597587354049, 7.966960743906858156, 7.000000000000000000 ) ) ;
#38926=EDGE_CURVE ( 'NONE', #18941, #26640, #20905, .T. ) ;
#38930=CARTESIAN_POINT ( 'NONE',  ( 3.914034194965611668, 30.06176806842419680, 9.000000000000001776 ) ) ;
#38931=ORIENTED_EDGE ( 'NONE', *, *, #14771, .T. ) ;
#38933=EDGE_CURVE ( 'NONE', #16076, #39330, #13758, .T. ) ;
#38936=DIRECTION ( 'NONE',  ( 0.9781476007338043566, -0.2079116908177657264, 0.000000000000000000 ) ) ;
#38937=DIRECTION ( 'NONE',  ( 0.2113248654051944064, 0.7886751345948047609, 0.5773502691896342798 ) ) ;
#38940=CONICAL_SURFACE ( 'NONE', #35700, 0.5000000000000065503, 0.7853981633974495002 ) ;
#38941=ORIENTED_EDGE ( 'NONE', *, *, #32459, .F. ) ;
#38942=EDGE_CURVE ( 'NONE', #10398, #2507, #37775, .T. ) ;
#38943=VECTOR ( 'NONE', #11272, 1000.000000000000114 ) ;
#38947=CARTESIAN_POINT ( 'NONE',  ( 6.643188263510064751, 35.96180620077102219, 10.49999999999999822 ) ) ;
#38948=CARTESIAN_POINT ( 'NONE',  ( 0.5000000000000002220, 36.00000000000000711, 10.00000000000000000 ) ) ;
#38952=DIRECTION ( 'NONE',  ( 0.000000000000000000, 0.000000000000000000, -1.000000000000000000 ) ) ;
#38953=CARTESIAN_POINT ( 'NONE',  ( 12.74038105676654453, 14.56698729810772264, 10.49999999999999822 ) ) ;
#38954=CARTESIAN_POINT ( 'NONE',  ( 9.427394655437332460, 10.98460639141775808, 10.49999999999999645 ) ) ;
#38956=DIRECTION ( 'NONE',  ( -1.000000000000000000, 0.000000000000000000, 0.000000000000000000 ) ) ;
#38957=ORIENTED_EDGE ( 'NONE', *, *, #39842, .T. ) ;
#38958=VECTOR ( 'NONE', #13955, 1000.000000000000114 ) ;
#38960=DIRECTION ( 'NONE',  ( 0.9945218953682742891, 0.1045284632676437425, -0.000000000000000000 ) ) ;
#38963=CARTESIAN_POINT ( 'NONE',  ( 8.410254037844358876, 17.06698729810774395, 10.49999999999999822 ) ) ;
#38967=ADVANCED_FACE ( 'NONE', ( #35388 ), #19338, .T. ) ;
#38971=ADVANCED_FACE ( 'NONE', ( #24888 ), #35180, .F. ) ;
#38973=DIRECTION ( 'NONE',  ( 0.000000000000000000, 0.000000000000000000, -1.000000000000000000 ) ) ;
#38974=ORIENTED_EDGE ( 'NONE', *, *, #20212, .F. ) ;
#38975=AXIS2_PLACEMENT_3D ( 'NONE', #34552, #429, #19111 ) ;
#38982=ORIENTED_EDGE ( 'NONE', *, *, #27736, .T. ) ;
#38984=ORIENTED_EDGE ( 'NONE', *, *, #8528, .T. ) ;
#38986=VECTOR ( 'NONE', #23207, 1000.000000000000227 ) ;
#38987=ORIENTED_EDGE ( 'NONE', *, *, #22044, .F. ) ;
#38988=DIRECTION ( 'NONE',  ( -0.1470157664652021190, 0.6916548014802263999, -0.7071067811865459074 ) ) ;
#38989=ORIENTED_EDGE ( 'NONE', *, *, #19138, .F. ) ;
#38990=FACE_OUTER_BOUND ( 'NONE', #1617, .T. ) ;
#38991=CARTESIAN_POINT ( 'NONE',  ( 7.611215932167711529, 18.68301270189218855, 9.000000000000001776 ) ) ;
#38993=DIRECTION ( 'NONE',  ( 0.000000000000000000, -0.6445931928399307731, 0.7645257456387090089 ) ) ;
#38994=VERTEX_POINT ( 'NONE', #19946 ) ;
#38998=AXIS2_PLACEMENT_3D ( 'NONE', #10316, #22898, #23317 ) ;
#39002=ORIENTED_EDGE ( 'NONE', *, *, #33265, .F. ) ;
#39003=CARTESIAN_POINT ( 'NONE',  ( 5.198706521309295780, 29.65540566576566661, 7.000000000000000000 ) ) ;
#39004=CARTESIAN_POINT ( 'NONE',  ( 13.63581098909226874, 27.45627467658428955, 9.000000000000001776 ) ) ;
#39007=CARTESIAN_POINT ( 'NONE',  ( -14.47283171447380212, 21.48159823030330529, 11.00000000000000000 ) ) ;
#39011=VECTOR ( 'NONE', #2866, 1000.000000000000000 ) ;
#39012=DIRECTION ( 'NONE',  ( -0.3090169943749573878, -0.9510565162951503115, 0.000000000000000000 ) ) ;
#39013=VERTEX_POINT ( 'NONE', #16499 ) ;
#39014=ORIENTED_EDGE ( 'NONE', *, *, #31511, .T. ) ;
#39016=DIRECTION ( 'NONE',  ( -1.000000000000000000, 0.000000000000000000, 0.000000000000000000 ) ) ;
#39022=DIRECTION ( 'NONE',  ( -0.000000000000000000, -0.000000000000000000, -1.000000000000000000 ) ) ;
#39024=AXIS2_PLACEMENT_3D ( 'NONE', #21927, #1003, #22129 ) ;
#39029=ORIENTED_EDGE ( 'NONE', *, *, #20205, .T. ) ;
#39032=ORIENTED_EDGE ( 'NONE', *, *, #8420, .F. ) ;
#39037=AXIS2_PLACEMENT_3D ( 'NONE', #35098, #10514, #25746 ) ;
#39038=PLANE ( 'NONE',  #17475 ) ;
#39040=EDGE_CURVE ( 'NONE', #11564, #4629, #34988, .T. ) ;
#39041=LINE ( 'NONE', #6990, #24960 ) ;
#39045=EDGE_CURVE ( 'NONE', #26235, #5593, #1058, .T. ) ;
#39047=AXIS2_PLACEMENT_3D ( 'NONE', #13787, #26586, #17459 ) ;
#39051=CARTESIAN_POINT ( 'NONE',  ( 1.693998953219503445, 12.12549434688615690, 10.50000000000000000 ) ) ;
#39053=ORIENTED_EDGE ( 'NONE', *, *, #35361, .T. ) ;
#39058=DIRECTION ( 'NONE',  ( 1.000000000000000000, 0.000000000000000000, 0.000000000000000000 ) ) ;
#39060=ORIENTED_EDGE ( 'NONE', *, *, #4304, .F. ) ;
#39062=ORIENTED_EDGE ( 'NONE', *, *, #12404, .F. ) ;
#39064=DIRECTION ( 'NONE',  ( -0.000000000000000000, -0.000000000000000000, -1.000000000000000000 ) ) ;
#39066=CARTESIAN_POINT ( 'NONE',  ( 13.00577423375721864, 27.77729443754439487, 9.500000000000000000 ) ) ;
#39072=EDGE_LOOP ( 'NONE', ( #17383, #38086, #38056, #40013 ) ) ;
#39074=DIRECTION ( 'NONE',  ( 0.000000000000000000, 0.000000000000000000, 1.000000000000000000 ) ) ;
#39075=EDGE_CURVE ( 'NONE', #36019, #1586, #25435, .T. ) ;
#39077=ADVANCED_FACE ( 'NONE', ( #22779 ), #19755, .T. ) ;
#39078=VERTEX_POINT ( 'NONE', #36191 ) ;
#39082=ORIENTED_EDGE ( 'NONE', *, *, #4564, .T. ) ;
#39083=VECTOR ( 'NONE', #6491, 1000.000000000000227 ) ;
#39087=VECTOR ( 'NONE', #10235, 1000.000000000000114 ) ;
#39088=DIRECTION ( 'NONE',  ( -0.000000000000000000, -0.000000000000000000, -1.000000000000000000 ) ) ;
#39089=EDGE_CURVE ( 'NONE', #23174, #24240, #37114, .T. ) ;
#39090=CARTESIAN_POINT ( 'NONE',  ( 13.87104230352200140, 20.53934056656866147, 7.500000000000010658 ) ) ;
#39092=DIRECTION ( 'NONE',  ( -0.000000000000000000, -0.000000000000000000, 1.000000000000000000 ) ) ;
#39093=ORIENTED_EDGE ( 'NONE', *, *, #2328, .F. ) ;
#39098=CARTESIAN_POINT ( 'NONE',  ( 9.819582157326486538, 24.63911342745429778, 10.50000000000000533 ) ) ;
#39100=VECTOR ( 'NONE', #5772, 1000.000000000000000 ) ;
#39101=CARTESIAN_POINT ( 'NONE',  ( -9.697889840765288483, 31.90483559858339646, 9.500000000000000000 ) ) ;
#39102=ORIENTED_EDGE ( 'NONE', *, *, #34983, .T. ) ;
#39108=VERTEX_POINT ( 'NONE', #39425 ) ;
#39109=CARTESIAN_POINT ( 'NONE',  ( -14.97009266215794376, 21.42933399866948463, 10.50000000000000178 ) ) ;
#39110=ORIENTED_EDGE ( 'NONE', *, *, #25174, .T. ) ;
#39115=CIRCLE ( 'NONE', #3411, 0.5000000000000004441 ) ;
#39119=ORIENTED_EDGE ( 'NONE', *, *, #19083, .T. ) ;
#39121=DIRECTION ( 'NONE',  ( -1.000000000000000000, 0.000000000000000000, 0.000000000000000000 ) ) ;
#39123=ADVANCED_FACE ( 'NONE', ( #8553 ), #20555, .T. ) ;
#39124=PLANE ( 'NONE',  #36836 ) ;
#39125=ORIENTED_EDGE ( 'NONE', *, *, #29980, .T. ) ;
#39127=VECTOR ( 'NONE', #31203, 1000.000000000000000 ) ;
#39131=CARTESIAN_POINT ( 'NONE',  ( -13.28503138821885798, 15.53523575316151195, 7.499999999999993783 ) ) ;
#39132=( NAMED_UNIT ( * ) SI_UNIT ( $, .STERADIAN. ) SOLID_ANGLE_UNIT ( ) );
#39135=ORIENTED_EDGE ( 'NONE', *, *, #38670, .F. ) ;
#39136=CARTESIAN_POINT ( 'NONE',  ( -12.68475447279705470, 27.14725768220950641, 10.00000000000000000 ) ) ;
#39137=ADVANCED_FACE ( 'NONE', ( #17110 ), #26639, .T. ) ;
#39138=AXIS2_PLACEMENT_3D ( 'NONE', #13301, #9865, #25698 ) ;
#39139=CARTESIAN_POINT ( 'NONE',  ( 6.513333500389088648, 35.89988989478896997, 10.82238861112342043 ) ) ;
#39140=CARTESIAN_POINT ( 'NONE',  ( -8.927394655428429360, 11.06314620770957013, 9.000000000000001776 ) ) ;
#39141=ADVANCED_FACE ( 'NONE', ( #29886 ), #20151, .T. ) ;
#39143=CARTESIAN_POINT ( 'NONE',  ( -5.198706521309195416, 29.65540566576573767, 9.000000000000001776 ) ) ;
#39144=CARTESIAN_POINT ( 'NONE',  ( -12.92073081513906452, 15.61756285494255003, 11.00000000000000000 ) ) ;
#39145=DIRECTION ( 'NONE',  ( -0.000000000000000000, -0.000000000000000000, -1.000000000000000000 ) ) ;
#39147=AXIS2_PLACEMENT_3D ( 'NONE', #4776, #33030, #39502 ) ;
#39150=CYLINDRICAL_SURFACE ( 'NONE', #9479, 6.000000000000015987 ) ;
#39151=ORIENTED_EDGE ( 'NONE', *, *, #2120, .F. ) ;
#39152=EDGE_CURVE ( 'NONE', #26378, #20669, #26234, .T. ) ;
#39156=CARTESIAN_POINT ( 'NONE',  ( -0.4999999999999998890, 37.50000000000000711, 10.49999999999999467 ) ) ;
#39158=DIRECTION ( 'NONE',  ( 1.000000000000000000, 0.000000000000000000, 0.000000000000000000 ) ) ;
#39161=DIRECTION ( 'NONE',  ( -1.000000000000000000, 0.000000000000000000, 0.000000000000000000 ) ) ;
#39162=VECTOR ( 'NONE', #32872, 1000.000000000000000 ) ;
#39167=CARTESIAN_POINT ( 'NONE',  ( -14.31603901957233660, 19.98981538725089990, 7.500000000000004441 ) ) ;
#39168=EDGE_CURVE ( 'NONE', #13732, #31717, #9492, .T. ) ;
#39169=ORIENTED_EDGE ( 'NONE', *, *, #40178, .T. ) ;
#39172=EDGE_LOOP ( 'NONE', ( #17236, #39510, #597, #10902, #26595, #33312, #39179, #19560, #23804, #11160, #23733, #32170, #31425, #29772, #13063, #25453, #24216, #7547, #30346, #33204, #36598, #10853, #36382, #15499, #21332, #9195, #18972, #13297, #7061, #23620, #16088, #6178, #910, #29841, #19388, #36638, #12765, #36333, #6527, #18943, #4552, #4557, #34981, #29715, #30127, #249 ) ) ;
#39173=EDGE_CURVE ( 'NONE', #13029, #9605, #9907, .T. ) ;
#39175=CARTESIAN_POINT ( 'NONE',  ( 4.908384188814759241, 36.67470053474868052, 7.102637441331453694 ) ) ;
#39176=ORIENTED_EDGE ( 'NONE', *, *, #3169, .F. ) ;
#39177=DIRECTION ( 'NONE',  ( -0.5138379476002908897, 0.6345370204114160195, 0.5773502691896168493 ) ) ;
#39179=ORIENTED_EDGE ( 'NONE', *, *, #34849, .F. ) ;
#39181=EDGE_LOOP ( 'NONE', ( #33221, #6710, #31531 ) ) ;
#39184=ORIENTED_EDGE ( 'NONE', *, *, #14351, .F. ) ;
#39186=CARTESIAN_POINT ( 'NONE',  ( -6.354454053420242943, 35.54304081427989814, 11.00000000000000000 ) ) ;
#39187=ORIENTED_EDGE ( 'NONE', *, *, #11126, .T. ) ;
#39188=DIRECTION ( 'NONE',  ( -0.5877852522924796874, -0.8090169943749426773, 0.000000000000000000 ) ) ;
#39189=FACE_OUTER_BOUND ( 'NONE', #46, .T. ) ;
#39193=LINE ( 'NONE', #14617, #9692 ) ;
#39194=ORIENTED_EDGE ( 'NONE', *, *, #31983, .F. ) ;
#39195=ADVANCED_FACE ( 'NONE', ( #33354 ), #37798, .T. ) ;
#39197=DIRECTION ( 'NONE',  ( 0.7071067811865451302, 8.659560562354889717E-17, -0.7071067811865500152 ) ) ;
#39198=CARTESIAN_POINT ( 'NONE',  ( -8.410254037844433483, 17.06698729810786475, 10.00000000000000000 ) ) ;
#39201=CIRCLE ( 'NONE', #283, 0.5000000000000004441 ) ;
#39202=EDGE_LOOP ( 'NONE', ( #13893, #34733, #15650, #38468 ) ) ;
#39203=ADVANCED_FACE ( 'NONE', ( #14044 ), #17911, .T. ) ;
#39204=DIRECTION ( 'NONE',  ( -0.000000000000000000, -0.000000000000000000, -1.000000000000000000 ) ) ;
#39205=DIRECTION ( 'NONE',  ( 0.9781476007338041345, -0.2079116908177664202, -0.000000000000000000 ) ) ;
#39207=DIRECTION ( 'NONE',  ( 1.000000000000000000, 0.000000000000000000, 0.000000000000000000 ) ) ;
#39210=VECTOR ( 'NONE', #8771, 1000.000000000000114 ) ;
#39213=DIRECTION ( 'NONE',  ( 0.8090169943749426773, -0.5877852522924796874, -0.000000000000000000 ) ) ;
#39214=ORIENTED_EDGE ( 'NONE', *, *, #5213, .F. ) ;
#39215=ORIENTED_EDGE ( 'NONE', *, *, #7448, .F. ) ;
#39217=CARTESIAN_POINT ( 'NONE',  ( -4.003793317224517700, 8.420815634768723967, 11.00000000000000000 ) ) ;
#39219=ADVANCED_FACE ( 'NONE', ( #32550 ), #15738, .T. ) ;
#39220=AXIS2_PLACEMENT_3D ( 'NONE', #19312, #19923, #28858 ) ;
#39221=DIRECTION ( 'NONE',  ( 0.000000000000000000, 0.000000000000000000, 1.000000000000000000 ) ) ;
#39222=ORIENTED_EDGE ( 'NONE', *, *, #31739, .F. ) ;
#39225=DIRECTION ( 'NONE',  ( 0.7622652262560051240, -0.2926062055178242916, 0.5773502691896332806 ) ) ;
#39229=CARTESIAN_POINT ( 'NONE',  ( 0.000000000000000000, 22.50000000000000355, 7.000000000000000000 ) ) ;
#39230=ORIENTED_EDGE ( 'NONE', *, *, #37582, .F. ) ;
#39237=DIRECTION ( 'NONE',  ( -0.7431448254773882489, 0.6691306063588648989, 0.000000000000000000 ) ) ;
#39239=DIRECTION ( 'NONE',  ( -0.7032331762534054231, 0.07391278520356943382, -0.7071067811865461294 ) ) ;
#39240=VERTEX_POINT ( 'NONE', #1663 ) ;
#39241=EDGE_CURVE ( 'NONE', #37722, #751, #26436, .T. ) ;
#39244=AXIS2_PLACEMENT_3D ( 'NONE', #28813, #16632, #9732 ) ;
#39246=DIRECTION ( 'NONE',  ( -1.224646799147351235E-16, 1.000000000000000000, 0.000000000000000000 ) ) ;
#39249=FACE_OUTER_BOUND ( 'NONE', #7103, .T. ) ;
#39250=CARTESIAN_POINT ( 'NONE',  ( -13.01373512358517459, 15.56386679242537774, 10.94387467462635577 ) ) ;
#39251=CARTESIAN_POINT ( 'NONE',  ( 2.596139932171742437, 7.881254734312914678, 10.87262190629281200 ) ) ;
#39252=ORIENTED_EDGE ( 'NONE', *, *, #34109, .F. ) ;
#39255=TOROIDAL_SURFACE ( 'NONE', #6162, 1.000000000000000000, 0.5000000000000000000 ) ;
#39257=AXIS2_PLACEMENT_3D ( 'NONE', #28714, #9834, #25270 ) ;
#39259=CARTESIAN_POINT ( 'NONE',  ( -14.45052027064702749, 26.47704597190823606, 10.49999999999999822 ) ) ;
#39261=EDGE_LOOP ( 'NONE', ( #26260, #1113, #34909 ) ) ;
#39263=ORIENTED_EDGE ( 'NONE', *, *, #7990, .T. ) ;
#39265=DIRECTION ( 'NONE',  ( 1.000000000000000000, 0.000000000000000000, 0.000000000000000000 ) ) ;
#39267=DIRECTION ( 'NONE',  ( 0.000000000000000000, 0.000000000000000000, -1.000000000000000000 ) ) ;
#39268=VERTEX_POINT ( 'NONE', #34143 ) ;
#39271=DIRECTION ( 'NONE',  ( 1.000000000000000000, -3.469446951953574746E-15, 0.000000000000000000 ) ) ;
#39274=EDGE_CURVE ( 'NONE', #19973, #2054, #22221, .T. ) ;
#39275=CARTESIAN_POINT ( 'NONE',  ( -4.527363138135027221, 36.35651410043147536, 7.000000000000000000 ) ) ;
#39276=DIRECTION ( 'NONE',  ( 0.6459741880212496179, -0.2876062384759507373, 0.7071067811865487940 ) ) ;
#39277=B_SPLINE_CURVE_WITH_KNOTS ( 'NONE', 3,
 ( #24766, #37162, #18877, #12772, #10132, #3236 ),
 .UNSPECIFIED., .F., .F.,
 ( 4, 2, 4 ),
 ( 0.000000000000000000, 0.5000000000000000000, 1.000000000000000000 ),
 .UNSPECIFIED. ) ;
#39282=ORIENTED_EDGE ( 'NONE', *, *, #25148, .T. ) ;
#39286=FACE_OUTER_BOUND ( 'NONE', #12499, .T. ) ;
#39287=DIRECTION ( 'NONE',  ( -0.9945218953682740670, -0.1045284632676460046, 0.000000000000000000 ) ) ;
#39289=CIRCLE ( 'NONE', #28898, 0.4999999999999995559 ) ;
#39290=DIRECTION ( 'NONE',  ( 0.000000000000000000, 0.000000000000000000, -1.000000000000000000 ) ) ;
#39291=CARTESIAN_POINT ( 'NONE',  ( 6.354454053420411697, 35.54304081427980577, 7.000000000000000000 ) ) ;
#39293=CARTESIAN_POINT ( 'NONE',  ( -3.503793317224517700, 8.420815634768727520, 9.500000000000000000 ) ) ;
#39294=ORIENTED_EDGE ( 'NONE', *, *, #39297, .T. ) ;
#39296=LINE ( 'NONE', #11474, #33299 ) ;
#39297=EDGE_CURVE ( 'NONE', #18974, #163, #31093, .T. ) ;
#39301=FACE_OUTER_BOUND ( 'NONE', #35429, .T. ) ;
#39304=VERTEX_POINT ( 'NONE', #37384 ) ;
#39307=CARTESIAN_POINT ( 'NONE',  ( 11.80736835487432401, 14.81698729810772619, 7.499999999999997335 ) ) ;
#39311=ORIENTED_EDGE ( 'NONE', *, *, #36498, .F. ) ;
#39312=AXIS2_PLACEMENT_3D ( 'NONE', #21223, #12471, #21812 ) ;
#39314=DIRECTION ( 'NONE',  ( 1.000000000000000000, -6.938893903907174735E-15, 0.000000000000000000 ) ) ;
#39317=AXIS2_PLACEMENT_3D ( 'NONE', #7258, #33771, #29006 ) ;
#39321=CARTESIAN_POINT ( 'NONE',  ( 5.238409041734346516, 36.41108174777518514, 10.49999999999999822 ) ) ;
#39323=VERTEX_POINT ( 'NONE', #39824 ) ;
#39325=CIRCLE ( 'NONE', #31543, 0.5000000000000004441 ) ;
#39327=DIRECTION ( 'NONE',  ( 0.2876062384759419666, -0.6459741880212652720, -0.7071067811865382469 ) ) ;
#39328=CARTESIAN_POINT ( 'NONE',  ( 8.238488885696289898, 24.65111619403943877, 9.000000000000001776 ) ) ;
#39330=VERTEX_POINT ( 'NONE', #33939 ) ;
#39335=CARTESIAN_POINT ( 'NONE',  ( -14.47283171447380212, 21.48159823030330884, 9.500000000000000000 ) ) ;
#39336=EDGE_CURVE ( 'NONE', #22956, #34728, #24391, .T. ) ;
#39339=EDGE_LOOP ( 'NONE', ( #9851, #1036, #39850, #39709 ) ) ;
#39341=CIRCLE ( 'NONE', #4311, 0.5000000000000004441 ) ;
#39342=DIRECTION ( 'NONE',  ( 0.000000000000000000, 0.000000000000000000, 1.000000000000000000 ) ) ;
#39345=CARTESIAN_POINT ( 'NONE',  ( -5.524694096546769018, 36.45979188825334916, 10.49999999999999645 ) ) ;
#39347=EDGE_CURVE ( 'NONE', #38300, #20973, #15104, .T. ) ;
#39348=DIRECTION ( 'NONE',  ( -0.3090169943749573322, -0.9510565162951505336, 0.000000000000000000 ) ) ;
#39349=ADVANCED_FACE ( 'NONE', ( #12598 ), #21145, .T. ) ;
#39351=DIRECTION ( 'NONE',  ( 0.000000000000000000, -0.7071067811865451302, 0.7071067811865500152 ) ) ;
#39352=CARTESIAN_POINT ( 'NONE',  ( -2.525645716490710679, 8.212903943950959018, 7.000000000000000000 ) ) ;
#39353=DIRECTION ( 'NONE',  ( 1.000000000000000000, 0.000000000000000000, 0.000000000000000000 ) ) ;
#39355=DIRECTION ( 'NONE',  ( 0.1045284632676569680, 0.9945218953682730678, 0.000000000000000000 ) ) ;
#39356=VERTEX_POINT ( 'NONE', #18304 ) ;
#39358=CARTESIAN_POINT ( 'NONE',  ( -13.97557076678966403, 21.53386246193713305, 10.00000000000000000 ) ) ;
#39359=DIRECTION ( 'NONE',  ( -0.6459741880212467313, 0.2876062384759635604, 0.7071067811865462405 ) ) ;
#39361=PLANE ( 'NONE',  #33446 ) ;
#39364=CARTESIAN_POINT ( 'NONE',  ( 14.36830325120613772, 20.48707633493483371, 9.500000000000000000 ) ) ;
#39369=DIRECTION ( 'NONE',  ( 0.000000000000000000, 0.000000000000000000, 1.000000000000000000 ) ) ;
#39370=ORIENTED_EDGE ( 'NONE', *, *, #28199, .T. ) ;
#39372=ORIENTED_EDGE ( 'NONE', *, *, #5751, .T. ) ;
#39373=EDGE_CURVE ( 'NONE', #2857, #37653, #5900, .T. ) ;
#39374=VECTOR ( 'NONE', #21437, 1000.000000000000000 ) ;
#39377=ORIENTED_EDGE ( 'NONE', *, *, #37595, .F. ) ;
#39378=DIRECTION ( 'NONE',  ( -0.000000000000000000, -0.000000000000000000, -1.000000000000000000 ) ) ;
#39379=CARTESIAN_POINT ( 'NONE',  ( 2.672146553953312687, 12.33340603770390942, 10.00000000000000000 ) ) ;
#39384=DIRECTION ( 'NONE',  ( 0.4999999999999921174, -0.8660254037844431485, -0.000000000000000000 ) ) ;
#39385=ORIENTED_EDGE ( 'NONE', *, *, #13497, .T. ) ;
#39386=DIRECTION ( 'NONE',  ( -1.000000000000000000, 0.000000000000000000, 0.000000000000000000 ) ) ;
#39388=DIRECTION ( 'NONE',  ( -0.4446959099295410001, 0.6847716512521619947, 0.5773502691896187367 ) ) ;
#39389=ORIENTED_EDGE ( 'NONE', *, *, #11235, .T. ) ;
#39390=CARTESIAN_POINT ( 'NONE',  ( -5.644276917315534270, 36.40655018617698602, 10.49999999999999822 ) ) ;
#39391=LINE ( 'NONE', #17683, #7210 ) ;
#39393=EDGE_CURVE ( 'NONE', #38482, #27384, #10496, .T. ) ;
#39395=AXIS2_PLACEMENT_3D ( 'NONE', #29080, #850, #3891 ) ;
#39402=FACE_OUTER_BOUND ( 'NONE', #11491, .T. ) ;
#39403=AXIS2_PLACEMENT_3D ( 'NONE', #9854, #13493, #13088 ) ;
#39405=VECTOR ( 'NONE', #9272, 1000.000000000000000 ) ;
#39409=FACE_OUTER_BOUND ( 'NONE', #34414, .T. ) ;
#39410=ORIENTED_EDGE ( 'NONE', *, *, #15603, .T. ) ;
#39411=VERTEX_POINT ( 'NONE', #12396 ) ;
#39413=CYLINDRICAL_SURFACE ( 'NONE', #25634, 0.5000000000000004441 ) ;
#39414=ADVANCED_FACE ( 'NONE', ( #33552 ), #9356, .F. ) ;
#39415=CARTESIAN_POINT ( 'NONE',  ( -12.14063985594382800, 14.34296697341692095, 10.49999999999999822 ) ) ;
#39419=EDGE_CURVE ( 'NONE', #37722, #7787, #24785, .T. ) ;
#39420=CARTESIAN_POINT ( 'NONE',  ( 10.81260707898150386, 32.90853150812155548, 11.00000000000000000 ) ) ;
#39422=CARTESIAN_POINT ( 'NONE',  ( -2.629601561899593598, 7.723830143584060615, 10.49999999999999112 ) ) ;
#39425=CARTESIAN_POINT ( 'NONE',  ( -12.05736835487443237, 14.38397459621567442, 10.50000000000000000 ) ) ;
#39426=ORIENTED_EDGE ( 'NONE', *, *, #3200, .F. ) ;
#39429=AXIS2_PLACEMENT_3D ( 'NONE', #24682, #37078, #21436 ) ;
#39432=ORIENTED_EDGE ( 'NONE', *, *, #33257, .F. ) ;
#39440=EDGE_LOOP ( 'NONE', ( #11414, #4750, #10959 ) ) ;
#39441=DIRECTION ( 'NONE',  ( -0.7032331762534090869, 0.07391278520354985226, -0.7071067811865444641 ) ) ;
#39444=EDGE_CURVE ( 'NONE', #4676, #15434, #2465, .T. ) ;
#39449=DIRECTION ( 'NONE',  ( 0.9781476007338042455, -0.2079116908177663092, 0.000000000000000000 ) ) ;
#39451=DIRECTION ( 'NONE',  ( -0.9135454576426005335, 0.4067366430758008744, -0.000000000000000000 ) ) ;
#39455=ORIENTED_EDGE ( 'NONE', *, *, #38814, .T. ) ;
#39457=VECTOR ( 'NONE', #39074, 1000.000000000000000 ) ;
#39459=CARTESIAN_POINT ( 'NONE',  ( -3.938766756526925761, 8.166638875703812417, 10.49999999999999822 ) ) ;
#39463=ORIENTED_EDGE ( 'NONE', *, *, #39641, .F. ) ;
#39464=CIRCLE ( 'NONE', #552, 1.000000000000002665 ) ;
#39466=DIRECTION ( 'NONE',  ( 0.000000000000000000, 0.000000000000000000, 1.000000000000000000 ) ) ;
#39467=B_SPLINE_CURVE_WITH_KNOTS ( 'NONE', 3,
 ( #40087, #11867, #8619, #3315 ),
 .UNSPECIFIED., .F., .F.,
 ( 4, 4 ),
 ( 0.0006014480309583149914, 0.0009453384547274258469 ),
 .UNSPECIFIED. ) ;
#39469=ADVANCED_FACE ( 'NONE', ( #5699 ), #3405, .T. ) ;
#39470=CARTESIAN_POINT ( 'NONE',  ( -6.557822374958137246, 35.99981354310120452, 7.000000000000000000 ) ) ;
#39471=VECTOR ( 'NONE', #24387, 1000.000000000000114 ) ;
#39479=CARTESIAN_POINT ( 'NONE',  ( -8.317671217786068993, 10.20105690706398249, 10.87262190629279601 ) ) ;
#39480=CARTESIAN_POINT ( 'NONE',  ( 3.607749162633204332, 7.931741834401770497, 7.000000000000000000 ) ) ;
#39481=VERTEX_POINT ( 'NONE', #10353 ) ;
#39483=ORIENTED_EDGE ( 'NONE', *, *, #23415, .T. ) ;
#39489=LINE ( 'NONE', #26898, #10254 ) ;
#39492=DIRECTION ( 'NONE',  ( -0.000000000000000000, 0.000000000000000000, -1.000000000000000000 ) ) ;
#39495=CARTESIAN_POINT ( 'NONE',  ( 0.5000000000000035527, 32.50000000000000000, 10.50000000000000178 ) ) ;
#39496=ORIENTED_EDGE ( 'NONE', *, *, #17005, .F. ) ;
#39498=CARTESIAN_POINT ( 'NONE',  ( -13.63581098909220479, 27.45627467658446008, 7.499999999999993783 ) ) ;
#39501=ADVANCED_FACE ( 'NONE', ( #13392 ), #19287, .T. ) ;
#39502=DIRECTION ( 'NONE',  ( 1.000000000000000000, 0.000000000000000000, 0.000000000000000000 ) ) ;
#39505=ORIENTED_EDGE ( 'NONE', *, *, #30647, .F. ) ;
#39508=CARTESIAN_POINT ( 'NONE',  ( -13.94482798346716201, 26.50521816028930999, 7.000000000000000000 ) ) ;
#39510=ORIENTED_EDGE ( 'NONE', *, *, #9465, .F. ) ;
#39517=AXIS2_PLACEMENT_3D ( 'NONE', #11343, #27180, #39565 ) ;
#39518=VECTOR ( 'NONE', #18231, 999.9999999999998863 ) ;
#39521=DIRECTION ( 'NONE',  ( 0.9510565162951544194, 0.3090169943749449533, -0.000000000000000000 ) ) ;
#39523=ORIENTED_EDGE ( 'NONE', *, *, #27694, .T. ) ;
#39525=DIRECTION ( 'NONE',  ( -0.6123724356957955806, 0.3535533905932792820, -0.7071067811865437980 ) ) ;
#39527=DIRECTION ( 'NONE',  ( -0.000000000000000000, -0.000000000000000000, -1.000000000000000000 ) ) ;
#39528=AXIS2_PLACEMENT_3D ( 'NONE', #33518, #39388, #38993 ) ;
#39529=EDGE_LOOP ( 'NONE', ( #14481, #3892, #37823 ) ) ;
#39537=VERTEX_POINT ( 'NONE', #31682 ) ;
#39538=CARTESIAN_POINT ( 'NONE',  ( 14.98522546127354182, 21.83078073962648347, 7.382773698552468566 ) ) ;
#39541=FACE_OUTER_BOUND ( 'NONE', #35716, .T. ) ;
#39542=EDGE_LOOP ( 'NONE', ( #16043, #27425, #19873, #35736 ) ) ;
#39544=DIRECTION ( 'NONE',  ( 0.000000000000000000, 0.000000000000000000, 1.000000000000000000 ) ) ;
#39545=EDGE_CURVE ( 'NONE', #10050, #31776, #16250, .T. ) ;
#39546=CARTESIAN_POINT ( 'NONE',  ( -13.24038105676664401, 15.43301270189234486, 10.49999999999999822 ) ) ;
#39547=CARTESIAN_POINT ( 'NONE',  ( 21.39877161664088590, 15.54711762656346075, 7.000000000000000000 ) ) ;
#39548=CONICAL_SURFACE ( 'NONE', #19418, 0.9999999999999970024, 0.7853981633974552734 ) ;
#39550=DIRECTION ( 'NONE',  ( 1.000000000000000000, 0.000000000000000000, 0.000000000000000000 ) ) ;
#39551=CYLINDRICAL_SURFACE ( 'NONE', #8694, 0.4999999999999999445 ) ;
#39553=CARTESIAN_POINT ( 'NONE',  ( 9.581182426140127717, 10.95854901866634812, 7.339470489435492517 ) ) ;
#39554=VERTEX_POINT ( 'NONE', #37779 ) ;
#39556=LINE ( 'NONE', #30224, #25215 ) ;
#39557=EDGE_CURVE ( 'NONE', #29202, #13434, #34536, .T. ) ;
#39558=CARTESIAN_POINT ( 'NONE',  ( 13.24038105676654986, 15.43301270189216368, 10.49999999999999822 ) ) ;
#39560=EDGE_CURVE ( 'NONE', #27233, #10152, #7287, .T. ) ;
#39563=ORIENTED_EDGE ( 'NONE', *, *, #6413, .F. ) ;
#39565=DIRECTION ( 'NONE',  ( -1.000000000000000000, 0.000000000000000000, 0.000000000000000000 ) ) ;
#39571=B_SPLINE_CURVE_WITH_KNOTS ( 'NONE', 3,
 ( #21662, #34066, #18629, #3184 ),
 .UNSPECIFIED., .F., .F.,
 ( 4, 4 ),
 ( 0.000000000000000000, 1.000000000000000000 ),
 .UNSPECIFIED. ) ;
#39573=EDGE_LOOP ( 'NONE', ( #17007, #17364, #3058, #32162 ) ) ;
#39576=ORIENTED_EDGE ( 'NONE', *, *, #10569, .T. ) ;
#39577=FACE_OUTER_BOUND ( 'NONE', #6262, .T. ) ;
#39581=AXIS2_PLACEMENT_3D ( 'NONE', #26601, #23359, #17478 ) ;
#39584=ORIENTED_EDGE ( 'NONE', *, *, #32395, .T. ) ;
#39586=CARTESIAN_POINT ( 'NONE',  ( -4.984135866956331817, 36.15314577889358105, 7.500000000000000888 ) ) ;
#39587=ORIENTED_EDGE ( 'NONE', *, *, #32223, .F. ) ;
#39588=CARTESIAN_POINT ( 'NONE',  ( 13.37378135583786332, 20.59160479820249279, 10.00000000000000000 ) ) ;
#39592=ORIENTED_EDGE ( 'NONE', *, *, #33487, .T. ) ;
#39595=CARTESIAN_POINT ( 'NONE',  ( -13.30736835487442349, 15.68301270189233954, 7.499999999999993783 ) ) ;
#39601=ORIENTED_EDGE ( 'NONE', *, *, #37090, .F. ) ;
#39603=FACE_OUTER_BOUND ( 'NONE', #35409, .T. ) ;
#39607=CARTESIAN_POINT ( 'NONE',  ( 9.941034666242806850, 32.57396620494213124, 7.000000000000000000 ) ) ;
#39611=DIRECTION ( 'NONE',  ( 1.000000000000000000, 0.000000000000000000, 0.000000000000000000 ) ) ;
#39613=ORIENTED_EDGE ( 'NONE', *, *, #10914, .F. ) ;
#39616=DIRECTION ( 'NONE',  ( -0.6691306063588561281, 0.7431448254773961315, 0.000000000000000000 ) ) ;
#39617=AXIS2_PLACEMENT_3D ( 'NONE', #19859, #17016, #26349 ) ;
#39618=FACE_OUTER_BOUND ( 'NONE', #12844, .T. ) ;
#39619=ORIENTED_EDGE ( 'NONE', *, *, #18736, .T. ) ;
#39621=VECTOR ( 'NONE', #21851, 1000.000000000000000 ) ;
#39622=CARTESIAN_POINT ( 'NONE',  ( -14.47283171447380035, 21.48159823030330884, 7.000000000000000000 ) ) ;
#39623=CARTESIAN_POINT ( 'NONE',  ( -2.629601561899621576, 7.723830143584065056, 10.59344459855561382 ) ) ;
#39624=EDGE_CURVE ( 'NONE', #490, #13732, #11295, .T. ) ;
#39625=ORIENTED_EDGE ( 'NONE', *, *, #32797, .F. ) ;
#39631=EDGE_LOOP ( 'NONE', ( #27621, #5838, #27639, #34896, #6560 ) ) ;
#39635=DIRECTION ( 'NONE',  ( 0.9135454576426048634, 0.4067366430757912710, 0.000000000000000000 ) ) ;
#39638=ORIENTED_EDGE ( 'NONE', *, *, #24693, .F. ) ;
#39641=EDGE_CURVE ( 'NONE', #23735, #6691, #37139, .T. ) ;
#39644=CARTESIAN_POINT ( 'NONE',  ( -9.754330675317843813, 26.45797082815842316, 10.74999999999999645 ) ) ;
#39645=ADVANCED_FACE ( 'NONE', ( #29773 ), #8638, .T. ) ;
#39647=AXIS2_PLACEMENT_3D ( 'NONE', #4514, #29497, #10814 ) ;
#39650=LINE ( 'NONE', #15469, #30028 ) ;
#39651=DIRECTION ( 'NONE',  ( 0.000000000000000000, 0.000000000000000000, 1.000000000000000000 ) ) ;
#39652=ORIENTED_EDGE ( 'NONE', *, *, #37086, .F. ) ;
#39656=ADVANCED_FACE ( 'NONE', ( #1749 ), #24275, .T. ) ;
#39661=ORIENTED_EDGE ( 'NONE', *, *, #36084, .T. ) ;
#39665=CARTESIAN_POINT ( 'NONE',  ( 13.67979938750375979, 27.47056737363388734, 10.99999999999999289 ) ) ;
#39672=VERTEX_POINT ( 'NONE', #30175 ) ;
#39675=PLANE ( 'NONE',  #8928 ) ;
#39676=ADVANCED_FACE ( 'NONE', ( #20640 ), #28166, .T. ) ;
#39677=ORIENTED_EDGE ( 'NONE', *, *, #4066, .T. ) ;
#39678=EDGE_CURVE ( 'NONE', #19098, #855, #35191, .T. ) ;
#39683=AXIS2_PLACEMENT_3D ( 'NONE', #30058, #29851, #24560 ) ;
#39685=AXIS2_PLACEMENT_3D ( 'NONE', #34100, #6454, #16008 ) ;
#39688=CARTESIAN_POINT ( 'NONE',  ( -10.33756681542519118, 33.36973668161310513, 7.202682876670055911 ) ) ;
#39691=LINE ( 'NONE', #37045, #32503 ) ;
#39693=CARTESIAN_POINT ( 'NONE',  ( 8.118377661053324701, 10.47536095541698486, 9.500000000000000000 ) ) ;
#39694=ADVANCED_FACE ( 'NONE', ( #12871 ), #18188, .F. ) ;
#39695=DIRECTION ( 'NONE',  ( -0.5877852522924797984, -0.8090169943749425663, 0.000000000000000000 ) ) ;
#39698=DIRECTION ( 'NONE',  ( 0.1045284632676559550, 0.9945218953682730678, 0.000000000000000000 ) ) ;
#39701=DIRECTION ( 'NONE',  ( -0.000000000000000000, -0.000000000000000000, -1.000000000000000000 ) ) ;
#39704=ORIENTED_EDGE ( 'NONE', *, *, #8912, .T. ) ;
#39709=ORIENTED_EDGE ( 'NONE', *, *, #352, .T. ) ;
#39714=B_SPLINE_CURVE_WITH_KNOTS ( 'NONE', 3,
 ( #2297, #38864, #36227, #4734 ),
 .UNSPECIFIED., .F., .F.,
 ( 4, 4 ),
 ( 0.000000000000000000, 1.000000000000000000 ),
 .UNSPECIFIED. ) ;
#39719=DIRECTION ( 'NONE',  ( 0.3090169943749465631, -0.9510565162951538642, 0.000000000000000000 ) ) ;
#39721=ORIENTED_EDGE ( 'NONE', *, *, #33018, .F. ) ;
#39724=TOROIDAL_SURFACE ( 'NONE', #15703, 1.000000000000000000, 0.5000000000000000000 ) ;
#39725=CYLINDRICAL_SURFACE ( 'NONE', #12113, 0.5000000000000005551 ) ;
#39726=FACE_OUTER_BOUND ( 'NONE', #26111, .T. ) ;
#39727=ORIENTED_EDGE ( 'NONE', *, *, #26182, .F. ) ;
#39731=DIRECTION ( 'NONE',  ( 0.9781476007338069101, 0.2079116908177532363, 0.000000000000000000 ) ) ;
#39737=CARTESIAN_POINT ( 'NONE',  ( 10.10646936306337729, 32.94553861768082470, 7.499999999999997335 ) ) ;
#39738=DIRECTION ( 'NONE',  ( 0.4067366430757995976, 0.9135454576426010886, 0.000000000000000000 ) ) ;
#39743=AXIS2_PLACEMENT_3D ( 'NONE', #30498, #34343, #36784 ) ;
#39744=LINE ( 'NONE', #11922, #10989 ) ;
#39745=DIRECTION ( 'NONE',  ( 1.000000000000000000, 0.000000000000000000, 0.000000000000000000 ) ) ;
#39749=CARTESIAN_POINT ( 'NONE',  ( -13.37378135583788286, 20.59160479820268108, 10.50000000000000000 ) ) ;
#39750=ORIENTED_EDGE ( 'NONE', *, *, #39173, .F. ) ;
#39754=LINE ( 'NONE', #36720, #22428 ) ;
#39767=DIRECTION ( 'NONE',  ( -0.9135454576426005335, 0.4067366430758010964, 0.000000000000000000 ) ) ;
#39769=ORIENTED_EDGE ( 'NONE', *, *, #40153, .F. ) ;
#39771=AXIS2_PLACEMENT_3D ( 'NONE', #33529, #23764, #8730 ) ;
#39776=CONICAL_SURFACE ( 'NONE', #24202, 0.5000000000000046629, 0.7853981633974492782 ) ;
#39777=DIRECTION ( 'NONE',  ( 1.000000000000000000, 0.000000000000000000, 0.000000000000000000 ) ) ;
#39780=VECTOR ( 'NONE', #7905, 1000.000000000000000 ) ;
#39781=ADVANCED_FACE ( 'NONE', ( #6372 ), #27914, .F. ) ;
#39782=EDGE_LOOP ( 'NONE', ( #8987, #22733, #6814, #7625 ) ) ;
#39784=ORIENTED_EDGE ( 'NONE', *, *, #9937, .T. ) ;
#39787=DIRECTION ( 'NONE',  ( -0.000000000000000000, -0.000000000000000000, -1.000000000000000000 ) ) ;
#39788=CARTESIAN_POINT ( 'NONE',  ( -3.820972158149174458, 8.017991022712379845, 10.49999999999999822 ) ) ;
#39789=VERTEX_POINT ( 'NONE', #15531 ) ;
#39791=CYLINDRICAL_SURFACE ( 'NONE', #24992, 0.5000000000000004441 ) ;
#39793=DIRECTION ( 'NONE',  ( -0.1045284632676569680, -0.9945218953682730678, 0.000000000000000000 ) ) ;
#39799=FACE_OUTER_BOUND ( 'NONE', #9610, .T. ) ;
#39804=DIRECTION ( 'NONE',  ( 1.000000000000000000, 0.000000000000000000, 0.000000000000000000 ) ) ;
#39805=CARTESIAN_POINT ( 'NONE',  ( -13.48130249190472796, 27.93180293473203335, 9.500000000000000000 ) ) ;
#39809=CARTESIAN_POINT ( 'NONE',  ( 11.61617248865833396, 31.85261603038683376, 10.49999999999999822 ) ) ;
#39810=VERTEX_POINT ( 'NONE', #6179 ) ;
#39813=CARTESIAN_POINT ( 'NONE',  ( 0.8223886111234900431, 37.39061994947682877, 10.49999999999999822 ) ) ;
#39819=DIRECTION ( 'NONE',  ( -0.000000000000000000, -0.000000000000000000, 1.000000000000000000 ) ) ;
#39823=EDGE_CURVE ( 'NONE', #19575, #15240, #22886, .T. ) ;
#39824=CARTESIAN_POINT ( 'NONE',  ( -13.47830981910552772, 21.58612669357095015, 10.00000000000000000 ) ) ;
#39825=ORIENTED_EDGE ( 'NONE', *, *, #26410, .F. ) ;
#39835=ORIENTED_EDGE ( 'NONE', *, *, #9616, .F. ) ;
#39840=VECTOR ( 'NONE', #8169, 1000.000000000000000 ) ;
#39842=EDGE_CURVE ( 'NONE', #30884, #39356, #18384, .T. ) ;
#39846=FACE_OUTER_BOUND ( 'NONE', #25368, .T. ) ;
#39848=VERTEX_POINT ( 'NONE', #27519 ) ;
#39850=ORIENTED_EDGE ( 'NONE', *, *, #11486, .F. ) ;
#39858=CARTESIAN_POINT ( 'NONE',  ( 13.84312823610354748, 27.91543399189757579, 10.49999999999999822 ) ) ;
#39860=CARTESIAN_POINT ( 'NONE',  ( 14.78469161520106034, 20.18088120075953640, 10.49999999999999822 ) ) ;
#39866=ORIENTED_EDGE ( 'NONE', *, *, #33431, .F. ) ;
#39868=FACE_OUTER_BOUND ( 'NONE', #18582, .T. ) ;
#39870=ORIENTED_EDGE ( 'NONE', *, *, #2420, .T. ) ;
#39872=ADVANCED_FACE ( 'NONE', ( #9828 ), #39776, .T. ) ;
#39876=ORIENTED_EDGE ( 'NONE', *, *, #17259, .T. ) ;
#39878=CARTESIAN_POINT ( 'NONE',  ( -10.67421745135738043, 33.03884568954855183, 7.485699520496981840 ) ) ;
#39879=AXIS2_PLACEMENT_3D ( 'NONE', #3233, #21517, #24368 ) ;
#39880=DIRECTION ( 'NONE',  ( 0.4999999999999920064, -0.8660254037844432595, 0.000000000000000000 ) ) ;
#39882=CARTESIAN_POINT ( 'NONE',  ( -1.204925152852743375, 12.02153850147729308, 10.50000000000000355 ) ) ;
#39883=AXIS2_PLACEMENT_3D ( 'NONE', #17840, #9276, #34063 ) ;
#39884=CIRCLE ( 'NONE', #20457, 1.000000000000002665 ) ;
#39886=LINE ( 'NONE', #17783, #37983 ) ;
#39889=CARTESIAN_POINT ( 'NONE',  ( 1.400691654708310141, 37.43445890845833901, 7.000000000000000000 ) ) ;
#39892=EDGE_CURVE ( 'NONE', #32345, #14313, #18973, .T. ) ;
#39893=LINE ( 'NONE', #14924, #9897 ) ;
#39897=ORIENTED_EDGE ( 'NONE', *, *, #24010, .T. ) ;
#39900=CARTESIAN_POINT ( 'NONE',  ( 2.525645716490518833, 8.212903943950921715, 7.000000000000000000 ) ) ;
#39902=EDGE_LOOP ( 'NONE', ( #19840, #21987, #2812, #26232 ) ) ;
#39903=DIRECTION ( 'NONE',  ( -0.5877852522924797984, -0.8090169943749425663, 0.000000000000000000 ) ) ;
#39906=DIRECTION ( 'NONE',  ( 1.000000000000000000, 0.000000000000000000, 0.000000000000000000 ) ) ;
#39912=CARTESIAN_POINT ( 'NONE',  ( -11.85099884957084626, 31.69690594862152722, 7.259166423030696258 ) ) ;
#39917=CARTESIAN_POINT ( 'NONE',  ( -12.80736835487442349, 15.68301270189233954, 7.499999999999993783 ) ) ;
#39918=DIRECTION ( 'NONE',  ( 0.000000000000000000, 0.000000000000000000, 1.000000000000000000 ) ) ;
#39924=AXIS2_PLACEMENT_3D ( 'NONE', #39495, #11274, #5171 ) ;
#39925=VECTOR ( 'NONE', #39267, 1000.000000000000000 ) ;
#39926=CARTESIAN_POINT ( 'NONE',  ( 0.000000000000000000, 22.50000000000000355, 7.000000000000000000 ) ) ;
#39932=ORIENTED_EDGE ( 'NONE', *, *, #5943, .T. ) ;
#39933=PLANE ( 'NONE',  #2237 ) ;
#39935=LINE ( 'NONE', #33667, #35238 ) ;
#39937=CARTESIAN_POINT ( 'NONE',  ( -5.037377569032697622, 36.27272859966233653, 10.49999999999999822 ) ) ;
#39938=DIRECTION ( 'NONE',  ( -0.4156269377774379215, 0.5720614028176924659, -0.7071067811865500152 ) ) ;
#39943=DIRECTION ( 'NONE',  ( 1.000000000000000000, 0.000000000000000000, 0.000000000000000000 ) ) ;
#39947=CARTESIAN_POINT ( 'NONE',  ( -14.09933648065464062, 26.02968990214173317, 7.000000000000000000 ) ) ;
#39948=ORIENTED_EDGE ( 'NONE', *, *, #31146, .F. ) ;
#39951=AXIS2_PLACEMENT_3D ( 'NONE', #36168, #11387, #2638 ) ;
#39952=CARTESIAN_POINT ( 'NONE',  ( -6.282361020112263716, 14.70372268239681190, 10.50000000000000533 ) ) ;
#39953=VECTOR ( 'NONE', #336, 1000.000000000000000 ) ;
#39958=VERTEX_POINT ( 'NONE', #13266 ) ;
#39959=CARTESIAN_POINT ( 'NONE',  ( -4.003810537522578983, 8.420815593655365916, 10.49999999999999822 ) ) ;
#39960=DIRECTION ( 'NONE',  ( -0.8660254037844364872, 0.5000000000000038858, 0.000000000000000000 ) ) ;
#39966=CARTESIAN_POINT ( 'NONE',  ( 13.05736835487433289, 16.11602540378438420, 10.50000000000000178 ) ) ;
#39970=ADVANCED_FACE ( 'NONE', ( #25859 ), #22406, .T. ) ;
#39974=CARTESIAN_POINT ( 'NONE',  ( -14.97009266215794021, 21.42933399866948463, 7.000000000000000000 ) ) ;
#39980=VERTEX_POINT ( 'NONE', #13469 ) ;
#39981=LINE ( 'NONE', #9313, #40094 ) ;
#39982=ORIENTED_EDGE ( 'NONE', *, *, #27318, .T. ) ;
#39983=DIRECTION ( 'NONE',  ( 0.000000000000000000, 0.000000000000000000, 1.000000000000000000 ) ) ;
#39984=FACE_OUTER_BOUND ( 'NONE', #17547, .T. ) ;
#39985=DIRECTION ( 'NONE',  ( 0.000000000000000000, 0.000000000000000000, -1.000000000000000000 ) ) ;
#39986=ORIENTED_EDGE ( 'NONE', *, *, #23558, .T. ) ;
#39988=DIRECTION ( 'NONE',  ( 0.000000000000000000, 0.000000000000000000, -1.000000000000000000 ) ) ;
#39989=CARTESIAN_POINT ( 'NONE',  ( 6.576253646258389374, 14.29921418520925869, 10.00000000000000000 ) ) ;
#39990=DIRECTION ( 'NONE',  ( 0.8660254037844364872, -0.5000000000000038858, 0.000000000000000000 ) ) ;
#39999=EDGE_CURVE ( 'NONE', #8131, #10797, #13062, .T. ) ;
#40006=CARTESIAN_POINT ( 'NONE',  ( 19.15807744002891155, 8.842452143891316396, 7.000000000000000000 ) ) ;
#40008=ORIENTED_EDGE ( 'NONE', *, *, #34226, .F. ) ;
#40010=CARTESIAN_POINT ( 'NONE',  ( 0.6308996938995748982, 37.50000000000000711, 10.49999999999999645 ) ) ;
#40012=CARTESIAN_POINT ( 'NONE',  ( -9.067459072332603398, 10.87036407658132120, 10.94387467463491070 ) ) ;
#40013=ORIENTED_EDGE ( 'NONE', *, *, #22230, .T. ) ;
#40017=EDGE_LOOP ( 'NONE', ( #6830, #14618, #29528, #28589 ) ) ;
#40019=DIRECTION ( 'NONE',  ( -0.000000000000000000, -0.000000000000000000, -1.000000000000000000 ) ) ;
#40020=ORIENTED_EDGE ( 'NONE', *, *, #12360, .T. ) ;
#40024=EDGE_CURVE ( 'NONE', #27921, #26306, #30041, .T. ) ;
#40029=AXIS2_PLACEMENT_3D ( 'NONE', #354, #34082, #37724 ) ;
#40033=LINE ( 'NONE', #8768, #21711 ) ;
#40034=DIRECTION ( 'NONE',  ( 0.000000000000000000, 0.000000000000000000, 1.000000000000000000 ) ) ;
#40035=AXIS2_PLACEMENT_3D ( 'NONE', #35491, #16197, #22880 ) ;
#40037=VECTOR ( 'NONE', #39145, 1000.000000000000000 ) ;
#40039=CARTESIAN_POINT ( 'NONE',  ( 2.063787492809801893, 7.980908877017387937, 10.49999999999999467 ) ) ;
#40041=B_SPLINE_CURVE_WITH_KNOTS ( 'NONE', 3,
 ( #2129, #17974, #9021, #2332, #33813, #1934, #3120, #13049 ),
 .UNSPECIFIED., .F., .F.,
 ( 4, 2, 2, 4 ),
 ( 0.000000000000000000, 0.0002364868538934332008, 0.0004729737077868664016, 0.0009459474155737283580 ),
 .UNSPECIFIED. ) ;
#40043=CARTESIAN_POINT ( 'NONE',  ( -2.568190708544555001, 12.82247983807085134, 10.50000000000000533 ) ) ;
#40050=ADVANCED_FACE ( 'NONE', ( #10634 ), #34808, .F. ) ;
#40057=CARTESIAN_POINT ( 'NONE',  ( -6.354454053420243831, 35.54304081427989814, 7.500000000000000888 ) ) ;
#40058=AXIS2_PLACEMENT_3D ( 'NONE', #21536, #18498, #15442 ) ;
#40060=ORIENTED_EDGE ( 'NONE', *, *, #34928, .F. ) ;
#40066=DIRECTION ( 'NONE',  ( 0.000000000000000000, 0.000000000000000000, 1.000000000000000000 ) ) ;
#40067=DIRECTION ( 'NONE',  ( -1.000000000000000000, 0.000000000000000000, 0.000000000000000000 ) ) ;
#40068=VECTOR ( 'NONE', #6206, 999.9999999999998863 ) ;
#40076=ADVANCED_FACE ( 'NONE', ( #19165 ), #35210, .T. ) ;
#40079=ADVANCED_FACE ( 'NONE', ( #31764 ), #4125, .F. ) ;
#40083=LINE ( 'NONE', #9215, #26627 ) ;
#40084=CIRCLE ( 'NONE', #22564, 0.9999999999999996669 ) ;
#40086=AXIS2_PLACEMENT_3D ( 'NONE', #9001, #40066, #12438 ) ;
#40087=CARTESIAN_POINT ( 'NONE',  ( -11.74460609746112461, 31.83082137946488643, 7.365559175140416137 ) ) ;
#40089=ORIENTED_EDGE ( 'NONE', *, *, #27301, .F. ) ;
#40092=DIRECTION ( 'NONE',  ( -1.000000000000000000, 0.000000000000000000, 0.000000000000000000 ) ) ;
#40094=VECTOR ( 'NONE', #368, 1000.000000000000000 ) ;
#40096=ADVANCED_FACE ( 'NONE', ( #3663 ), #12806, .F. ) ;
#40098=ORIENTED_EDGE ( 'NONE', *, *, #26662, .F. ) ;
#40103=ORIENTED_EDGE ( 'NONE', *, *, #19189, .F. ) ;
#40104=DIRECTION ( 'NONE',  ( 0.8090169943749503378, 0.5877852522924691403, 0.000000000000000000 ) ) ;
#40105=VERTEX_POINT ( 'NONE', #22147 ) ;
#40107=CARTESIAN_POINT ( 'NONE',  ( -13.13581098909220479, 27.45627467658446008, 9.500000000000000000 ) ) ;
#40114=ORIENTED_EDGE ( 'NONE', *, *, #17365, .F. ) ;
#40119=ORIENTED_EDGE ( 'NONE', *, *, #10356, .T. ) ;
#40124=DIRECTION ( 'NONE',  ( 0.4067366430757984874, 0.9135454576426016438, -2.428612866367517941E-14 ) ) ;
#40126=ORIENTED_EDGE ( 'NONE', *, *, #16587, .F. ) ;
#40128=CIRCLE ( 'NONE', #31060, 0.5000000000000004441 ) ;
#40130=ADVANCED_FACE ( 'NONE', ( #226 ), #32082, .T. ) ;
#40133=ORIENTED_EDGE ( 'NONE', *, *, #10356, .F. ) ;
#40134=CARTESIAN_POINT ( 'NONE',  ( 3.914034194965609892, 30.06176806842420035, 9.000000000000001776 ) ) ;
#40135=B_SPLINE_CURVE_WITH_KNOTS ( 'NONE', 3,
 ( #28922, #19375, #31568, #32388 ),
 .UNSPECIFIED., .F., .F.,
 ( 4, 4 ),
 ( 0.000000000000000000, 1.000000000000000000 ),
 .UNSPECIFIED. ) ;
#40139=CARTESIAN_POINT ( 'NONE',  ( -13.63581098909220302, 27.45627467658446719, 11.00000000000000000 ) ) ;
#40140=DIRECTION ( 'NONE',  ( -0.000000000000000000, -0.000000000000000000, -1.000000000000000000 ) ) ;
#40143=CARTESIAN_POINT ( 'NONE',  ( 11.64304932069170029, 31.95750204166777309, 7.455539900862796721 ) ) ;
#40145=CARTESIAN_POINT ( 'NONE',  ( 14.33090402811217068, 26.16159042914056698, 10.49999999999999467 ) ) ;
#40151=CARTESIAN_POINT ( 'NONE',  ( -6.282361020112263716, 14.70372268239681190, 10.50000000000000533 ) ) ;
#40153=EDGE_CURVE ( 'NONE', #10907, #33136, #18514, .T. ) ;
#40158=AXIS2_PLACEMENT_3D ( 'NONE', #12852, #6157, #37441 ) ;
#40160=CARTESIAN_POINT ( 'NONE',  ( 7.126083911573380725, 10.99048532364570008, 10.50000000000000000 ) ) ;
#40163=EDGE_CURVE ( 'NONE', #24240, #26220, #12513, .T. ) ;
#40170=ORIENTED_EDGE ( 'NONE', *, *, #38050, .T. ) ;
#40176=EDGE_CURVE ( 'NONE', #18778, #163, #34353, .T. ) ;
#40178=EDGE_CURVE ( 'NONE', #31871, #2935, #17083, .T. ) ;
#40183=ORIENTED_EDGE ( 'NONE', *, *, #29005, .T. ) ;
#40185=FACE_OUTER_BOUND ( 'NONE', #39440, .T. ) ;
#40186=CARTESIAN_POINT ( 'NONE',  ( -11.11016527260153630, 31.83082137946488643, 7.500000000000004441 ) ) ;
#40188=VERTEX_POINT ( 'NONE', #18907 ) ;
#40191=LINE ( 'NONE', #12364, #21520 ) ;
#40194=EDGE_CURVE ( 'NONE', #31812, #34769, #24605, .T. ) ;
#40197=VERTEX_POINT ( 'NONE', #27648 ) ;
ENDSEC;
END-ISO-10303-21;
